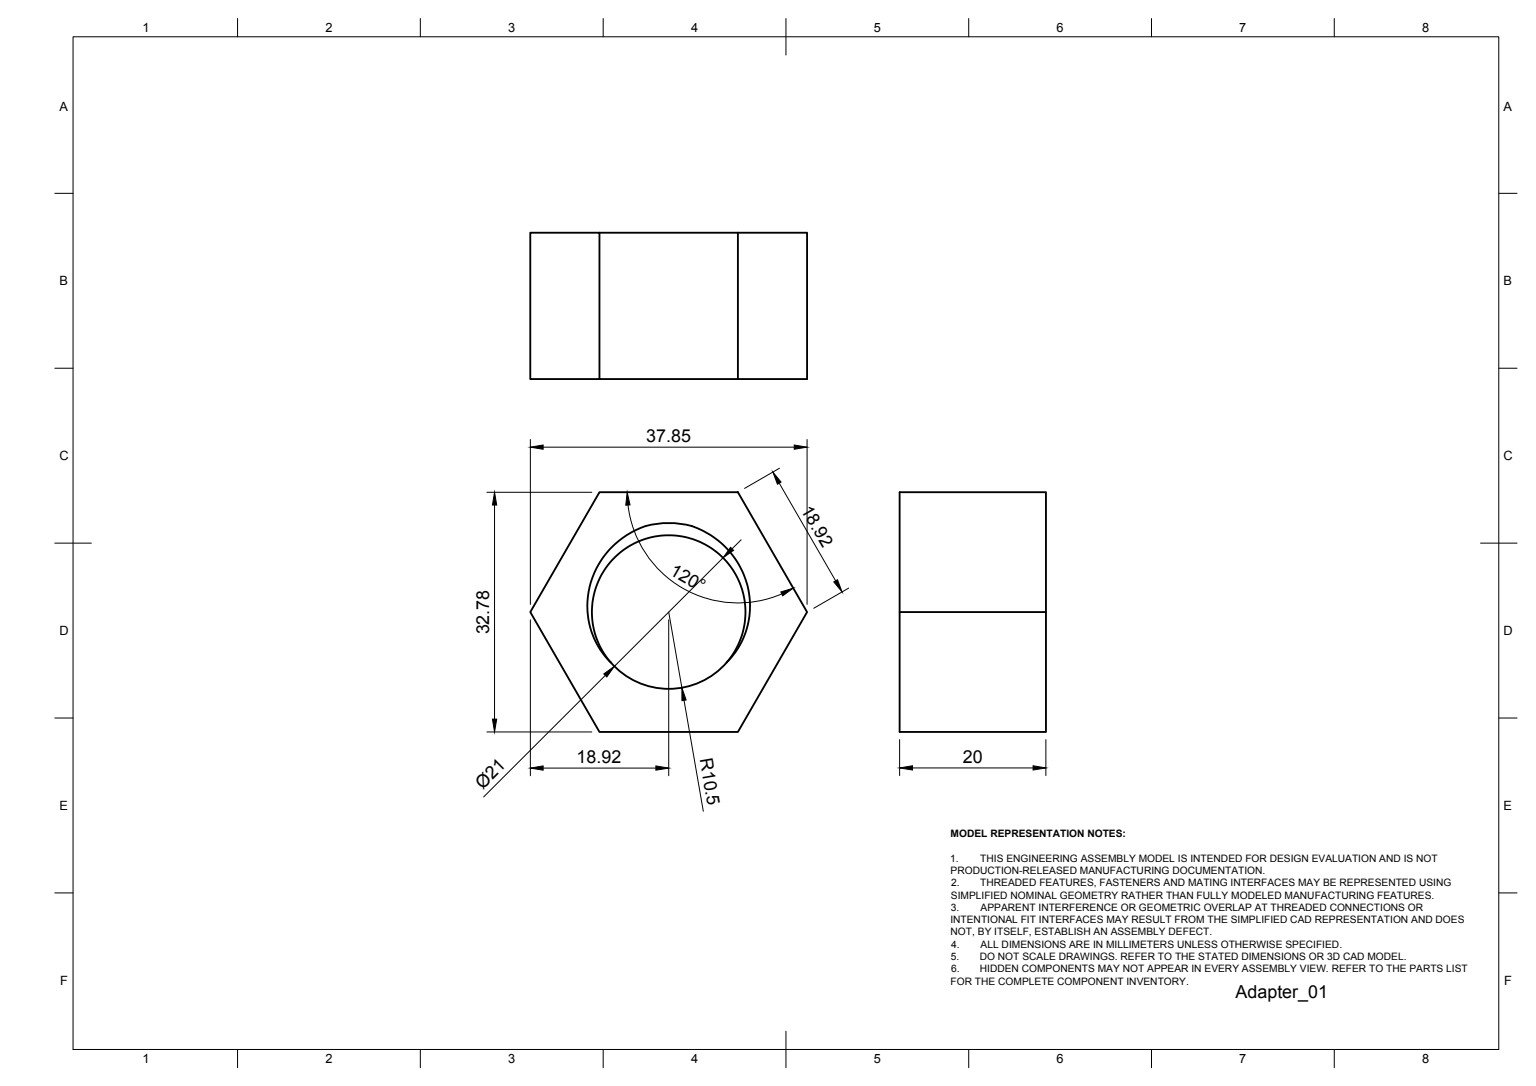
ISO-10303-21;
HEADER;
/* Generated by software containing ST-Developer
 * from STEP Tools, Inc. (www.steptools.com) 
 */

FILE_DESCRIPTION(
/* description */ (''),
/* implementation_level */ '2;1');

FILE_NAME(
/* name */ 'Adapter_01.step',
/* time_stamp */ '2026-10-06T12:47:13-07:00',
/* author */ (''),
/* organization */ (''),
/* preprocessor_version */ 'ST-DEVELOPER v20.2',
/* originating_system */ 'Autodesk Translation Framework v15.15.0.0',
/* authorisation */ '');

FILE_SCHEMA (('AUTOMOTIVE_DESIGN { 1 0 10303 214 3 1 1 }'));
ENDSEC;

DATA;
#10=MECHANICAL_DESIGN_GEOMETRIC_PRESENTATION_REPRESENTATION('',(#75),#42667);
#57=SHAPE_REPRESENTATION_RELATIONSHIP('SRR','None',#42710,#66);
#66=ADVANCED_BREP_SHAPE_REPRESENTATION('',(#84),#42666);
#75=STYLED_ITEM('',(#42756),#84);
#84=MANIFOLD_SOLID_BREP('Body1',#4040);
#92=B_SPLINE_SURFACE_WITH_KNOTS('',3,3,((#41391,#41392,#41393,#41394,#41395,
#41396,#41397,#41398,#41399,#41400,#41401,#41402,#41403,#41404,#41405,#41406,
#41407,#41408,#41409,#41410,#41411,#41412,#41413,#41414,#41415,#41416,#41417,
#41418,#41419,#41420,#41421,#41422,#41423,#41424,#41425,#41426,#41427,#41428,
#41429,#41430,#41431,#41432,#41433,#41434,#41435,#41436,#41437,#41438,#41439,
#41440,#41441,#41442,#41443,#41444,#41445,#41446,#41447,#41448,#41449,#41450,
#41451,#41452,#41453,#41454,#41455,#41456,#41457,#41458,#41459,#41460,#41461,
#41462,#41463,#41464,#41465,#41466,#41467,#41468,#41469,#41470,#41471,#41472,
#41473,#41474,#41475,#41476,#41477,#41478,#41479,#41480,#41481),(#41482,
#41483,#41484,#41485,#41486,#41487,#41488,#41489,#41490,#41491,#41492,#41493,
#41494,#41495,#41496,#41497,#41498,#41499,#41500,#41501,#41502,#41503,#41504,
#41505,#41506,#41507,#41508,#41509,#41510,#41511,#41512,#41513,#41514,#41515,
#41516,#41517,#41518,#41519,#41520,#41521,#41522,#41523,#41524,#41525,#41526,
#41527,#41528,#41529,#41530,#41531,#41532,#41533,#41534,#41535,#41536,#41537,
#41538,#41539,#41540,#41541,#41542,#41543,#41544,#41545,#41546,#41547,#41548,
#41549,#41550,#41551,#41552,#41553,#41554,#41555,#41556,#41557,#41558,#41559,
#41560,#41561,#41562,#41563,#41564,#41565,#41566,#41567,#41568,#41569,#41570,
#41571,#41572),(#41573,#41574,#41575,#41576,#41577,#41578,#41579,#41580,
#41581,#41582,#41583,#41584,#41585,#41586,#41587,#41588,#41589,#41590,#41591,
#41592,#41593,#41594,#41595,#41596,#41597,#41598,#41599,#41600,#41601,#41602,
#41603,#41604,#41605,#41606,#41607,#41608,#41609,#41610,#41611,#41612,#41613,
#41614,#41615,#41616,#41617,#41618,#41619,#41620,#41621,#41622,#41623,#41624,
#41625,#41626,#41627,#41628,#41629,#41630,#41631,#41632,#41633,#41634,#41635,
#41636,#41637,#41638,#41639,#41640,#41641,#41642,#41643,#41644,#41645,#41646,
#41647,#41648,#41649,#41650,#41651,#41652,#41653,#41654,#41655,#41656,#41657,
#41658,#41659,#41660,#41661,#41662,#41663),(#41664,#41665,#41666,#41667,
#41668,#41669,#41670,#41671,#41672,#41673,#41674,#41675,#41676,#41677,#41678,
#41679,#41680,#41681,#41682,#41683,#41684,#41685,#41686,#41687,#41688,#41689,
#41690,#41691,#41692,#41693,#41694,#41695,#41696,#41697,#41698,#41699,#41700,
#41701,#41702,#41703,#41704,#41705,#41706,#41707,#41708,#41709,#41710,#41711,
#41712,#41713,#41714,#41715,#41716,#41717,#41718,#41719,#41720,#41721,#41722,
#41723,#41724,#41725,#41726,#41727,#41728,#41729,#41730,#41731,#41732,#41733,
#41734,#41735,#41736,#41737,#41738,#41739,#41740,#41741,#41742,#41743,#41744,
#41745,#41746,#41747,#41748,#41749,#41750,#41751,#41752,#41753,#41754)),
 .UNSPECIFIED.,.F.,.F.,.F.,(4,4),(4,1,1,1,1,1,1,1,1,1,1,1,1,1,1,1,1,1,1,
1,1,1,1,1,1,1,1,1,1,1,1,1,1,1,1,1,1,1,1,1,1,1,1,1,1,1,1,1,1,1,1,1,1,1,1,
1,1,1,1,1,1,1,1,1,1,1,1,1,1,1,1,1,1,1,1,1,1,1,1,1,1,1,1,1,1,1,1,1,4),(-0.000129081019394558,
0.193330292353948),(11.8519068837255,12.3510302549558,12.8500245451668,
13.3490188353777,13.8480131255886,14.3470074157995,14.8460017060104,15.3449959962214,
15.8439902864323,16.3429845766432,16.8419788668541,17.3409731570651,17.839967447276,
18.3389617374869,18.8379560276978,19.3369503179088,19.8359446081197,20.3349388983306,
20.8339331885415,21.3329274787524,21.8319217689634,22.3309160591743,22.8299103493852,
23.3289046395961,23.8278989298071,24.326893220018,24.8258875102289,25.3248818004398,
25.8238760906508,26.3228703808617,26.8218646710726,27.3208589612835,27.8198532514944,
28.3188475417054,28.8178418319163,29.3168361221272,29.8158304123381,30.3148247025491,
30.81381899276,31.3128132829709,31.8118075731818,32.3108018633928,32.8097961536037,
33.3087904438146,33.8077847340255,34.3067790242364,34.8057733144474,35.3047676046583,
35.8037618948692,36.3027561850801,36.8017504752911,37.300744765502,37.7997390557129,
38.2987333459238,38.7977276361348,39.2967219263457,39.7957162165566,40.2947105067675,
40.7937047969784,41.2926990871894,41.7916933774003,42.2906876676112,42.7896819578221,
43.2886762480331,43.787670538244,44.2866648284549,44.7856591186658,45.2846534088767,
45.7836476990877,46.2826419892986,46.7816362795095,47.2806305697204,47.7796248599314,
48.2786191501423,48.7776134403532,49.2766077305641,49.7756020207751,50.274596310986,
50.7735906011969,51.2725848914078,51.7715791816187,52.2705734718297,52.7695677620406,
53.2685620522515,53.7675563424624,54.2665506326734,54.7655449228843,55.2645392130952,
55.7635335033061),.UNSPECIFIED.);
#93=B_SPLINE_SURFACE_WITH_KNOTS('',3,3,((#41996,#41997,#41998,#41999,#42000,
#42001,#42002,#42003,#42004,#42005,#42006,#42007,#42008,#42009,#42010,#42011,
#42012,#42013,#42014,#42015,#42016,#42017,#42018,#42019,#42020,#42021,#42022,
#42023,#42024,#42025,#42026,#42027,#42028,#42029,#42030,#42031,#42032,#42033,
#42034,#42035,#42036,#42037,#42038,#42039,#42040,#42041,#42042,#42043,#42044,
#42045,#42046,#42047,#42048,#42049,#42050,#42051,#42052,#42053,#42054,#42055,
#42056,#42057,#42058,#42059,#42060,#42061,#42062,#42063,#42064,#42065,#42066,
#42067,#42068,#42069,#42070,#42071,#42072,#42073,#42074,#42075,#42076,#42077,
#42078,#42079,#42080,#42081,#42082,#42083,#42084,#42085,#42086),(#42087,
#42088,#42089,#42090,#42091,#42092,#42093,#42094,#42095,#42096,#42097,#42098,
#42099,#42100,#42101,#42102,#42103,#42104,#42105,#42106,#42107,#42108,#42109,
#42110,#42111,#42112,#42113,#42114,#42115,#42116,#42117,#42118,#42119,#42120,
#42121,#42122,#42123,#42124,#42125,#42126,#42127,#42128,#42129,#42130,#42131,
#42132,#42133,#42134,#42135,#42136,#42137,#42138,#42139,#42140,#42141,#42142,
#42143,#42144,#42145,#42146,#42147,#42148,#42149,#42150,#42151,#42152,#42153,
#42154,#42155,#42156,#42157,#42158,#42159,#42160,#42161,#42162,#42163,#42164,
#42165,#42166,#42167,#42168,#42169,#42170,#42171,#42172,#42173,#42174,#42175,
#42176,#42177),(#42178,#42179,#42180,#42181,#42182,#42183,#42184,#42185,
#42186,#42187,#42188,#42189,#42190,#42191,#42192,#42193,#42194,#42195,#42196,
#42197,#42198,#42199,#42200,#42201,#42202,#42203,#42204,#42205,#42206,#42207,
#42208,#42209,#42210,#42211,#42212,#42213,#42214,#42215,#42216,#42217,#42218,
#42219,#42220,#42221,#42222,#42223,#42224,#42225,#42226,#42227,#42228,#42229,
#42230,#42231,#42232,#42233,#42234,#42235,#42236,#42237,#42238,#42239,#42240,
#42241,#42242,#42243,#42244,#42245,#42246,#42247,#42248,#42249,#42250,#42251,
#42252,#42253,#42254,#42255,#42256,#42257,#42258,#42259,#42260,#42261,#42262,
#42263,#42264,#42265,#42266,#42267,#42268),(#42269,#42270,#42271,#42272,
#42273,#42274,#42275,#42276,#42277,#42278,#42279,#42280,#42281,#42282,#42283,
#42284,#42285,#42286,#42287,#42288,#42289,#42290,#42291,#42292,#42293,#42294,
#42295,#42296,#42297,#42298,#42299,#42300,#42301,#42302,#42303,#42304,#42305,
#42306,#42307,#42308,#42309,#42310,#42311,#42312,#42313,#42314,#42315,#42316,
#42317,#42318,#42319,#42320,#42321,#42322,#42323,#42324,#42325,#42326,#42327,
#42328,#42329,#42330,#42331,#42332,#42333,#42334,#42335,#42336,#42337,#42338,
#42339,#42340,#42341,#42342,#42343,#42344,#42345,#42346,#42347,#42348,#42349,
#42350,#42351,#42352,#42353,#42354,#42355,#42356,#42357,#42358,#42359)),
 .UNSPECIFIED.,.F.,.F.,.F.,(4,4),(4,1,1,1,1,1,1,1,1,1,1,1,1,1,1,1,1,1,1,
1,1,1,1,1,1,1,1,1,1,1,1,1,1,1,1,1,1,1,1,1,1,1,1,1,1,1,1,1,1,1,1,1,1,1,1,
1,1,1,1,1,1,1,1,1,1,1,1,1,1,1,1,1,1,1,1,1,1,1,1,1,1,1,1,1,1,1,1,1,4),(-9.09719654654217E-5,
0.1933682374602),(14.3987024268659,14.8976967170768,15.3966910072877,15.8956852974986,
16.3946795877096,16.8936738779205,17.3926681681314,17.8916624583423,18.3906567485533,
18.8896510387642,19.3886453289751,19.887639619186,20.386633909397,20.8856281996079,
21.3846224898188,21.8836167800297,22.3826110702406,22.8816053604516,23.3805996506625,
23.8795939408734,24.3785882310843,24.8775825212953,25.3765768115062,25.8755711017171,
26.374565391928,26.8735596821389,27.3725539723499,27.8715482625608,28.3705425527717,
28.8695368429826,29.3685311331936,29.8675254234045,30.3665197136154,30.8655140038263,
31.3645082940373,31.8635025842482,32.3624968744591,32.86149116467,33.3604854548809,
33.8594797450919,34.3584740353028,34.8574683255137,35.3564626157246,35.8554569059356,
36.3544511961465,36.8534454863574,37.3524397765683,37.8514340667792,38.3504283569902,
38.8494226472011,39.348416937412,39.8474112276229,40.3464055178339,40.8453998080448,
41.3443940982557,41.8433883884666,42.3423826786776,42.8413769688885,43.3403712590994,
43.8393655493103,44.3383598395212,44.8373541297322,45.3363484199431,45.835342710154,
46.3343370003649,46.8333312905759,47.3323255807868,47.8313198709977,48.3303141612086,
48.8293084514195,49.3283027416305,49.8272970318414,50.3262913220523,50.8252856122632,
51.3242799024742,51.8232741926851,52.322268482896,52.8212627731069,53.3202570633179,
53.8192513535288,54.3182456437397,54.8172399339506,55.3162342241615,55.8152285143725,
56.3142228045834,56.8132170947943,57.3122113850052,57.8112056752162,58.3103290677895),
 .UNSPECIFIED.);
#324=B_SPLINE_CURVE_WITH_KNOTS('',3,(#36923,#36924,#36925,#36926),
 .UNSPECIFIED.,.F.,.F.,(4,4),(55.632514020542,55.7635335033061),
 .UNSPECIFIED.);
#325=B_SPLINE_CURVE_WITH_KNOTS('',3,(#36929,#36930,#36931,#36932,#36933),
 .UNSPECIFIED.,.F.,.F.,(4,1,4),(55.6324918109698,55.8152285143725,56.2866044747298),
 .UNSPECIFIED.);
#326=B_SPLINE_CURVE_WITH_KNOTS('',3,(#36939,#36940,#36941,#36942,#36943,
#36944,#36945,#36946,#36947,#36948,#36949,#36950,#36951,#36952,#36953,#36954,
#36955,#36956,#36957,#36958,#36959,#36960,#36961,#36962,#36963,#36964,#36965,
#36966,#36967,#36968,#36969,#36970,#36971,#36972,#36973,#36974,#36975,#36976,
#36977,#36978,#36979,#36980,#36981,#36982,#36983,#36984,#36985,#36986,#36987,
#36988,#36989,#36990,#36991,#36992,#36993,#36994,#36995,#36996,#36997,#36998,
#36999,#37000,#37001,#37002,#37003,#37004,#37005,#37006,#37007,#37008,#37009,
#37010,#37011,#37012,#37013,#37014,#37015,#37016,#37017,#37018,#37019,#37020,
#37021,#37022,#37023,#37024,#37025,#37026,#37027,#37028,#37029,#37030,#37031,
#37032,#37033,#37034,#37035,#37036,#37037,#37038,#37039,#37040,#37041,#37042,
#37043,#37044,#37045,#37046,#37047,#37048,#37049,#37050,#37051,#37052,#37053,
#37054,#37055,#37056,#37057,#37058,#37059,#37060,#37061,#37062,#37063,#37064,
#37065,#37066,#37067,#37068,#37069,#37070,#37071,#37072,#37073,#37074,#37075,
#37076,#37077,#37078,#37079,#37080,#37081,#37082,#37083,#37084,#37085,#37086,
#37087,#37088,#37089,#37090,#37091,#37092,#37093,#37094,#37095,#37096,#37097,
#37098,#37099,#37100,#37101,#37102,#37103,#37104,#37105,#37106,#37107,#37108,
#37109,#37110),.UNSPECIFIED.,.F.,.F.,(4,3,3,3,3,3,3,3,3,3,3,3,3,3,3,3,3,
3,3,3,3,3,3,3,3,3,3,3,3,3,3,3,3,3,3,3,3,3,3,3,3,3,3,3,3,3,3,3,3,3,3,3,3,
3,3,3,3,4),(49.3493405936366,49.4193689479141,49.4893896861999,49.5609427698437,
49.6309674799891,49.7032847503821,49.7756020207751,49.8456426343618,49.9156713518887,
49.9856922954051,50.0579182993003,50.1279429852639,50.201269648125,50.274596310986,
50.3446366811021,50.4146651537395,50.4846858515977,50.5569120389975,50.6269364804616,
50.7002635408293,50.7735906011969,50.8436318783237,50.9136612616073,50.9836828713458,
51.0559083763613,51.1259337214531,51.1992593064304,51.2725848914078,51.3426239524563,
51.4126511125654,51.4826704978761,51.5548976688117,51.6249208138906,51.6982499977546,
51.7715791816187,51.8416224003585,51.9116537285312,51.9816772813509,52.0539013289706,
52.1239285887193,52.1972510302745,52.2705734718297,52.3406109642765,52.4106365581925,
52.4806543837547,52.5528827283262,52.6229043486391,52.6962360553399,52.7695677620406,
52.8396086885631,52.9096377028379,52.9796589263131,53.0518847077977,53.1219096292928,
53.1952358407721,53.2685620522515,53.3417764954199,53.4070751084796),
 .UNSPECIFIED.);
#327=B_SPLINE_CURVE_WITH_KNOTS('',3,(#37111,#37112,#37113,#37114,#37115,
#37116,#37117,#37118),.UNSPECIFIED.,.F.,.F.,(4,1,1,1,1,4),(53.4070751110265,
53.7675563424624,54.2665506326734,54.7655449228843,55.2645392130952,55.632514020542),
 .UNSPECIFIED.);
#328=B_SPLINE_CURVE_WITH_KNOTS('',3,(#37120,#37121,#37122,#37123,#37124,
#37125,#37126,#37127),.UNSPECIFIED.,.F.,.F.,(4,1,1,1,1,4),(53.4070751344278,
53.8192513535288,54.3182456437397,54.8172399339506,55.3162342241615,55.6324918109698),
 .UNSPECIFIED.);
#329=B_SPLINE_CURVE_WITH_KNOTS('',3,(#37128,#37129,#37130,#37131,#37132,
#37133,#37134,#37135,#37136,#37137,#37138,#37139,#37140,#37141,#37142,#37143,
#37144,#37145,#37146,#37147,#37148,#37149,#37150,#37151,#37152,#37153,#37154,
#37155,#37156,#37157,#37158,#37159,#37160,#37161,#37162,#37163,#37164,#37165,
#37166,#37167,#37168,#37169,#37170,#37171,#37172,#37173,#37174,#37175,#37176,
#37177,#37178,#37179,#37180,#37181,#37182,#37183,#37184,#37185,#37186,#37187,
#37188,#37189,#37190,#37191,#37192,#37193,#37194,#37195,#37196,#37197,#37198,
#37199,#37200,#37201,#37202,#37203,#37204,#37205,#37206,#37207,#37208,#37209,
#37210,#37211,#37212,#37213,#37214,#37215,#37216,#37217,#37218,#37219,#37220,
#37221,#37222,#37223,#37224,#37225,#37226,#37227,#37228,#37229,#37230,#37231,
#37232,#37233,#37234,#37235,#37236,#37237,#37238,#37239,#37240,#37241,#37242,
#37243,#37244,#37245,#37246,#37247,#37248,#37249,#37250,#37251,#37252,#37253,
#37254,#37255,#37256,#37257,#37258,#37259,#37260,#37261,#37262,#37263,#37264,
#37265,#37266,#37267,#37268,#37269,#37270,#37271,#37272,#37273,#37274,#37275,
#37276,#37277,#37278,#37279,#37280,#37281,#37282,#37283,#37284,#37285,#37286,
#37287,#37288,#37289,#37290,#37291,#37292,#37293,#37294,#37295,#37296,#37297,
#37298,#37299,#37300,#37301,#37302),.UNSPECIFIED.,.F.,.F.,(4,3,3,3,3,3,
3,3,3,3,3,3,3,3,3,3,3,3,3,3,3,3,3,3,3,3,3,3,3,3,3,3,3,3,3,3,3,3,3,3,3,3,
3,3,3,3,3,3,3,3,3,3,3,3,3,3,3,3,4),(49.3493315211037,49.4193681064343,49.4893940333262,
49.5594134227735,49.6294388812757,49.6994638047524,49.7695045346538,49.8272970318414,
49.8973376266719,49.9673663251347,50.0373872493319,50.109613267512,50.1796379337725,
50.2529646279124,50.3262913220523,50.3963319018199,50.4663605851638,50.5363814942255,
50.6086075237349,50.678632175007,50.7519588936351,50.8252856122632,50.8953262259418,
50.9653549432983,51.0353758863851,51.1076018904074,51.1776265753145,51.2509532388943,
51.3242799024742,51.3943204573068,51.4643491156853,51.5343699998164,51.6065960480335,
51.6766206747678,51.7499474337265,51.8232741926851,51.8933148183004,51.963343547517,
52.0333645023575,52.1055904974922,52.1756151937477,52.2489418383219,52.322268482896,
52.3923090961645,52.4623378133711,52.5323587565658,52.6045847607011,52.674609446344,
52.7479361097254,52.8212627731069,52.8913031445529,52.961331618526,53.0313523177225,
53.1035785041213,53.1736029469128,53.2469300051154,53.3202570633179,53.3951479415614,
53.4070751110265),.UNSPECIFIED.);
#330=B_SPLINE_CURVE_WITH_KNOTS('',3,(#37308,#37309,#37310,#37311,#37312,
#37313,#37314,#37315,#37316,#37317,#37318,#37319,#37320,#37321,#37322,#37323,
#37324,#37325,#37326,#37327,#37328,#37329,#37330,#37331,#37332,#37333,#37334,
#37335,#37336,#37337,#37338,#37339,#37340,#37341,#37342,#37343,#37344,#37345,
#37346,#37347,#37348,#37349,#37350,#37351,#37352,#37353,#37354,#37355,#37356,
#37357,#37358,#37359,#37360,#37361,#37362,#37363,#37364,#37365,#37366,#37367,
#37368,#37369,#37370,#37371,#37372,#37373,#37374,#37375,#37376,#37377,#37378,
#37379,#37380,#37381,#37382,#37383,#37384,#37385,#37386,#37387,#37388,#37389,
#37390,#37391,#37392,#37393,#37394,#37395,#37396,#37397,#37398,#37399,#37400,
#37401,#37402,#37403,#37404,#37405,#37406,#37407,#37408,#37409,#37410,#37411,
#37412,#37413,#37414,#37415,#37416,#37417,#37418,#37419,#37420,#37421,#37422,
#37423,#37424,#37425,#37426,#37427,#37428,#37429,#37430,#37431,#37432,#37433,
#37434,#37435,#37436,#37437,#37438,#37439,#37440,#37441,#37442,#37443,#37444,
#37445,#37446,#37447,#37448,#37449,#37450,#37451,#37452,#37453,#37454,#37455,
#37456,#37457,#37458,#37459,#37460,#37461,#37462,#37463,#37464,#37465,#37466,
#37467,#37468,#37469,#37470,#37471,#37472,#37473,#37474,#37475,#37476,#37477,
#37478,#37479,#37480,#37481,#37482),.UNSPECIFIED.,.F.,.F.,(4,3,3,3,3,3,
3,3,3,3,3,3,3,3,3,3,3,3,3,3,3,3,3,3,3,3,3,3,3,3,3,3,3,3,3,3,3,3,3,3,3,3,
3,3,3,3,3,3,3,3,3,3,3,3,3,3,3,3,4),(43.0661349437165,43.1361595852945,43.2061863657319,
43.2762263384948,43.2886762480331,43.3587168388614,43.4287455333042,43.4987664534742,
43.5709924746666,43.6410171369318,43.7143438375879,43.787670538244,43.8577111290883,
43.9277398235473,43.9977607437335,44.0699867649139,44.1400114271953,44.2133381278251,
44.2866648284549,44.356705419211,44.426734113581,44.4967550336782,44.5689810549251,
44.6390057171185,44.7123324178922,44.7856591186658,44.8556997096685,44.9257284042863,
44.9957493246315,45.0679753456928,45.1380000081315,45.2113267085041,45.2846534088767,
45.3546939993659,45.4247226934689,45.4947436132985,45.5669696347458,45.6369942966754,
45.7103209978815,45.7836476990877,45.8536882903938,45.9237169853148,45.9937379059628,
46.0659639267968,46.1359885895326,46.2093152894156,46.2826419892986,46.3526825797948,
46.4227112739064,46.4927321937468,46.5649582151875,46.6349828771319,46.7083095783207,
46.7816362795095,46.8516132827516,46.9215804164053,46.9915381364908,47.0614983061719,
47.1238898038469),.UNSPECIFIED.);
#331=B_SPLINE_CURVE_WITH_KNOTS('',3,(#37483,#37484,#37485,#37486,#37487,
#37488,#37489,#37490,#37491,#37492,#37493,#37494,#37495,#37496,#37497,#37498,
#37499,#37500,#37501,#37502,#37503,#37504,#37505,#37506,#37507,#37508,#37509,
#37510,#37511,#37512,#37513,#37514,#37515,#37516,#37517,#37518,#37519,#37520,
#37521,#37522,#37523,#37524,#37525,#37526,#37527,#37528,#37529,#37530,#37531,
#37532,#37533,#37534,#37535,#37536,#37537,#37538,#37539,#37540,#37541,#37542,
#37543,#37544,#37545,#37546,#37547,#37548,#37549,#37550,#37551,#37552,#37553,
#37554,#37555,#37556,#37557,#37558,#37559,#37560,#37561,#37562,#37563,#37564,
#37565,#37566,#37567,#37568,#37569,#37570,#37571,#37572,#37573,#37574,#37575,
#37576,#37577,#37578,#37579),.UNSPECIFIED.,.F.,.F.,(4,3,3,3,3,3,3,3,3,3,
3,3,3,3,3,3,3,3,3,3,3,3,3,3,3,3,3,3,3,3,3,3,4),(47.1238898039153,47.1966069931218,
47.269346291875,47.2806305697204,47.3506711645816,47.4206998630754,47.4907207873035,
47.5629468054605,47.6329714717519,47.7062981658417,47.7796248599314,47.8496654396268,
47.919694122898,47.9897150318869,48.0619410614508,48.1319657126511,48.2052924313967,
48.2786191501423,48.3486597639494,48.4186884814349,48.4887094246505,48.5609354285762,
48.6309601136108,48.704286776982,48.7776134403532,48.8476539950211,48.9176826532346,
48.987703537201,49.0599295855418,49.1299542121136,49.2032809713389,49.2766077305641,
49.3493405936366),.UNSPECIFIED.);
#332=B_SPLINE_CURVE_WITH_KNOTS('',3,(#37581,#37582,#37583,#37584,#37585,
#37586,#37587,#37588,#37589,#37590,#37591,#37592,#37593,#37594,#37595,#37596,
#37597,#37598,#37599,#37600,#37601,#37602,#37603,#37604,#37605,#37606,#37607,
#37608,#37609,#37610,#37611,#37612,#37613,#37614,#37615,#37616,#37617,#37618,
#37619,#37620,#37621,#37622,#37623,#37624,#37625,#37626,#37627,#37628,#37629,
#37630,#37631,#37632,#37633,#37634,#37635,#37636,#37637,#37638,#37639,#37640,
#37641,#37642,#37643,#37644,#37645,#37646,#37647,#37648,#37649,#37650,#37651,
#37652,#37653,#37654,#37655,#37656,#37657,#37658,#37659,#37660,#37661,#37662,
#37663,#37664,#37665,#37666,#37667,#37668,#37669,#37670,#37671,#37672,#37673,
#37674,#37675,#37676,#37677),.UNSPECIFIED.,.F.,.F.,(4,3,3,3,3,3,3,3,3,3,
3,3,3,3,3,3,3,3,3,3,3,3,3,3,3,3,3,3,3,3,3,3,4),(47.1238898039108,47.1954657532806,
47.2670653523193,47.3323255807868,47.4023661717881,47.4723948664045,47.5424157867478,
47.6146418078103,47.6846664702475,47.7579931706226,47.8313198709977,47.9013604614893,
47.9713891555945,48.0414100754268,48.1136360968722,48.1836607588042,48.2569874600064,
48.3303141612086,48.4003547525115,48.4703834474297,48.5404043680745,48.6126303889108,
48.6826550516439,48.7559817515317,48.8293084514195,48.8993490419166,48.9693777360291,
49.0393986558705,49.1116246773105,49.1816493392556,49.2549760404431,49.3283027416305,
49.3493315211037),.UNSPECIFIED.);
#333=B_SPLINE_CURVE_WITH_KNOTS('',3,(#37678,#37679,#37680,#37681,#37682,
#37683,#37684,#37685,#37686,#37687,#37688,#37689,#37690,#37691,#37692,#37693,
#37694,#37695,#37696,#37697,#37698,#37699,#37700,#37701,#37702,#37703,#37704,
#37705,#37706,#37707,#37708,#37709,#37710,#37711,#37712,#37713,#37714,#37715,
#37716,#37717,#37718,#37719,#37720,#37721,#37722,#37723,#37724,#37725,#37726,
#37727,#37728,#37729,#37730,#37731,#37732,#37733,#37734,#37735,#37736,#37737,
#37738,#37739,#37740,#37741,#37742,#37743,#37744,#37745,#37746,#37747,#37748,
#37749,#37750,#37751,#37752,#37753,#37754,#37755,#37756,#37757,#37758,#37759,
#37760,#37761,#37762,#37763,#37764,#37765,#37766,#37767,#37768,#37769,#37770,
#37771,#37772,#37773,#37774,#37775,#37776,#37777,#37778,#37779,#37780,#37781,
#37782,#37783,#37784,#37785,#37786,#37787,#37788,#37789,#37790,#37791,#37792,
#37793,#37794,#37795,#37796,#37797,#37798,#37799,#37800,#37801,#37802,#37803,
#37804,#37805,#37806,#37807,#37808,#37809,#37810,#37811,#37812,#37813,#37814,
#37815,#37816,#37817,#37818,#37819,#37820,#37821,#37822,#37823,#37824,#37825,
#37826,#37827,#37828,#37829,#37830,#37831,#37832,#37833,#37834,#37835,#37836,
#37837,#37838,#37839,#37840,#37841,#37842,#37843,#37844,#37845,#37846,#37847,
#37848,#37849),.UNSPECIFIED.,.F.,.F.,(4,3,3,3,3,3,3,3,3,3,3,3,3,3,3,3,3,
3,3,3,3,3,3,3,3,3,3,3,3,3,3,3,3,3,3,3,3,3,3,3,3,3,3,3,3,3,3,3,3,3,3,3,3,
3,3,3,3,4),(43.0661440137509,43.1361697254765,43.2061945280937,43.2762355868376,
43.3403712590994,43.4104118499255,43.4804405443662,43.550461464534,43.6226874857281,
43.6927121479913,43.7660388486508,43.8393655493103,43.909406140138,43.9794348345803,
44.0494557547496,44.1216817759425,44.1917064382073,44.2650331388643,44.3383598395212,
44.408400430345,44.4784291247834,44.5484500449487,44.6206760661446,44.6907007284056,
44.7640274290689,44.8373541297322,44.9073947205635,44.9774234150094,45.0474443351824,
45.1196703563726,45.1896950186409,45.263021719292,45.3363484199431,45.4063890107635,
45.4764177051986,45.5464386253606,45.618664646559,45.6886893088167,45.7620160094854,
45.835342710154,45.9053833009824,45.9754119954253,46.0454329155953,46.1176589367877,
46.187683599053,46.2610102997089,46.3343370003649,46.4043775912091,46.4744062856679,
46.544427205854,46.6166532270345,46.6866778893158,46.7600045899459,46.8333312905759,
46.9059709188937,46.9763616597276,47.0501257317873,47.1238898038469),
 .UNSPECIFIED.);
#334=B_SPLINE_CURVE_WITH_KNOTS('',3,(#37855,#37856,#37857,#37858,#37859,
#37860,#37861,#37862,#37863,#37864,#37865,#37866,#37867),.UNSPECIFIED.,
 .F.,.F.,(4,1,1,1,1,1,1,1,1,1,4),(36.7829477512195,36.8017504752911,37.300744765502,
37.7997390557129,38.2987333459238,38.7977276361348,39.2967219263457,39.7957162165566,
40.2947105067675,40.7937047969784,40.8407044966673),.UNSPECIFIED.);
#335=B_SPLINE_CURVE_WITH_KNOTS('',3,(#37868,#37869,#37870,#37871,#37872,
#37873,#37874,#37875,#37876,#37877,#37878,#37879,#37880,#37881,#37882,#37883,
#37884,#37885,#37886,#37887,#37888,#37889,#37890,#37891,#37892,#37893,#37894,
#37895,#37896,#37897,#37898,#37899,#37900,#37901,#37902,#37903,#37904,#37905,
#37906,#37907,#37908,#37909,#37910,#37911,#37912,#37913,#37914,#37915,#37916,
#37917,#37918,#37919,#37920,#37921,#37922,#37923,#37924,#37925,#37926,#37927,
#37928,#37929,#37930,#37931,#37932,#37933,#37934,#37935,#37936,#37937,#37938,
#37939,#37940,#37941,#37942,#37943,#37944,#37945,#37946,#37947,#37948,#37949,
#37950,#37951,#37952,#37953,#37954,#37955,#37956,#37957,#37958,#37959,#37960,
#37961,#37962,#37963,#37964),.UNSPECIFIED.,.F.,.F.,(4,3,3,3,3,3,3,3,3,3,
3,3,3,3,3,3,3,3,3,3,3,3,3,3,3,3,3,3,3,3,3,3,4),(40.8407044966673,40.910513107026,
40.9803103162599,41.050100831576,41.1198969722149,41.1896937756429,41.2595054868552,
41.2926990871894,41.3627396780171,41.4327683724595,41.5027892926283,41.5750153138213,
41.645039976086,41.7183666767432,41.7916933774003,41.861733968224,41.9317626626622,
42.0017835828273,42.0740096040233,42.1440342662842,42.2173609669477,42.2906876676112,
42.3607282584425,42.4307569528884,42.500777873061,42.5730038942513,42.6430285565196,
42.7163552571708,42.7896819578221,42.859723254519,42.9297517388031,42.9997772294764,
43.0661349437165),.UNSPECIFIED.);
#336=B_SPLINE_CURVE_WITH_KNOTS('',3,(#37966,#37967,#37968,#37969,#37970,
#37971,#37972,#37973,#37974,#37975,#37976,#37977,#37978,#37979,#37980,#37981,
#37982,#37983,#37984,#37985,#37986,#37987,#37988,#37989,#37990,#37991,#37992,
#37993,#37994,#37995,#37996,#37997,#37998,#37999,#38000,#38001,#38002,#38003,
#38004,#38005,#38006,#38007,#38008,#38009,#38010,#38011,#38012,#38013,#38014,
#38015,#38016,#38017,#38018,#38019,#38020,#38021,#38022,#38023,#38024,#38025,
#38026,#38027,#38028,#38029,#38030,#38031,#38032,#38033,#38034,#38035,#38036,
#38037,#38038,#38039,#38040,#38041,#38042,#38043,#38044,#38045,#38046,#38047,
#38048,#38049,#38050,#38051,#38052,#38053,#38054,#38055,#38056,#38057,#38058,
#38059,#38060,#38061,#38062,#38063,#38064,#38065),.UNSPECIFIED.,.F.,.F.,
(4,3,3,3,3,3,3,3,3,3,3,3,3,3,3,3,3,3,3,3,3,3,3,3,3,3,3,3,3,3,3,3,3,4),(40.8407044966673,
40.8453998080448,40.9154403988712,40.9854690933122,41.0554900134805,41.1277160346743,
41.1977406969378,41.2710673975968,41.3443940982557,41.4144346890823,41.4844633835235,
41.5544843036917,41.6267103248854,41.6967349871492,41.7700616878079,41.8433883884666,
41.913428979293,41.9834576737341,42.0534785939022,42.1257046150961,42.1957292773597,
42.2690559780186,42.3423826786776,42.4124232695042,42.4824519639455,42.5524728841137,
42.6246989053074,42.6947235675711,42.7680502682298,42.8413769688885,42.9114171285507,
42.981444789593,43.051465392962,43.0661440137509),.UNSPECIFIED.);
#337=B_SPLINE_CURVE_WITH_KNOTS('',3,(#38066,#38067,#38068,#38069,#38070,
#38071,#38072,#38073,#38074,#38075,#38076,#38077,#38078,#38079,#38080,#38081,
#38082,#38083,#38084,#38085,#38086,#38087,#38088,#38089,#38090,#38091,#38092,
#38093,#38094,#38095,#38096,#38097,#38098,#38099,#38100,#38101,#38102,#38103,
#38104,#38105,#38106,#38107,#38108,#38109,#38110,#38111,#38112,#38113,#38114,
#38115,#38116,#38117,#38118,#38119,#38120,#38121,#38122,#38123,#38124,#38125,
#38126,#38127,#38128,#38129,#38130,#38131,#38132,#38133,#38134,#38135,#38136,
#38137,#38138,#38139,#38140,#38141,#38142,#38143,#38144,#38145,#38146,#38147,
#38148,#38149,#38150,#38151,#38152,#38153,#38154,#38155,#38156,#38157,#38158,
#38159,#38160,#38161,#38162,#38163,#38164,#38165,#38166,#38167,#38168,#38169,
#38170,#38171,#38172,#38173,#38174,#38175,#38176,#38177,#38178,#38179,#38180,
#38181,#38182,#38183,#38184,#38185,#38186,#38187,#38188,#38189,#38190,#38191,
#38192,#38193,#38194,#38195,#38196,#38197,#38198,#38199,#38200,#38201,#38202,
#38203,#38204,#38205,#38206,#38207,#38208,#38209,#38210,#38211,#38212,#38213,
#38214,#38215,#38216,#38217,#38218,#38219,#38220,#38221,#38222,#38223,#38224,
#38225,#38226,#38227,#38228,#38229,#38230,#38231,#38232,#38233,#38234,#38235,
#38236,#38237),.UNSPECIFIED.,.F.,.F.,(4,3,3,3,3,3,3,3,3,3,3,3,3,3,3,3,3,
3,3,3,3,3,3,3,3,3,3,3,3,3,3,3,3,3,3,3,3,3,3,3,3,3,3,3,3,3,3,3,3,3,3,3,3,
3,3,3,3,4),(36.7829389522053,36.8534454863574,36.9234860771838,36.993514771625,
37.0635356917935,37.1357617129872,37.2057863752507,37.2791130759095,37.3524397765683,
37.4224803673948,37.4925090618357,37.5625299820039,37.6347560031977,37.7047806654614,
37.7781073661203,37.8514340667792,37.9214746576057,37.9915033520468,38.0615242722151,
38.1337502934089,38.2037749556726,38.2771016563314,38.3504283569902,38.4204689478168,
38.4904976422578,38.5605185624258,38.6327445836196,38.7027692458831,38.7760959465421,
38.8494226472011,38.9194632380276,38.9894919324685,39.0595128526359,39.1317388738299,
39.2017635360937,39.2750902367529,39.348416937412,39.4184575282385,39.4884862226793,
39.5585071428479,39.6307331640416,39.7007578263054,39.7740845269641,39.8474112276229,
39.9174518184494,39.9874805128906,40.0575014330589,40.1297274542526,40.1997521165164,
40.2730788171751,40.3464055178339,40.4164150422325,40.4864125754172,40.5564023218123,
40.6274778655123,40.6974714282655,40.7690879624389,40.8407044966123),
 .UNSPECIFIED.);
#338=B_SPLINE_CURVE_WITH_KNOTS('',3,(#38243,#38244,#38245,#38246,#38247,
#38248,#38249,#38250,#38251,#38252,#38253,#38254,#38255,#38256,#38257,#38258,
#38259,#38260,#38261,#38262,#38263,#38264,#38265,#38266,#38267,#38268,#38269,
#38270,#38271,#38272,#38273,#38274,#38275,#38276,#38277,#38278,#38279,#38280,
#38281,#38282,#38283,#38284,#38285,#38286,#38287,#38288,#38289,#38290,#38291,
#38292,#38293,#38294,#38295,#38296,#38297,#38298,#38299,#38300,#38301,#38302,
#38303,#38304,#38305,#38306,#38307,#38308,#38309,#38310,#38311,#38312,#38313,
#38314,#38315,#38316,#38317,#38318,#38319,#38320,#38321,#38322,#38323,#38324,
#38325,#38326,#38327,#38328,#38329,#38330,#38331,#38332,#38333,#38334,#38335,
#38336,#38337,#38338,#38339,#38340,#38341,#38342,#38343,#38344,#38345,#38346,
#38347,#38348,#38349,#38350,#38351,#38352,#38353,#38354,#38355,#38356,#38357,
#38358,#38359,#38360,#38361,#38362,#38363,#38364,#38365,#38366,#38367,#38368,
#38369,#38370,#38371,#38372,#38373,#38374,#38375,#38376,#38377,#38378,#38379,
#38380,#38381,#38382,#38383,#38384,#38385,#38386,#38387,#38388,#38389,#38390,
#38391,#38392,#38393,#38394,#38395,#38396,#38397,#38398,#38399,#38400,#38401,
#38402,#38403,#38404,#38405,#38406,#38407,#38408,#38409,#38410,#38411,#38412,
#38413,#38414,#38415,#38416,#38417),.UNSPECIFIED.,.F.,.F.,(4,3,3,3,3,3,
3,3,3,3,3,3,3,3,3,3,3,3,3,3,3,3,3,3,3,3,3,3,3,3,3,3,3,3,3,3,3,3,3,3,3,3,
3,3,3,3,3,3,3,3,3,3,3,3,3,3,3,3,4),(30.4997797388357,30.5697978420759,30.6398226552016,
30.7098483404733,30.7798883251637,30.81381899276,30.8838595835864,30.9538882780275,
31.0239091981955,31.0961352193893,31.166159881653,31.2394865823119,31.3128132829709,
31.3828538737974,31.4528825682385,31.5229034884066,31.5951295096004,31.6651541718641,
31.7384808725229,31.8118075731818,31.8818481640083,31.9518768584493,32.0218977786175,
32.0941237998113,32.164148462075,32.2374751627339,32.3108018633928,32.3808424542193,
32.4508711486604,32.5208920688285,32.5931180900223,32.6631427522861,32.7364694529449,
32.8097961536037,32.8798367444301,32.9498654388712,33.0198863590392,33.0921123802331,
33.1621370424967,33.2354637431556,33.3087904438146,33.378831034641,33.4488597290821,
33.5188806492501,33.5911066704439,33.6611313327075,33.7344580333665,33.8077847340255,
33.877825324852,33.9478540192931,34.0178749394612,34.090100960655,34.1601256229187,
34.2334523235775,34.3067790242364,34.3776775785114,34.4485623759747,34.5194352520091,
34.5575191894138),.UNSPECIFIED.);
#339=B_SPLINE_CURVE_WITH_KNOTS('',3,(#38418,#38419,#38420,#38421,#38422,
#38423,#38424,#38425),.UNSPECIFIED.,.F.,.F.,(4,1,1,1,1,4),(34.5575191894877,
34.8057733144474,35.3047676046583,35.8037618948692,36.3027561850801,36.7829477512195),
 .UNSPECIFIED.);
#340=B_SPLINE_CURVE_WITH_KNOTS('',3,(#38427,#38428,#38429,#38430,#38431,
#38432,#38433,#38434,#38435,#38436,#38437,#38438,#38439,#38440,#38441,#38442,
#38443,#38444,#38445,#38446,#38447,#38448,#38449,#38450,#38451,#38452,#38453,
#38454,#38455,#38456,#38457,#38458,#38459,#38460,#38461,#38462,#38463,#38464,
#38465,#38466,#38467,#38468,#38469,#38470,#38471,#38472,#38473,#38474,#38475,
#38476,#38477,#38478,#38479,#38480,#38481,#38482,#38483,#38484,#38485,#38486,
#38487,#38488,#38489,#38490,#38491,#38492,#38493,#38494,#38495,#38496,#38497,
#38498,#38499,#38500,#38501,#38502,#38503,#38504,#38505,#38506,#38507,#38508,
#38509,#38510,#38511,#38512,#38513,#38514,#38515,#38516,#38517,#38518,#38519,
#38520,#38521,#38522,#38523),.UNSPECIFIED.,.F.,.F.,(4,3,3,3,3,3,3,3,3,3,
3,3,3,3,3,3,3,3,3,3,3,3,3,3,3,3,3,3,3,3,3,3,4),(34.5575191894877,34.6277996055737,
34.6980904637057,34.7683845128919,34.8386929125139,34.8574683255137,34.9275089163402,
34.9975376107813,35.0675585309494,35.1397845521432,35.2098092144068,35.2831359150657,
35.3564626157246,35.4265032065511,35.4965319009923,35.5665528211606,35.6387788423543,
35.7088035046181,35.7821302052769,35.8554569059356,35.9254974967621,35.9955261912031,
36.0655471113711,36.1377731325649,36.2077977948286,36.2811244954875,36.3544511961465,
36.4244912351492,36.4945191737348,36.5666241183524,36.6366450905632,36.7097920213842,
36.7829389522053),.UNSPECIFIED.);
#341=B_SPLINE_CURVE_WITH_KNOTS('',3,(#38524,#38525,#38526,#38527,#38528,
#38529,#38530,#38531,#38532,#38533,#38534,#38535,#38536,#38537,#38538,#38539,
#38540,#38541,#38542,#38543,#38544,#38545,#38546,#38547,#38548,#38549,#38550,
#38551,#38552,#38553,#38554,#38555,#38556,#38557,#38558,#38559,#38560,#38561,
#38562,#38563,#38564,#38565,#38566,#38567,#38568,#38569,#38570,#38571,#38572,
#38573,#38574,#38575,#38576,#38577,#38578,#38579,#38580,#38581,#38582,#38583,
#38584,#38585,#38586,#38587,#38588,#38589,#38590,#38591,#38592,#38593,#38594,
#38595,#38596,#38597,#38598,#38599,#38600,#38601,#38602,#38603,#38604,#38605,
#38606,#38607,#38608,#38609,#38610,#38611,#38612,#38613,#38614,#38615,#38616,
#38617,#38618,#38619,#38620,#38621,#38622,#38623,#38624,#38625,#38626,#38627,
#38628,#38629,#38630,#38631,#38632,#38633,#38634,#38635,#38636,#38637,#38638,
#38639,#38640,#38641,#38642,#38643,#38644,#38645,#38646,#38647,#38648,#38649,
#38650,#38651,#38652,#38653,#38654,#38655,#38656,#38657,#38658,#38659,#38660,
#38661,#38662,#38663,#38664,#38665,#38666,#38667,#38668,#38669,#38670,#38671,
#38672,#38673,#38674,#38675,#38676,#38677,#38678,#38679,#38680,#38681,#38682,
#38683,#38684,#38685,#38686,#38687,#38688,#38689,#38690,#38691,#38692,#38693,
#38694,#38695,#38696,#38697,#38698),.UNSPECIFIED.,.F.,.F.,(4,3,3,3,3,3,
3,3,3,3,3,3,3,3,3,3,3,3,3,3,3,3,3,3,3,3,3,3,3,3,3,3,3,3,3,3,3,3,3,3,3,3,
3,3,3,3,3,3,3,3,3,3,3,3,3,3,3,3,4),(30.4997851996723,30.5698066945125,30.6398241339171,
30.7098487763432,30.7798753719464,30.8499153073756,30.8655140038263,30.9355545946528,
31.0055832890939,31.0756042092621,31.1478302304559,31.2178548927196,31.2911815933785,
31.3645082940373,31.4345488848638,31.5045775793049,31.574598499473,31.6468245206668,
31.7168491829305,31.7901758835893,31.8635025842482,31.9335431750747,32.0035718695158,
32.0735927896839,32.1458188108777,32.2158434731413,32.2891701738002,32.3624968744591,
32.4325374652855,32.5025661597266,32.5725870798947,32.6448131010885,32.7148377633521,
32.788164464011,32.86149116467,32.9315317554965,33.0015604499375,33.0715813701056,
33.1438073912994,33.2138320535631,33.287158754222,33.3604854548809,33.4305260457074,
33.5005547401485,33.5705756603166,33.6428016815104,33.712826343774,33.786153044433,
33.8594797450919,33.9295203359184,33.9995490303595,34.0695699505274,34.1417959717213,
34.211820633985,34.2851473346439,34.3584740353028,34.4302564390369,34.5020210945599,
34.557519189415),.UNSPECIFIED.);
#342=B_SPLINE_CURVE_WITH_KNOTS('',3,(#38704,#38705,#38706,#38707,#38708,
#38709,#38710,#38711,#38712,#38713,#38714,#38715,#38716,#38717,#38718,#38719,
#38720,#38721,#38722,#38723,#38724,#38725,#38726,#38727,#38728,#38729,#38730,
#38731,#38732,#38733,#38734,#38735,#38736,#38737,#38738,#38739,#38740,#38741,
#38742,#38743,#38744,#38745,#38746,#38747,#38748,#38749,#38750,#38751,#38752,
#38753,#38754,#38755,#38756,#38757,#38758,#38759,#38760,#38761,#38762,#38763,
#38764,#38765,#38766,#38767,#38768,#38769,#38770,#38771,#38772,#38773,#38774,
#38775,#38776,#38777,#38778,#38779,#38780,#38781,#38782,#38783,#38784,#38785,
#38786,#38787,#38788,#38789,#38790,#38791,#38792,#38793,#38794,#38795,#38796,
#38797,#38798,#38799,#38800,#38801,#38802,#38803,#38804,#38805,#38806,#38807,
#38808,#38809,#38810,#38811,#38812,#38813,#38814,#38815,#38816,#38817,#38818,
#38819,#38820,#38821,#38822,#38823,#38824,#38825,#38826,#38827,#38828,#38829,
#38830,#38831,#38832,#38833,#38834,#38835,#38836,#38837,#38838,#38839,#38840,
#38841,#38842,#38843,#38844,#38845,#38846,#38847,#38848,#38849,#38850,#38851,
#38852,#38853,#38854,#38855,#38856,#38857,#38858,#38859,#38860,#38861,#38862,
#38863,#38864,#38865,#38866,#38867,#38868,#38869,#38870,#38871,#38872,#38873,
#38874,#38875,#38876,#38877,#38878),.UNSPECIFIED.,.F.,.F.,(4,3,3,3,3,3,
3,3,3,3,3,3,3,3,3,3,3,3,3,3,3,3,3,3,3,3,3,3,3,3,3,3,3,3,3,3,3,3,3,3,3,3,
3,3,3,3,3,3,3,3,3,3,3,3,3,3,3,3,4),(24.216566741472,24.2866068494992,24.326893220018,
24.3969338108387,24.4669625052738,24.5369834254368,24.6092094466348,24.6792341088923,
24.7525608095606,24.8258875102289,24.8959281010602,24.9659567955063,25.0359777156793,
25.1082037368695,25.1782283991379,25.2515550997889,25.3248818004398,25.3949223912636,
25.4649510857019,25.5349720058675,25.6071980270633,25.6772226893242,25.7505493899875,
25.8238760906508,25.8939166814786,25.963945375921,26.0339662960902,26.106192317283,
26.1762169795479,26.2495436802048,26.3228703808617,26.3929109716879,26.4629396661284,
26.5329605862962,26.6051866074903,26.6752112697534,26.748537970413,26.8218646710726,
26.8919052618991,26.9619339563401,27.031954876509,27.1041808977026,27.1742055599662,
27.2475322606249,27.3208589612835,27.3908995521103,27.4609282465518,27.5309491667197,
27.6031751879134,27.6731998501771,27.7465265508357,27.8198532514944,27.8896727070108,
27.9594796023928,28.0292786272708,28.0990816217299,28.1688842155913,28.238700456284,
28.2743338822293),.UNSPECIFIED.);
#343=B_SPLINE_CURVE_WITH_KNOTS('',3,(#38879,#38880,#38881,#38882,#38883,
#38884,#38885,#38886,#38887,#38888,#38889,#38890,#38891,#38892,#38893,#38894,
#38895,#38896,#38897,#38898,#38899,#38900,#38901,#38902,#38903,#38904,#38905,
#38906,#38907,#38908,#38909,#38910,#38911,#38912,#38913,#38914,#38915,#38916,
#38917,#38918,#38919,#38920,#38921,#38922,#38923,#38924,#38925,#38926,#38927,
#38928,#38929,#38930,#38931,#38932,#38933,#38934,#38935,#38936,#38937,#38938,
#38939,#38940,#38941,#38942,#38943,#38944,#38945,#38946,#38947,#38948,#38949,
#38950,#38951,#38952,#38953,#38954,#38955,#38956,#38957,#38958,#38959,#38960,
#38961,#38962,#38963,#38964,#38965,#38966,#38967,#38968,#38969,#38970,#38971,
#38972,#38973,#38974,#38975),.UNSPECIFIED.,.F.,.F.,(4,3,3,3,3,3,3,3,3,3,
3,3,3,3,3,3,3,3,3,3,3,3,3,3,3,3,3,3,3,3,3,3,4),(28.2743338823081,28.3188475417054,
28.3888881325318,28.4589168269729,28.5289377471412,28.601163768335,28.6711884305987,
28.7445151312575,28.8178418319163,28.8878824227428,28.9579111171838,29.0279320373515,
29.1001580585454,29.170182720809,29.2435094214681,29.3168361221272,29.3868767129537,
29.4569054073949,29.526926327563,29.5991523487568,29.6691770110205,29.7425037116793,
29.8158304123381,29.8858710031646,29.9558996976058,30.025920617774,30.0981466389678,
30.1681713012315,30.2414980018903,30.3148247025491,30.3848646031318,30.4548937584111,
30.4997797388357),.UNSPECIFIED.);
#344=B_SPLINE_CURVE_WITH_KNOTS('',3,(#38977,#38978,#38979,#38980,#38981,
#38982,#38983,#38984,#38985,#38986,#38987,#38988,#38989,#38990,#38991,#38992,
#38993,#38994,#38995,#38996,#38997,#38998,#38999,#39000,#39001,#39002,#39003,
#39004,#39005,#39006,#39007,#39008,#39009,#39010,#39011,#39012,#39013,#39014,
#39015,#39016,#39017,#39018,#39019,#39020,#39021,#39022,#39023,#39024,#39025,
#39026,#39027,#39028,#39029,#39030,#39031,#39032,#39033,#39034,#39035,#39036,
#39037,#39038,#39039,#39040,#39041,#39042,#39043,#39044,#39045,#39046,#39047,
#39048,#39049,#39050,#39051,#39052,#39053,#39054,#39055,#39056,#39057,#39058,
#39059,#39060,#39061,#39062,#39063,#39064,#39065,#39066,#39067,#39068,#39069,
#39070,#39071,#39072,#39073),.UNSPECIFIED.,.F.,.F.,(4,3,3,3,3,3,3,3,3,3,
3,3,3,3,3,3,3,3,3,3,3,3,3,3,3,3,3,3,3,3,3,3,4),(28.2743338823081,28.3488858316158,
28.3705425527717,28.4405831435994,28.5106118380417,28.5806327582111,28.652858779404,
28.7228834416689,28.7962101423258,28.8695368429826,28.9395774338088,29.0096061282494,
29.0796270484171,29.1518530696112,29.2218777318745,29.295204432534,29.3685311331936,
29.4385717240202,29.5086004184613,29.5786213386295,29.6508473598232,29.7208720220869,
29.7941987227457,29.8675254234045,29.937566014231,30.0075947086721,30.0776156288402,
30.149841650034,30.2198663122976,30.2931930129565,30.3665197136154,30.4365607218776,
30.4997851996723),.UNSPECIFIED.);
#345=B_SPLINE_CURVE_WITH_KNOTS('',3,(#39074,#39075,#39076,#39077,#39078,
#39079,#39080,#39081,#39082,#39083,#39084,#39085,#39086,#39087,#39088,#39089,
#39090,#39091,#39092,#39093,#39094,#39095,#39096,#39097,#39098,#39099,#39100,
#39101,#39102,#39103,#39104,#39105,#39106,#39107,#39108,#39109,#39110,#39111,
#39112,#39113,#39114,#39115,#39116,#39117,#39118,#39119,#39120,#39121,#39122,
#39123,#39124,#39125,#39126,#39127,#39128,#39129,#39130,#39131,#39132,#39133,
#39134,#39135,#39136,#39137,#39138,#39139,#39140,#39141,#39142,#39143,#39144,
#39145,#39146,#39147,#39148,#39149,#39150,#39151,#39152,#39153,#39154,#39155,
#39156,#39157,#39158,#39159,#39160,#39161,#39162,#39163,#39164,#39165,#39166,
#39167,#39168,#39169,#39170,#39171,#39172,#39173,#39174,#39175,#39176,#39177,
#39178,#39179,#39180,#39181,#39182,#39183,#39184,#39185,#39186,#39187,#39188,
#39189,#39190,#39191,#39192,#39193,#39194,#39195,#39196,#39197,#39198,#39199,
#39200,#39201,#39202,#39203,#39204,#39205,#39206,#39207,#39208,#39209,#39210,
#39211,#39212,#39213,#39214,#39215,#39216,#39217,#39218,#39219,#39220,#39221,
#39222,#39223,#39224,#39225,#39226,#39227,#39228,#39229,#39230,#39231,#39232,
#39233,#39234,#39235,#39236,#39237,#39238,#39239,#39240,#39241,#39242,#39243,
#39244,#39245,#39246,#39247,#39248),.UNSPECIFIED.,.F.,.F.,(4,3,3,3,3,3,
3,3,3,3,3,3,3,3,3,3,3,3,3,3,3,3,3,3,3,3,3,3,3,3,3,3,3,3,3,3,3,3,3,3,3,3,
3,3,3,3,3,3,3,3,3,3,3,3,3,3,3,3,4),(24.2165701374682,24.2865963860171,24.356636287462,
24.3785882310843,24.4486288215852,24.5186575156965,24.5886784355325,24.6609044569732,
24.7309291189008,24.804255820098,24.8775825212953,24.9476231122925,25.0176518069063,
25.0876727272481,25.1598987483126,25.2299234107518,25.303250111129,25.3765768115062,
25.4466174022641,25.5166460966359,25.5866670167347,25.6588930379803,25.7289177001737,
25.8022444009454,25.8755711017171,25.9456116925611,26.0156403870197,26.0856613072058,
26.1578873283863,26.2279119906679,26.3012386912979,26.374565391928,26.4446059827562,
26.5146346771987,26.5846555973683,26.6568816185609,26.7269062808266,26.8002329814827,
26.8735596821389,26.9436002729597,27.0136289673946,27.0836498875575,27.1558759087556,
27.2259005710137,27.2992272716818,27.3725539723499,27.4425945631809,27.5126232576271,
27.5826441778001,27.6548701989903,27.7248948612584,27.7982215619096,27.8715482625608,
27.9413131725913,28.0110652143382,28.0808150034561,28.1505602216933,28.2203156472821,
28.2743338822406),.UNSPECIFIED.);
#346=B_SPLINE_CURVE_WITH_KNOTS('',3,(#39254,#39255,#39256,#39257,#39258,
#39259,#39260,#39261,#39262),.UNSPECIFIED.,.F.,.F.,(4,1,1,1,1,1,4),(15.7079632679489,
15.8956852974986,16.3946795877096,16.8936738779205,17.3926681681314,17.8916624583423,
17.9334121841373),.UNSPECIFIED.);
#347=B_SPLINE_CURVE_WITH_KNOTS('',3,(#39264,#39265,#39266,#39267,#39268,
#39269),.UNSPECIFIED.,.F.,.F.,(4,1,1,4),(14.3987024268659,14.8976967170768,
15.3966910072877,15.7079632679489),.UNSPECIFIED.);
#348=B_SPLINE_CURVE_WITH_KNOTS('',3,(#39273,#39274,#39275,#39276,#39277,
#39278,#39279,#39280,#39281,#39282,#39283,#39284,#39285,#39286,#39287,#39288,
#39289,#39290,#39291,#39292,#39293,#39294,#39295,#39296,#39297,#39298,#39299,
#39300,#39301,#39302,#39303,#39304,#39305,#39306,#39307,#39308,#39309,#39310,
#39311,#39312,#39313,#39314,#39315,#39316,#39317,#39318,#39319,#39320,#39321,
#39322,#39323,#39324,#39325,#39326,#39327,#39328,#39329,#39330,#39331,#39332,
#39333,#39334,#39335,#39336,#39337,#39338,#39339,#39340,#39341,#39342,#39343,
#39344,#39345,#39346,#39347,#39348,#39349,#39350,#39351,#39352,#39353,#39354),
 .UNSPECIFIED.,.F.,.F.,(4,3,3,3,3,3,3,3,3,3,3,3,3,3,3,3,3,3,3,3,3,3,3,3,
3,3,3,4),(13.8756314554422,13.9455244015096,14.0154054819089,14.085279198689,
14.1551582454853,14.2250368331584,14.2949311931912,14.3470074157995,14.4170482343004,
14.487077175958,14.5570983621865,14.6293241981425,14.6993491698426,14.7726754379265,
14.8460017060104,14.9160393182244,14.9860649926552,15.0560828595175,15.1283111436935,
15.198332708346,15.2716643522837,15.3449959962214,15.4148686130277,15.488142276758,
15.5579967616873,15.6278466788921,15.697700868083,15.7079632679489),
 .UNSPECIFIED.);
#349=B_SPLINE_CURVE_WITH_KNOTS('',3,(#39355,#39356,#39357,#39358,#39359,
#39360,#39361,#39362,#39363,#39364,#39365,#39366,#39367,#39368,#39369,#39370,
#39371,#39372,#39373,#39374,#39375,#39376,#39377,#39378,#39379,#39380,#39381,
#39382,#39383,#39384,#39385,#39386,#39387,#39388,#39389,#39390,#39391,#39392,
#39393,#39394,#39395,#39396,#39397,#39398,#39399,#39400,#39401,#39402,#39403,
#39404,#39405,#39406,#39407,#39408,#39409,#39410,#39411,#39412,#39413,#39414,
#39415,#39416,#39417,#39418,#39419,#39420,#39421,#39422,#39423,#39424,#39425,
#39426,#39427,#39428,#39429,#39430,#39431,#39432,#39433,#39434,#39435,#39436,
#39437,#39438,#39439,#39440,#39441,#39442,#39443,#39444,#39445,#39446,#39447,
#39448,#39449,#39450,#39451),.UNSPECIFIED.,.F.,.F.,(4,3,3,3,3,3,3,3,3,3,
3,3,3,3,3,3,3,3,3,3,3,3,3,3,3,3,3,3,3,3,3,3,4),(15.7079632680278,15.781258546969,
15.8439902864323,15.9140293859905,15.9840565719878,16.0540759705774,16.1263031220939,
16.1963262492752,16.2696554129592,16.3429845766432,16.4130258394328,16.4830552130784,
16.5530768178735,16.6253023301186,16.6953276818739,16.768653274364,16.8419788668541,
16.9120192399517,16.9820477145933,17.0520684134795,17.1242945993759,17.1943190394544,
17.2676460982597,17.3409731570651,17.4110137716016,17.4810424897669,17.5510634336108,
17.6232894370271,17.6933141225493,17.7666407849127,17.839967447276,17.9100073812242,
17.933415291275),.UNSPECIFIED.);
#350=B_SPLINE_CURVE_WITH_KNOTS('',3,(#39457,#39458,#39459,#39460,#39461,
#39462,#39463,#39464,#39465,#39466,#39467,#39468,#39469,#39470,#39471,#39472,
#39473,#39474,#39475,#39476,#39477,#39478,#39479,#39480,#39481,#39482,#39483,
#39484,#39485,#39486,#39487,#39488,#39489,#39490,#39491,#39492,#39493,#39494,
#39495,#39496,#39497,#39498,#39499,#39500,#39501,#39502,#39503,#39504,#39505,
#39506,#39507,#39508,#39509,#39510,#39511,#39512,#39513,#39514,#39515,#39516,
#39517,#39518,#39519,#39520,#39521,#39522,#39523,#39524,#39525,#39526),
 .UNSPECIFIED.,.F.,.F.,(4,3,3,3,3,3,3,3,3,3,3,3,3,3,3,3,3,3,3,3,3,3,3,4),
(42.3163681282077,42.389003921528,42.4145146679284,42.48729869792,42.5600703328061,
42.632833872698,42.7056024032701,42.7783690429379,42.8511510266575,42.9135089581394,
42.9859787125309,43.0584354826672,43.1308844455598,43.2033410888313,43.275797773863,
43.3482751674385,43.4125032483503,43.4856192267066,43.5587218933442,43.6318145250677,
43.7049066040599,43.7779931512484,43.8510867420094,43.9114975385612),
 .UNSPECIFIED.);
#351=B_SPLINE_CURVE_WITH_KNOTS('',3,(#39529,#39530,#39531,#39532,#39533,
#39534,#39535,#39536,#39537,#39538,#39539,#39540,#39541,#39542,#39543,#39544,
#39545,#39546,#39547,#39548,#39549,#39550,#39551,#39552,#39553,#39554,#39555,
#39556,#39557,#39558,#39559,#39560,#39561,#39562,#39563,#39564,#39565,#39566,
#39567,#39568,#39569,#39570,#39571,#39572,#39573,#39574,#39575,#39576,#39577,
#39578,#39579,#39580),.UNSPECIFIED.,.F.,.F.,(4,2,2,2,2,2,2,2,2,2,2,2,2,
2,2,2,2,2,2,2,2,2,2,2,2,4),(-44.0788261103538,-43.9100592942155,-43.7715029329665,
-43.7074184572621,-43.6112929604573,-43.4302409268727,-43.2699713391976,
-43.0774948020758,-42.9661053858083,-42.8280933119776,-42.6572261911526,
-42.5615004460577,-42.3810883050336,-42.2202473083055,-42.0277910513795,
-41.9140420430288,-41.7767841864719,-41.610215244241,-41.5129059215617,
-41.4051211968993,-41.2624970586652,-41.0648615614014,-40.9791137834735,
-40.8748767190918,-40.7342210145313,-40.6004689346889),.UNSPECIFIED.);
#352=B_SPLINE_CURVE_WITH_KNOTS('',3,(#39586,#39587,#39588,#39589,#39590,
#39591,#39592,#39593,#39594,#39595),.UNSPECIFIED.,.F.,.F.,(4,1,1,1,1,1,
1,4),(36.0332287400247,36.4265831853974,36.9255774756083,37.4245717658192,
37.9235660560301,38.4225603462411,38.921554636452,39.0083726841606),
 .UNSPECIFIED.);
#353=B_SPLINE_CURVE_WITH_KNOTS('',3,(#39596,#39597,#39598,#39599,#39600,
#39601,#39602,#39603,#39604,#39605,#39606,#39607,#39608,#39609,#39610,#39611,
#39612,#39613,#39614,#39615,#39616,#39617,#39618,#39619,#39620,#39621,#39622,
#39623,#39624,#39625,#39626,#39627,#39628,#39629,#39630,#39631,#39632,#39633,
#39634,#39635,#39636,#39637,#39638,#39639,#39640,#39641,#39642,#39643,#39644,
#39645,#39646,#39647,#39648,#39649,#39650,#39651,#39652,#39653,#39654,#39655,
#39656,#39657,#39658,#39659,#39660,#39661,#39662,#39663,#39664,#39665,#39666,
#39667,#39668,#39669,#39670,#39671,#39672,#39673,#39674,#39675,#39676,#39677,
#39678,#39679,#39680,#39681,#39682,#39683,#39684,#39685,#39686,#39687,#39688,
#39689,#39690,#39691,#39692,#39693,#39694,#39695,#39696,#39697,#39698,#39699,
#39700,#39701,#39702,#39703,#39704,#39705,#39706,#39707,#39708,#39709,#39710,
#39711,#39712,#39713,#39714,#39715,#39716,#39717,#39718,#39719,#39720,#39721,
#39722,#39723,#39724,#39725,#39726,#39727,#39728,#39729,#39730,#39731,#39732,
#39733,#39734,#39735,#39736,#39737),.UNSPECIFIED.,.F.,.F.,(4,3,3,3,3,3,
3,3,3,3,3,3,3,3,3,3,3,3,3,3,3,3,3,3,3,3,3,3,3,3,3,3,3,3,3,3,3,3,3,3,3,3,
3,3,3,3,3,4),(39.0083726877398,39.0807497775609,39.1531170797185,39.225488567641,
39.2978589558457,39.3702461345474,39.4205489266629,39.4932256719064,39.5658896866155,
39.6385455807479,39.711207210472,39.7838675238172,39.8565448817808,39.9195432168738,
39.9922242628658,40.0648925892348,40.1375527937686,40.2102187009694,40.2828832672999,
40.3555648079552,40.4185375070847,40.4912126225807,40.5638750101892,40.6365292843827,
40.7091893168006,40.7818480476756,40.8545238586228,40.9175317972957,40.9902104856699,
41.062876431308,41.1355342389029,41.2081977415302,41.2808599026547,41.353539054321,
41.4165260875066,41.4892161017965,41.561893459126,41.6345627313086,41.7072376971513,
41.7799113036542,41.8526017895961,41.9155203777175,41.9881552979112,42.0607769946022,
42.1333953792814,42.2060085346025,42.2786289307035,42.3163681282077),
 .UNSPECIFIED.);
#354=B_SPLINE_CURVE_WITH_KNOTS('',3,(#39738,#39739,#39740,#39741,#39742,
#39743,#39744,#39745,#39746,#39747,#39748,#39749,#39750,#39751,#39752,#39753,
#39754,#39755,#39756,#39757,#39758,#39759,#39760,#39761,#39762,#39763,#39764,
#39765,#39766,#39767,#39768,#39769,#39770,#39771,#39772,#39773,#39774,#39775,
#39776,#39777,#39778,#39779,#39780,#39781,#39782,#39783,#39784,#39785,#39786,
#39787,#39788,#39789,#39790,#39791,#39792,#39793,#39794,#39795,#39796,#39797,
#39798,#39799,#39800,#39801,#39802,#39803,#39804,#39805,#39806,#39807,#39808,
#39809,#39810,#39811,#39812,#39813,#39814,#39815,#39816,#39817,#39818,#39819,
#39820,#39821,#39822,#39823,#39824,#39825,#39826,#39827,#39828,#39829,#39830,
#39831,#39832,#39833,#39834,#39835,#39836,#39837,#39838,#39839),
 .UNSPECIFIED.,.F.,.F.,(4,2,2,2,2,2,2,2,2,2,2,2,2,2,2,2,2,2,2,2,2,2,2,2,
2,2,2,2,2,2,2,2,2,2,2,2,2,2,2,2,2,2,2,2,2,2,2,2,2,2,4),(-40.6004689346889,
-40.5382784573951,-40.4534405320164,-40.3416795319586,-40.2037368545846,
-40.0326379413695,-39.9370698191387,-39.8251955624539,-39.6845032915067,
-39.4885263073456,-39.403674714177,-39.2918929257224,-39.1539481787511,
-38.9828339395382,-38.8872668655935,-38.7067744022686,-38.5459606666476,
-38.3535424066591,-38.2397373413956,-38.1024465050108,-37.9357284554644,
-37.8384839479232,-37.7304538855592,-37.5879176504572,-37.3903593908053,
-37.304622440894,-37.2004669159065,-37.0597470509154,-36.8637359886231,
-36.7788689324912,-36.667072666136,-36.5291062499929,-36.3579734505362,
-36.2623864991692,-36.0819166913421,-35.9210530384614,-35.7285782081487,
-35.6147565473853,-35.4774450105914,-35.310701862699,-35.2134429347374,
-35.1053958777011,-34.962838858293,-34.7652516189409,-34.6795019382082,
-34.5753295110467,-34.4345891017111,-34.2385490090928,-34.1536696820834,
-34.0418530693211,-33.9901053404391),.UNSPECIFIED.);
#355=B_SPLINE_CURVE_WITH_KNOTS('',3,(#39845,#39846,#39847,#39848,#39849,
#39850,#39851,#39852,#39853,#39854,#39855,#39856,#39857,#39858,#39859,#39860,
#39861,#39862,#39863,#39864,#39865,#39866,#39867,#39868,#39869,#39870,#39871,
#39872,#39873,#39874,#39875,#39876,#39877,#39878,#39879,#39880,#39881,#39882,
#39883,#39884,#39885,#39886,#39887,#39888),.UNSPECIFIED.,.F.,.F.,(4,2,2,
2,2,2,2,2,2,2,2,2,2,2,2,2,2,2,2,2,2,4),(-3.12972961237737,-3.02357540757013,
-2.9118472766391,-2.82699219400489,-2.63100103262062,-2.49030154085052,
-2.38757442686493,-2.30338638173099,-2.10758954946452,-1.96765695708937,
-1.86128621636086,-1.66893810480045,-1.5071366225871,-1.33126439654607,
-1.23915881419717,-1.05929928033435,-0.920096409516259,-0.811915618831055,
-0.619563874526152,-0.458108313007325,-0.280274621053177,-9.05352858358878E-5),
 .UNSPECIFIED.);
#356=B_SPLINE_CURVE_WITH_KNOTS('',3,(#39889,#39890,#39891,#39892,#39893,
#39894,#39895,#39896,#39897,#39898,#39899),.UNSPECIFIED.,.F.,.F.,(4,1,1,
1,1,1,1,1,4),(32.725187376981,32.9336231539209,33.4326174441318,33.9316117343428,
34.4306060245537,34.9296003147646,35.4285946049755,35.9275888951864,36.0332287400247),
 .UNSPECIFIED.);
#357=B_SPLINE_CURVE_WITH_KNOTS('',3,(#39900,#39901,#39902,#39903,#39904,
#39905,#39906,#39907,#39908,#39909,#39910,#39911,#39912,#39913,#39914,#39915,
#39916,#39917,#39918,#39919,#39920,#39921,#39922,#39923,#39924,#39925,#39926,
#39927,#39928,#39929,#39930,#39931,#39932,#39933,#39934,#39935,#39936,#39937,
#39938,#39939,#39940,#39941,#39942,#39943,#39944,#39945,#39946,#39947,#39948,
#39949,#39950,#39951,#39952,#39953,#39954,#39955,#39956,#39957,#39958,#39959,
#39960,#39961,#39962,#39963,#39964,#39965,#39966,#39967,#39968,#39969,#39970,
#39971,#39972,#39973,#39974,#39975,#39976,#39977,#39978,#39979,#39980,#39981,
#39982,#39983,#39984,#39985,#39986,#39987,#39988,#39989,#39990,#39991,#39992,
#39993,#39994,#39995),.UNSPECIFIED.,.F.,.F.,(4,2,2,2,2,2,2,2,2,2,2,2,2,
2,2,2,2,2,2,2,2,2,2,2,2,2,2,2,2,2,2,2,2,2,2,2,2,2,2,2,2,2,2,2,2,2,2,4),
(-33.9901053404391,-33.9038673318948,-33.7327011419815,-33.637106182711,
-33.4565608324522,-33.2956990203788,-33.1032226333052,-32.9893828405317,
-32.8520512012745,-32.6852812141468,-32.5880094929732,-32.479942641251,
-32.3373661984005,-32.1397513242891,-32.0539895105622,-31.9498084148103,
-31.8090448132149,-31.6129742235052,-31.5280807487632,-31.4162587573692,
-31.2782486103253,-31.1070816380028,-31.0114528472798,-30.8310388829762,
-30.670069132821,-30.4774319561785,-30.3631025817692,-30.2258998761992,
-30.0582964428501,-29.9617041394288,-29.8519653702877,-29.7101594091751,
-29.5132722958157,-29.427812221667,-29.3194457043472,-29.1801681390832,
-29.0002019561717,-28.9080559415564,-28.7321128205142,-28.5701604041746,
-28.3774966919828,-28.2702927158626,-28.1305494704203,-27.9507188228387,
-27.8579567925644,-27.6805464113609,-27.5190867418308,-27.3770201043626),
 .UNSPECIFIED.);
#358=B_SPLINE_CURVE_WITH_KNOTS('',3,(#40000,#40001,#40002,#40003,#40004,
#40005,#40006,#40007,#40008,#40009,#40010,#40011,#40012,#40013,#40014,#40015,
#40016,#40017,#40018,#40019,#40020,#40021,#40022,#40023,#40024,#40025,#40026,
#40027,#40028,#40029,#40030,#40031,#40032,#40033,#40034,#40035,#40036,#40037,
#40038,#40039,#40040,#40041,#40042,#40043,#40044,#40045,#40046,#40047,#40048,
#40049,#40050,#40051,#40052,#40053,#40054,#40055,#40056,#40057,#40058,#40059,
#40060,#40061,#40062,#40063,#40064,#40065,#40066,#40067,#40068,#40069,#40070,
#40071,#40072,#40073,#40074,#40075,#40076,#40077,#40078,#40079,#40080,#40081,
#40082,#40083,#40084,#40085,#40086,#40087,#40088,#40089,#40090,#40091,#40092,
#40093,#40094,#40095,#40096,#40097,#40098,#40099),.UNSPECIFIED.,.F.,.F.,
(4,2,2,2,2,2,2,2,2,2,2,2,2,2,2,2,2,2,2,2,2,2,2,2,2,2,2,2,2,2,2,2,2,2,2,
2,2,2,2,2,2,2,2,2,2,2,2,2,2,4),(-9.73964911326357,-9.65894423564208,-9.52165405446729,
-9.3550271395587,-9.25772955066524,-9.14984664875812,-9.0072582203635,-8.8096536995634,
-8.72390183789383,-8.61720571772894,-8.47737195858178,-8.28150856230035,
-8.19745982266304,-8.09412525168699,-7.95365224694775,-7.75777396042404,
-7.67308436584228,-7.55990517587196,-7.42241227653874,-7.24394313945267,
-7.15319218095859,-6.98064229341811,-6.81757845654217,-6.68181777293533,
-6.60983127964453,-6.48324291880089,-6.31089336699378,-6.17277800050596,
-6.06145328491304,-5.97652415069389,-5.78044190248597,-5.63962740124722,
-5.5370822032355,-5.34422406511019,-5.18331135139813,-5.003004613449,-4.90741064099126,
-4.73631665844469,-4.59836968489508,-4.48660310628703,-4.40174350696052,
-4.2057366129771,-4.06502900376254,-3.96227941747858,-3.76913349288581,
-3.60798908702072,-3.42816805541769,-3.33253521362127,-3.16151849539383,
-3.12972961237737),.UNSPECIFIED.);
#359=B_SPLINE_CURVE_WITH_KNOTS('',3,(#40100,#40101,#40102,#40103,#40104,
#40105,#40106,#40107,#40108,#40109,#40110,#40111,#40112,#40113,#40114,#40115,
#40116,#40117,#40118,#40119,#40120,#40121,#40122,#40123,#40124,#40125,#40126,
#40127,#40128,#40129,#40130,#40131,#40132,#40133,#40134,#40135,#40136,#40137,
#40138,#40139,#40140,#40141,#40142,#40143,#40144,#40145,#40146,#40147,#40148,
#40149,#40150,#40151,#40152,#40153,#40154,#40155,#40156,#40157,#40158,#40159,
#40160,#40161,#40162,#40163,#40164,#40165,#40166,#40167,#40168,#40169,#40170,
#40171,#40172,#40173,#40174,#40175,#40176,#40177,#40178,#40179,#40180,#40181,
#40182,#40183,#40184,#40185,#40186,#40187,#40188,#40189,#40190,#40191,#40192,
#40193,#40194,#40195,#40196,#40197,#40198,#40199),.UNSPECIFIED.,.F.,.F.,
(4,2,2,2,2,2,2,2,2,2,2,2,2,2,2,2,2,2,2,2,2,2,2,2,2,2,2,2,2,2,2,2,2,2,2,
2,2,2,2,2,2,2,2,2,2,2,2,2,2,4),(-27.3770201043626,-27.3259869988704,-27.2121100458388,
-27.0747318318027,-26.907907677031,-26.8106015462648,-26.7025019622452,
-26.5598757460337,-26.3621925865554,-26.276401273343,-26.1721783179693,
-26.031369543728,-25.835234238612,-25.7503136825854,-25.6384428300776,-25.5003900650916,
-25.3291408924148,-25.2334994027494,-25.1215330292327,-24.980722116227,
-24.7845791659393,-24.6996577482217,-24.587751418088,-24.4497009256982,
-24.2783782653954,-24.1827821137484,-24.0018061486208,-23.8410358604269,
-23.648313506953,-23.5456683319773,-23.4047387851586,-23.208514119051,-23.1235150604426,
-23.0121125410751,-22.8738727807086,-22.7013677308331,-22.6062089414503,
-22.4931655671665,-22.3528244948875,-22.1626309692493,-22.0396620413223,
-21.8456830127117,-21.6867004145244,-21.5047151786164,-21.4130670928768,
-21.2333822520101,-21.0946713588781,-20.984635287894,-20.89943271034,-20.7616952607919),
 .UNSPECIFIED.);
#360=B_SPLINE_CURVE_WITH_KNOTS('',3,(#40205,#40206,#40207,#40208,#40209,
#40210,#40211,#40212,#40213,#40214,#40215,#40216,#40217,#40218,#40219,#40220,
#40221,#40222,#40223,#40224,#40225,#40226,#40227,#40228,#40229,#40230,#40231,
#40232,#40233,#40234,#40235,#40236,#40237,#40238,#40239,#40240,#40241,#40242,
#40243,#40244,#40245,#40246,#40247,#40248,#40249,#40250,#40251,#40252),
 .UNSPECIFIED.,.F.,.F.,(4,2,2,2,2,2,2,2,2,2,2,2,2,2,2,2,2,2,2,2,2,2,2,4),
(-3.1291763693966,-3.06051423746629,-2.92058449029293,-2.81420514005639,
-2.62190166055115,-2.46014874464375,-2.28413518085184,-2.19197068595235,
-2.01208501479044,-1.87281886403111,-1.7648008422835,-1.67935277495058,
-1.48248212458146,-1.3406588528544,-1.23128928405176,-1.13465866826387,
-0.967307336117015,-0.830191190375465,-0.716028156243458,-0.52358859575441,
-0.362789859682845,-0.261165452376227,-0.169848216096543,-9.06239312916104E-5),
 .UNSPECIFIED.);
#361=B_SPLINE_CURVE_WITH_KNOTS('',3,(#40253,#40254,#40255,#40256,#40257,
#40258,#40259,#40260,#40261,#40262,#40263,#40264,#40265,#40266,#40267,#40268,
#40269,#40270,#40271,#40272,#40273,#40274,#40275,#40276,#40277,#40278,#40279,
#40280,#40281,#40282,#40283,#40284,#40285,#40286,#40287,#40288,#40289,#40290,
#40291,#40292,#40293,#40294,#40295,#40296,#40297,#40298,#40299,#40300,#40301,
#40302),.UNSPECIFIED.,.F.,.F.,(4,2,2,2,2,2,2,2,2,2,2,2,2,2,2,2,2,2,2,2,
2,2,2,2,4),(-13.2194666776149,-12.9315530398099,-12.75122112135,-12.589908851332,
-12.3969841603575,-12.2832071728717,-12.1459516433032,-11.9792739482411,
-11.8820560811831,-11.7740494421549,-11.6315517500151,-11.4340460508408,
-11.3483315663086,-11.2442051653794,-11.1035204605134,-10.9075589984911,
-10.8227130527622,-10.7109499613579,-10.5730172528488,-10.4019388774833,
-10.3063678811762,-10.126014625418,-9.96515477963546,-9.77269368223828,
-9.73964911326357),.UNSPECIFIED.);
#362=B_SPLINE_CURVE_WITH_KNOTS('',3,(#40303,#40304,#40305,#40306,#40307,
#40308,#40309,#40310,#40311,#40312,#40313,#40314,#40315,#40316,#40317,#40318,
#40319,#40320,#40321,#40322,#40323,#40324,#40325,#40326,#40327,#40328,#40329,
#40330,#40331,#40332,#40333,#40334,#40335,#40336,#40337,#40338,#40339,#40340,
#40341,#40342,#40343,#40344,#40345,#40346,#40347,#40348,#40349,#40350,#40351,
#40352,#40353,#40354,#40355,#40356,#40357,#40358,#40359,#40360,#40361,#40362,
#40363,#40364,#40365,#40366,#40367,#40368,#40369,#40370,#40371,#40372,#40373,
#40374,#40375,#40376,#40377,#40378,#40379,#40380,#40381,#40382,#40383,#40384,
#40385,#40386,#40387,#40388,#40389,#40390,#40391,#40392,#40393,#40394,#40395,
#40396,#40397,#40398),.UNSPECIFIED.,.F.,.F.,(4,2,2,2,2,2,2,2,2,2,2,2,2,
2,2,2,2,2,2,2,2,2,2,2,2,2,2,2,2,2,2,2,2,2,2,2,2,2,2,2,2,2,2,2,2,2,2,4),
(-20.7616952607919,-20.7029496957438,-20.5616751617043,-20.4598332609485,
-20.3752879168612,-20.1793086272156,-20.0389735427187,-19.9259781567096,
-19.830811580402,-19.6583753171218,-19.5201676949303,-19.4087472888494,
-19.323760071219,-19.1275406855933,-18.9866294727618,-18.8840041560849,
-18.6906355469538,-18.5292460976927,-18.3515792968921,-18.2587033595283,
-18.0792230303878,-17.9395673429201,-17.8321166758214,-17.6396150280574,
-17.4778874941757,-17.3012505448391,-17.2088095322091,-17.0287011678067,
-16.8891105195559,-16.7815262771041,-16.5890128193696,-16.427297435627,
-16.2506692805385,-16.1582332097997,-15.9781367449341,-15.8385542371383,
-15.7309808305531,-15.5384940691259,-15.3768029696543,-15.2001485340552,
-15.1077027118569,-14.9276141391687,-14.7880249429551,-14.6805000622446,
-14.4879272859893,-14.326137266756,-14.1498118449496,-14.1472447933216),
 .UNSPECIFIED.);
#363=B_SPLINE_CURVE_WITH_KNOTS('',3,(#40403,#40404,#40405,#40406,#40407,
#40408,#40409,#40410,#40411,#40412,#40413,#40414,#40415,#40416,#40417,#40418,
#40419,#40420,#40421,#40422,#40423,#40424,#40425,#40426,#40427,#40428,#40429,
#40430,#40431,#40432,#40433,#40434,#40435,#40436,#40437,#40438,#40439,#40440,
#40441,#40442,#40443,#40444,#40445,#40446,#40447,#40448,#40449,#40450,#40451,
#40452,#40453,#40454,#40455,#40456,#40457,#40458,#40459,#40460,#40461,#40462,
#40463,#40464,#40465,#40466,#40467,#40468,#40469,#40470,#40471,#40472,#40473,
#40474,#40475,#40476,#40477,#40478,#40479,#40480,#40481,#40482,#40483,#40484,
#40485,#40486,#40487,#40488,#40489,#40490,#40491,#40492,#40493,#40494,#40495,
#40496),.UNSPECIFIED.,.F.,.F.,(4,2,2,2,2,2,2,2,2,2,2,2,2,2,2,2,2,2,2,2,
2,2,2,2,2,2,2,2,2,2,2,2,2,2,2,2,2,2,2,2,2,2,2,2,2,2,4),(-9.73907321948152,
-9.68207929033005,-9.50606682630167,-9.34429241933644,-9.15174505724938,
-9.04418921938962,-8.90471039453844,-8.72475108610191,-8.63238861275138,
-8.4558984142504,-8.29427536776061,-8.10176496422375,-7.99359727989772,
-7.85434396130632,-7.67445500876044,-7.58231096741114,-7.40634697865959,
-7.24452603681246,-7.05199716640114,-6.94479278155016,-6.80515102333529,
-6.60907326560968,-6.49007026026039,-6.29718462836577,-6.13630043188297,
-5.95593809362674,-5.86035028525291,-5.6892474537243,-5.55130125481543,
-5.4395305186487,-5.35467110717155,-5.15866392769172,-5.01795654371566,
-4.91520488564753,-4.72235805791818,-4.56150317778389,-4.38113214900285,
-4.28555670779011,-4.11446637221707,-3.97653408287644,-3.86477229610324,
-3.77992130119884,-3.58393321331188,-3.44323974315957,-3.3404971617921,
-3.25631275523785,-3.1291763693966),.UNSPECIFIED.);
#364=B_SPLINE_CURVE_WITH_KNOTS('',3,(#40497,#40498,#40499,#40500,#40501,
#40502,#40503,#40504,#40505,#40506,#40507,#40508,#40509,#40510,#40511,#40512,
#40513,#40514,#40515,#40516,#40517,#40518,#40519,#40520,#40521,#40522,#40523,
#40524,#40525,#40526,#40527,#40528,#40529,#40530,#40531,#40532,#40533,#40534,
#40535,#40536,#40537,#40538,#40539,#40540,#40541,#40542,#40543,#40544,#40545,
#40546,#40547,#40548,#40549,#40550,#40551,#40552,#40553,#40554,#40555,#40556,
#40557,#40558,#40559,#40560,#40561,#40562,#40563,#40564,#40565,#40566,#40567,
#40568,#40569,#40570,#40571,#40572,#40573,#40574,#40575,#40576,#40577,#40578,
#40579,#40580,#40581,#40582,#40583,#40584,#40585,#40586,#40587,#40588,#40589,
#40590,#40591,#40592,#40593,#40594),.UNSPECIFIED.,.F.,.F.,(4,2,2,2,2,2,
2,2,2,2,2,2,2,2,2,2,2,2,2,2,2,2,2,2,2,2,2,2,2,2,2,2,2,2,2,2,2,2,2,2,2,2,
2,2,2,2,2,2,4),(-14.1472447933216,-14.0575049034936,-13.8774699909368,-13.7380261550839,
-13.6301613925409,-13.5446124284645,-13.3475129133717,-13.2054895048621,
-13.0962773970659,-12.9994925420233,-12.8321382968731,-12.6949129619141,
-12.5807375184919,-12.3881730793577,-12.2272643235089,-12.0467975217235,
-11.9511856625091,-11.7800223315118,-11.642034203121,-11.530225553396,-11.4453399801411,
-11.2492718413425,-11.1085208405746,-11.0057366599301,-10.9215177099878,
-10.7256392876854,-10.5856521355424,-10.4792301701748,-10.2867797134512,
-10.1248885606261,-9.94900977779425,-9.85689350345923,-9.67697256748017,
-9.53774173278488,-9.42943981513686,-9.23675780060404,-9.07499128425171,
-8.89879946346959,-8.80655398530214,-8.62658737009246,-8.48722110161676,
-8.37930287719263,-8.29379866125501,-8.0968018075072,-7.95486647715765,
-7.84559633168378,-7.74887863963778,-7.58153365577835,-7.53564154876179),
 .UNSPECIFIED.);
#365=B_SPLINE_CURVE_WITH_KNOTS('',3,(#40600,#40601,#40602,#40603,#40604,
#40605,#40606,#40607,#40608,#40609,#40610,#40611,#40612,#40613),
 .UNSPECIFIED.,.F.,.F.,(4,2,2,2,2,2,4),(-0.926590328528814,-0.753955484513565,
-0.6139958295923,-0.515954230626158,-0.443702087204974,-0.243068847343075,
-0.000135688299652575),.UNSPECIFIED.);
#366=B_SPLINE_CURVE_WITH_KNOTS('',3,(#40616,#40617,#40618,#40619,#40620,
#40621,#40622,#40623,#40624,#40625,#40626,#40627,#40628,#40629,#40630,#40631,
#40632,#40633,#40634,#40635,#40636,#40637,#40638,#40639,#40640,#40641,#40642,
#40643,#40644,#40645,#40646,#40647,#40648,#40649,#40650,#40651,#40652,#40653,
#40654,#40655,#40656,#40657,#40658,#40659,#40660,#40661,#40662,#40663,#40664,
#40665,#40666,#40667,#40668,#40669,#40670,#40671,#40672,#40673,#40674,#40675,
#40676,#40677,#40678,#40679,#40680,#40681,#40682,#40683,#40684,#40685,#40686,
#40687,#40688,#40689,#40690,#40691,#40692,#40693,#40694,#40695,#40696,#40697,
#40698,#40699,#40700,#40701,#40702,#40703,#40704,#40705,#40706,#40707,#40708,
#40709,#40710,#40711,#40712,#40713,#40714,#40715,#40716,#40717,#40718,#40719,
#40720,#40721,#40722,#40723,#40724,#40725,#40726,#40727),.UNSPECIFIED.,
 .F.,.F.,(4,3,3,3,3,3,3,3,3,3,3,3,3,3,3,3,3,3,3,3,3,3,3,3,3,3,3,3,3,3,3,
3,3,3,3,3,3,4),(2.02359556728784,2.09612063785746,2.16863302303831,2.24113775293914,
2.31364811582229,2.38615861296181,2.45868474905377,2.49497145105461,2.56765002727523,
2.64031589890252,2.71297367059207,2.78563719645063,2.85829941345175,2.93097867400525,
2.99396574126554,3.06664098081929,3.13930345029594,3.21195776421116,3.28461777093719,
3.35727644001194,3.42995213051997,3.49296003147646,3.56564099670242,3.63830926977429,
3.71096944845288,3.78363537238572,3.85629997895852,3.92898159803042,3.99195432168738,
4.06463110674485,4.13729514772772,4.20995105460738,4.28261267608537,4.35527296959603,
4.42795028890617,4.49094861189831,4.56362770609116,4.61729307130943),
 .UNSPECIFIED.);
#367=B_SPLINE_CURVE_WITH_KNOTS('',3,(#40730,#40731,#40732,#40733,#40734,
#40735,#40736,#40737,#40738,#40739,#40740,#40741,#40742,#40743,#40744,#40745,
#40746,#40747,#40748,#40749,#40750,#40751,#40752,#40753,#40754,#40755,#40756,
#40757,#40758,#40759,#40760,#40761,#40762,#40763,#40764,#40765,#40766,#40767,
#40768,#40769,#40770,#40771,#40772,#40773,#40774,#40775,#40776,#40777,#40778,
#40779,#40780,#40781,#40782,#40783,#40784,#40785,#40786,#40787,#40788,#40789,
#40790,#40791,#40792,#40793,#40794,#40795,#40796,#40797,#40798,#40799,#40800,
#40801,#40802,#40803,#40804,#40805,#40806,#40807,#40808,#40809,#40810,#40811,
#40812,#40813,#40814,#40815,#40816,#40817,#40818,#40819,#40820,#40821,#40822,
#40823,#40824,#40825,#40826,#40827,#40828,#40829,#40830,#40831,#40832,#40833,
#40834,#40835,#40836,#40837,#40838,#40839,#40840,#40841,#40842,#40843,#40844,
#40845,#40846,#40847,#40848,#40849,#40850,#40851,#40852,#40853,#40854,#40855,
#40856),.UNSPECIFIED.,.F.,.F.,(4,3,3,3,3,3,3,3,3,3,3,3,3,3,3,3,3,3,3,3,
3,3,3,3,3,3,3,3,3,3,3,3,3,3,3,3,3,3,3,3,3,3,4),(4.61729307130943,4.68995293710172,
4.7649504283536,4.83761291716063,4.91377790963493,4.98994290210923,5.06262100423254,
5.13528637842111,5.20794363080203,5.280606607111,5.35326825861506,5.42594693144097,
5.48893719232016,5.56161554328838,5.63428116853687,5.70693867347046,5.77960190281452,
5.85226380724567,5.92494273101668,5.98793148253108,6.06060984370026,6.13327547967456,
6.20593299582697,6.27859623707525,6.35125815377287,6.42393709031945,6.486925772742,
6.55960406326347,6.63226962758147,6.70492707127597,6.77759023934746,6.85025208257815,
6.92293094570417,6.98592006295293,7.05859841273454,7.13126403706467,7.20392154135016,
7.27658477047137,7.3492466749157,7.42192559908852,7.48491435316385,7.56187309461106,
7.59244614826265),.UNSPECIFIED.);
#368=B_SPLINE_CURVE_WITH_KNOTS('',3,(#40857,#40858,#40859,#40860,#40861,
#40862,#40863,#40864,#40865,#40866,#40867,#40868,#40869,#40870,#40871,#40872,
#40873,#40874,#40875,#40876,#40877,#40878,#40879,#40880,#40881,#40882,#40883,
#40884,#40885,#40886,#40887,#40888,#40889,#40890,#40891,#40892,#40893,#40894,
#40895,#40896,#40897,#40898,#40899,#40900,#40901,#40902,#40903,#40904,#40905,
#40906),.UNSPECIFIED.,.F.,.F.,(4,2,2,2,2,2,2,2,2,2,2,2,2,2,2,2,2,2,2,2,
2,2,2,2,4),(-13.2184356728779,-13.0690661818794,-12.9182477272931,-12.8289515586441,
-12.6545072282153,-12.4931147641064,-12.3007284920065,-12.1919123903746,
-12.0529529736406,-11.8732347157786,-11.7813473250141,-11.6059894283038,
-11.4440147867751,-11.2513298643328,-11.1440427766819,-11.0044821083306,
-10.8245209291215,-10.7320706544749,-10.5553651898818,-10.3938460406952,
-10.2014560813668,-10.0933860004824,-9.95411910849321,-9.7742410176212,
-9.73907321948152),.UNSPECIFIED.);
#369=B_SPLINE_CURVE_WITH_KNOTS('',3,(#40907,#40908,#40909,#40910,#40911,
#40912,#40913,#40914,#40915,#40916,#40917,#40918,#40919,#40920,#40921,#40922,
#40923,#40924,#40925,#40926,#40927,#40928,#40929,#40930,#40931,#40932,#40933,
#40934,#40935,#40936,#40937,#40938,#40939,#40940,#40941,#40942,#40943,#40944,
#40945,#40946,#40947,#40948,#40949,#40950,#40951,#40952,#40953,#40954,#40955,
#40956,#40957,#40958,#40959,#40960,#40961,#40962,#40963,#40964,#40965,#40966,
#40967,#40968,#40969,#40970,#40971,#40972,#40973,#40974,#40975,#40976,#40977,
#40978,#40979,#40980,#40981,#40982,#40983,#40984,#40985,#40986,#40987,#40988,
#40989,#40990,#40991,#40992,#40993,#40994,#40995,#40996,#40997,#40998,#40999,
#41000,#41001,#41002,#41003,#41004,#41005,#41006),.UNSPECIFIED.,.F.,.F.,
(4,2,2,2,2,2,2,2,2,2,2,2,2,2,2,2,2,2,2,2,2,2,2,2,2,2,2,2,2,2,2,2,2,2,2,
2,2,2,2,2,2,2,2,2,2,2,2,2,2,4),(-7.53564154876179,-7.44435895692881,-7.33019444534583,
-7.24560723684192,-7.0497538285448,-6.90940624634637,-6.79677075262341,
-6.7015593268547,-6.52958416487551,-6.39153932403596,-6.28004969084625,
-6.19514425977817,-5.99908544723558,-5.85829995364484,-5.75572199185766,
-5.67149445949106,-5.47569870552628,-5.33574083826483,-5.22938458578421,
-5.14353261448337,-4.94556272004269,-4.80263040407831,-4.69544159686438,
-4.59782648178253,-4.43158586807976,-4.29425923625493,-4.18071001141288,
-3.9881945699854,-3.8272860352096,-3.64697769618344,-3.55122885095793,-3.3828040614263,
-3.24580686616462,-3.13127629889031,-2.93878885368664,-2.77879708127779,
-2.59757913471578,-2.5020689489392,-2.33058784772183,-2.19201882225214,
-2.08183329883684,-1.89039846798437,-1.73322226283244,-1.54238350525133,
-1.43850896943895,-1.27779998733979,-1.13690736638403,-1.03040158727961,
-0.943996000995363,-0.926590328528814),.UNSPECIFIED.);
#370=B_SPLINE_CURVE_WITH_KNOTS('',3,(#41009,#41010,#41011,#41012,#41013,
#41014,#41015,#41016,#41017,#41018,#41019,#41020,#41021,#41022,#41023,#41024,
#41025,#41026,#41027,#41028,#41029,#41030,#41031,#41032,#41033,#41034,#41035,
#41036,#41037,#41038,#41039,#41040,#41041,#41042,#41043,#41044,#41045,#41046,
#41047,#41048,#41049,#41050,#41051,#41052,#41053,#41054,#41055,#41056,#41057,
#41058,#41059,#41060,#41061,#41062,#41063,#41064,#41065,#41066,#41067,#41068,
#41069,#41070,#41071,#41072,#41073,#41074,#41075,#41076,#41077,#41078,#41079,
#41080,#41081,#41082,#41083,#41084,#41085,#41086,#41087,#41088,#41089,#41090,
#41091,#41092,#41093,#41094,#41095,#41096,#41097,#41098,#41099,#41100,#41101,
#41102,#41103,#41104,#41105,#41106,#41107,#41108,#41109,#41110,#41111,#41112,
#41113,#41114,#41115,#41116,#41117,#41118,#41119,#41120,#41121,#41122,#41123,
#41124,#41125,#41126,#41127,#41128,#41129,#41130,#41131,#41132,#41133,#41134,
#41135,#41136,#41137,#41138,#41139,#41140,#41141,#41142,#41143,#41144,#41145,
#41146,#41147,#41148,#41149,#41150,#41151,#41152,#41153,#41154,#41155,#41156,
#41157,#41158,#41159,#41160,#41161,#41162,#41163,#41164,#41165,#41166,#41167,
#41168,#41169,#41170,#41171,#41172,#41173,#41174,#41175,#41176,#41177,#41178,
#41179,#41180,#41181,#41182,#41183),.UNSPECIFIED.,.F.,.F.,(4,3,3,3,3,3,
3,3,3,3,3,3,3,3,3,3,3,3,3,3,3,3,3,3,3,3,3,3,3,3,3,3,3,3,3,3,3,3,3,3,3,3,
3,3,3,3,3,3,3,3,3,3,3,3,3,3,3,3,4),(17.933415291275,18.0034409627842,18.0734602373726,
18.1434856452887,18.2135106587962,18.2835513152064,18.3389617374869,18.4090022932936,
18.4790309522727,18.5490518366316,18.6212778843982,18.6913025104407,18.7646292690693,
18.8379560276978,18.9079966408986,18.9780253579764,19.048046300983,19.1202723052145,
19.1902969905308,19.2636236542198,19.3369503179088,19.406990897852,19.47701958129,
19.5470404903645,19.6192665198033,19.6892911708883,19.762617889504,19.8359446081197,
19.9059852029146,19.9760139013638,20.0460348255693,20.1182608437596,20.1882855100817,
20.2616122042062,20.3349388983306,20.4049794883864,20.4750081820518,20.5450291014412,
20.6172551232163,20.6872797847037,20.7606064866226,20.8339331885415,20.9039737790573,
20.9740024731822,21.0440233930295,21.1162494144602,21.1862740763956,21.259600777574,
21.3329274787524,21.4029680700421,21.4729967649525,21.5430176855947,21.6152437064369,
21.6852683691804,21.7585950690719,21.8319217689634,21.9045986695098,21.9772545252523,
21.9911485750577),.UNSPECIFIED.);
#371=B_SPLINE_CURVE_WITH_KNOTS('',3,(#41184,#41185,#41186,#41187,#41188,
#41189,#41190,#41191,#41192,#41193,#41194,#41195,#41196,#41197,#41198,#41199,
#41200,#41201,#41202,#41203,#41204,#41205,#41206,#41207,#41208,#41209,#41210,
#41211,#41212,#41213,#41214,#41215,#41216,#41217,#41218,#41219,#41220,#41221,
#41222,#41223,#41224,#41225,#41226,#41227,#41228,#41229,#41230,#41231,#41232,
#41233,#41234,#41235,#41236,#41237,#41238,#41239,#41240,#41241,#41242,#41243,
#41244,#41245,#41246,#41247,#41248,#41249,#41250,#41251,#41252,#41253,#41254,
#41255,#41256,#41257,#41258,#41259,#41260,#41261,#41262,#41263,#41264,#41265,
#41266,#41267,#41268,#41269,#41270,#41271,#41272,#41273,#41274,#41275,#41276,
#41277,#41278,#41279,#41280),.UNSPECIFIED.,.F.,.F.,(4,3,3,3,3,3,3,3,3,3,
3,3,3,3,3,3,3,3,3,3,3,3,3,3,3,3,3,3,3,3,3,3,4),(21.9911485751285,22.0611187640108,
22.1310953555668,22.2010715824223,22.2710644969389,22.3309160591743,22.4009566501728,
22.4709853447878,22.541006265131,22.6132322861946,22.683256948635,22.7565836490101,
22.8299103493852,22.8999509401425,22.9699796345137,23.0400005546109,23.1122265758572,
23.18225123805,23.2555779388231,23.3289046395961,23.3989452304404,23.4689739248994,
23.5389948450855,23.6112208662659,23.6812455285476,23.7545722291773,23.8278989298071,
23.8979388431038,23.9679665406906,24.0379905648376,24.1080093565331,24.1780338634582,
24.216566741472),.UNSPECIFIED.);
#372=B_SPLINE_CURVE_WITH_KNOTS('',3,(#41282,#41283,#41284,#41285,#41286,
#41287,#41288,#41289,#41290,#41291,#41292,#41293,#41294,#41295,#41296,#41297,
#41298,#41299,#41300,#41301,#41302,#41303,#41304,#41305,#41306,#41307,#41308,
#41309,#41310,#41311,#41312,#41313,#41314,#41315,#41316,#41317,#41318,#41319,
#41320,#41321,#41322,#41323,#41324,#41325,#41326,#41327,#41328,#41329,#41330,
#41331,#41332,#41333,#41334,#41335,#41336,#41337,#41338,#41339,#41340,#41341,
#41342,#41343,#41344,#41345,#41346,#41347,#41348,#41349,#41350,#41351,#41352,
#41353,#41354,#41355,#41356,#41357,#41358,#41359,#41360,#41361,#41362,#41363,
#41364,#41365,#41366,#41367,#41368,#41369,#41370,#41371,#41372,#41373,#41374,
#41375,#41376,#41377,#41378),.UNSPECIFIED.,.F.,.F.,(4,3,3,3,3,3,3,3,3,3,
3,3,3,3,3,3,3,3,3,3,3,3,3,3,3,3,3,3,3,3,3,3,4),(21.9911485751285,22.0609174698852,
22.1306788205048,22.2004452722809,22.2702117236623,22.339993679049,22.3826110702406,
22.4526516650052,22.522680363424,22.5927012875987,22.6649273058119,22.7349519721031,
22.8082786662773,22.8816053604516,22.9516459505158,23.0216746441895,23.0916955635876,
23.1639215853563,23.2339462468523,23.3072729487574,23.3805996506625,23.4506402411789,
23.5206689353042,23.5906898551522,23.6629158765825,23.7329405385186,23.806267239696,
23.8795939408734,23.9496338916419,24.0196644904711,24.0896860414985,24.1597095893078,
24.2165701374682),.UNSPECIFIED.);
#373=B_SPLINE_CURVE_WITH_KNOTS('',3,(#41379,#41380,#41381,#41382,#41383,
#41384,#41385,#41386,#41387,#41388,#41389,#41390),.UNSPECIFIED.,.F.,.F.,
(4,1,1,1,1,1,1,1,1,4),(17.9334121841373,18.3906567485533,18.8896510387642,
19.3886453289751,19.887639619186,20.386633909397,20.8856281996079,21.3846224898188,
21.8836167800297,21.9911485751285),.UNSPECIFIED.);
#374=B_SPLINE_CURVE_WITH_KNOTS('',3,(#41756,#41757,#41758,#41759,#41760,
#41761,#41762,#41763,#41764,#41765,#41766,#41767,#41768,#41769,#41770,#41771,
#41772,#41773,#41774,#41775,#41776,#41777,#41778,#41779,#41780,#41781,#41782,
#41783,#41784,#41785,#41786,#41787,#41788,#41789,#41790,#41791,#41792,#41793,
#41794,#41795,#41796,#41797,#41798,#41799,#41800,#41801,#41802,#41803,#41804,
#41805,#41806,#41807,#41808,#41809,#41810,#41811,#41812,#41813,#41814,#41815,
#41816,#41817,#41818,#41819,#41820,#41821,#41822,#41823,#41824,#41825,#41826,
#41827,#41828,#41829,#41830,#41831,#41832,#41833,#41834,#41835,#41836,#41837,
#41838,#41839,#41840,#41841,#41842,#41843,#41844,#41845,#41846,#41847,#41848,
#41849,#41850,#41851,#41852,#41853,#41854,#41855,#41856,#41857,#41858,#41859,
#41860,#41861,#41862,#41863,#41864,#41865,#41866,#41867,#41868,#41869,#41870,
#41871,#41872,#41873,#41874,#41875,#41876),.UNSPECIFIED.,.F.,.F.,(4,3,3,
3,3,3,3,3,3,3,3,3,3,3,3,3,3,3,3,3,3,3,3,3,3,3,3,3,3,3,3,3,3,3,3,3,3,3,3,
3,4),(0.,0.0847077516938065,0.170225033901306,0.255907500614097,0.341119279334384,
0.425059357872854,0.455383656591401,0.465770691009882,0.474513364932373,
0.55829834295187,0.600642802906426,0.684662560232657,0.76868652492825,0.851862297560265,
0.912900878915177,0.924214418880625,0.933065505594978,1.0153136859126,1.09836343076413,
1.18141317561567,1.26373325194704,1.3454132435303,1.36175593088453,1.37449997082537,
1.45485338293641,1.53535345085992,1.61538859693277,1.69412331541584,1.74187144182578,
1.78111905912933,1.79651186347856,1.80847555122129,1.88768501760864,1.96689410761267,
2.04543359578892,2.05585238025418,2.07005430058833,2.14795915885765,2.22484263433871,
2.28089532743822,2.31010750305873),.UNSPECIFIED.);
#375=B_SPLINE_CURVE_WITH_KNOTS('',3,(#41877,#41878,#41879,#41880,#41881,
#41882,#41883,#41884,#41885,#41886,#41887,#41888,#41889,#41890,#41891,#41892,
#41893,#41894,#41895,#41896,#41897,#41898,#41899,#41900,#41901,#41902,#41903,
#41904,#41905,#41906,#41907,#41908,#41909,#41910,#41911,#41912,#41913,#41914,
#41915,#41916,#41917,#41918,#41919,#41920,#41921,#41922,#41923,#41924,#41925,
#41926,#41927,#41928,#41929,#41930,#41931,#41932,#41933,#41934,#41935,#41936,
#41937,#41938,#41939,#41940,#41941,#41942,#41943,#41944,#41945,#41946,#41947,
#41948,#41949,#41950,#41951,#41952,#41953,#41954,#41955,#41956,#41957,#41958,
#41959,#41960,#41961,#41962,#41963,#41964,#41965,#41966,#41967,#41968,#41969,
#41970,#41971,#41972,#41973,#41974,#41975,#41976,#41977,#41978,#41979,#41980,
#41981,#41982,#41983,#41984,#41985,#41986,#41987,#41988,#41989,#41990,#41991),
 .UNSPECIFIED.,.F.,.F.,(4,3,3,3,3,3,3,3,3,3,3,3,3,3,3,3,3,3,3,3,3,3,3,3,
3,3,3,3,3,3,3,3,3,3,3,3,3,3,4),(0.,0.0756021000860287,0.152393199413229,
0.230392842039223,0.308644925336307,0.386546669540438,0.408880923643587,
0.422045036141436,0.501691131541529,0.537249170842264,0.616137946028814,
0.695699298413659,0.775607582803438,0.834608203354004,0.843321085046558,
0.924172696188012,1.00955071586659,1.09492873554517,1.18019567138666,1.26546260722815,
1.27900992162839,1.28771744272705,1.3694636855273,1.45259721932159,1.53602421303522,
1.61905253984465,1.6726411664557,1.7128618032572,1.72976589346393,1.74248623587268,
1.82597852348531,1.91057121440841,1.99440626086767,2.0125183165509,2.02643670804109,
2.11207588022372,2.19783429700933,2.26933164573093,2.30291422475425),
 .UNSPECIFIED.);
#376=B_SPLINE_CURVE_WITH_KNOTS('',3,(#41992,#41993,#41994,#41995),
 .UNSPECIFIED.,.F.,.F.,(4,4),(-0.00101470513518961,0.),.UNSPECIFIED.);
#377=B_SPLINE_CURVE_WITH_KNOTS('',3,(#42360,#42361,#42362,#42363,#42364,
#42365,#42366,#42367,#42368,#42369,#42370,#42371,#42372,#42373,#42374,#42375,
#42376,#42377,#42378,#42379,#42380,#42381,#42382,#42383,#42384,#42385,#42386,
#42387,#42388,#42389,#42390,#42391,#42392,#42393,#42394,#42395,#42396,#42397,
#42398,#42399,#42400,#42401,#42402,#42403,#42404,#42405,#42406,#42407,#42408,
#42409,#42410,#42411,#42412,#42413,#42414,#42415,#42416,#42417,#42418,#42419,
#42420,#42421,#42422,#42423,#42424,#42425,#42426,#42427,#42428,#42429,#42430,
#42431,#42432,#42433,#42434,#42435,#42436,#42437,#42438,#42439,#42440,#42441,
#42442,#42443,#42444,#42445,#42446,#42447,#42448,#42449,#42450,#42451,#42452,
#42453,#42454,#42455,#42456,#42457,#42458,#42459,#42460,#42461,#42462,#42463,
#42464,#42465,#42466,#42467,#42468,#42469,#42470,#42471,#42472,#42473,#42474),
 .UNSPECIFIED.,.F.,.F.,(4,3,3,3,3,3,3,3,3,3,3,3,3,3,3,3,3,3,3,3,3,3,3,3,
3,3,3,3,3,3,3,3,3,3,3,3,3,3,4),(0.,0.0756020442574548,0.152393097282484,
0.230392716822797,0.308644794442198,0.386546558051837,0.408880856230141,
0.420928744427606,0.50056989933121,0.537249170842273,0.616073663427341,
0.695678467127519,0.775598187384106,0.815514505904238,0.834608291732455,
0.848410336526209,0.929311979470198,1.01212035750768,1.09492873554516,1.1760664859709,
1.25762667198288,1.27900990554167,1.28771743639829,1.3694636568822,1.45259718086404,
1.53602417093209,1.61905249850157,1.6726411664557,1.73231431654345,1.74174492869213,
1.82529436366377,1.90959642787817,1.99435898893753,2.01251832412271,2.02375496071478,
2.10938057767908,2.19514471613238,2.26933164573094,2.30291844692703),
 .UNSPECIFIED.);
#378=B_SPLINE_CURVE_WITH_KNOTS('',3,(#42475,#42476,#42477,#42478,#42479,
#42480,#42481,#42482,#42483,#42484,#42485,#42486,#42487,#42488,#42489,#42490,
#42491,#42492,#42493,#42494,#42495,#42496,#42497,#42498,#42499,#42500,#42501,
#42502,#42503,#42504,#42505,#42506,#42507,#42508,#42509,#42510,#42511,#42512,
#42513,#42514,#42515,#42516,#42517,#42518,#42519,#42520,#42521,#42522,#42523,
#42524,#42525,#42526,#42527,#42528,#42529,#42530,#42531,#42532,#42533,#42534,
#42535,#42536,#42537,#42538,#42539,#42540,#42541,#42542,#42543,#42544,#42545,
#42546,#42547,#42548,#42549,#42550,#42551,#42552,#42553,#42554,#42555,#42556,
#42557,#42558,#42559,#42560,#42561,#42562,#42563,#42564,#42565,#42566,#42567,
#42568,#42569,#42570,#42571,#42572,#42573,#42574,#42575,#42576,#42577,#42578,
#42579,#42580,#42581,#42582,#42583,#42584,#42585,#42586,#42587,#42588,#42589,
#42590,#42591,#42592,#42593,#42594,#42595,#42596,#42597,#42598),
 .UNSPECIFIED.,.F.,.F.,(4,3,3,3,3,3,3,3,3,3,3,3,3,3,3,3,3,3,3,3,3,3,3,3,
3,3,3,3,3,3,3,3,3,3,3,3,3,3,3,3,3,4),(6.61845341725208E-15,0.0849506171234813,
0.170583039080586,0.256324783642234,0.342404288458281,0.406963917070316,
0.455383638529342,0.468536166026273,0.479421865762467,0.563197401537396,
0.600642802906421,0.684641773439803,0.768646494241719,0.852075754316474,
0.893242931978871,0.912628999576665,0.923529204381824,0.932945920282631,
0.963808296830803,1.04604185775375,1.12763182076683,1.18141317561565,1.26548811560765,
1.34956305559966,1.36175593015859,1.37449997074551,1.45485337915234,1.53535344654489,
1.61538859022719,1.69412330072992,1.74187144182573,1.79625541798791,1.80632110746682,
1.88551239813011,1.96470047938476,2.04374919139812,2.05752087843184,2.07312514683444,
2.15101428972444,2.22787487685276,2.28089532743819,2.31010750305869),
 .UNSPECIFIED.);
#394=FACE_BOUND('',#1042,.T.);
#395=FACE_BOUND('',#1050,.T.);
#484=CYLINDRICAL_SURFACE('',#4431,12.1745);
#485=CYLINDRICAL_SURFACE('',#4433,12.1745);
#486=CYLINDRICAL_SURFACE('',#4434,12.1745);
#487=CYLINDRICAL_SURFACE('',#4435,12.1745);
#488=CYLINDRICAL_SURFACE('',#4436,12.1745);
#489=CYLINDRICAL_SURFACE('',#4437,12.1745);
#490=CYLINDRICAL_SURFACE('',#4438,12.1745);
#491=CYLINDRICAL_SURFACE('',#4440,10.501);
#492=CYLINDRICAL_SURFACE('',#4442,10.501);
#493=CYLINDRICAL_SURFACE('',#4443,10.501);
#494=CYLINDRICAL_SURFACE('',#4444,10.501);
#495=CYLINDRICAL_SURFACE('',#4445,10.501);
#496=CYLINDRICAL_SURFACE('',#4446,10.501);
#497=CYLINDRICAL_SURFACE('',#4447,10.501);
#498=CYLINDRICAL_SURFACE('',#4449,10.501);
#499=CYLINDRICAL_SURFACE('',#4450,12.1745);
#634=CIRCLE('',#4432,12.1745);
#635=CIRCLE('',#4439,12.1745);
#636=CIRCLE('',#4441,10.501);
#637=CIRCLE('',#4448,10.501);
#810=FACE_OUTER_BOUND('',#1023,.T.);
#811=FACE_OUTER_BOUND('',#1024,.T.);
#812=FACE_OUTER_BOUND('',#1025,.T.);
#813=FACE_OUTER_BOUND('',#1026,.T.);
#814=FACE_OUTER_BOUND('',#1027,.T.);
#815=FACE_OUTER_BOUND('',#1028,.T.);
#816=FACE_OUTER_BOUND('',#1029,.T.);
#817=FACE_OUTER_BOUND('',#1030,.T.);
#818=FACE_OUTER_BOUND('',#1031,.T.);
#819=FACE_OUTER_BOUND('',#1032,.T.);
#820=FACE_OUTER_BOUND('',#1033,.T.);
#821=FACE_OUTER_BOUND('',#1034,.T.);
#822=FACE_OUTER_BOUND('',#1035,.T.);
#823=FACE_OUTER_BOUND('',#1036,.T.);
#824=FACE_OUTER_BOUND('',#1037,.T.);
#825=FACE_OUTER_BOUND('',#1038,.T.);
#826=FACE_OUTER_BOUND('',#1039,.T.);
#827=FACE_OUTER_BOUND('',#1040,.T.);
#828=FACE_OUTER_BOUND('',#1041,.T.);
#829=FACE_OUTER_BOUND('',#1043,.T.);
#830=FACE_OUTER_BOUND('',#1044,.T.);
#831=FACE_OUTER_BOUND('',#1045,.T.);
#832=FACE_OUTER_BOUND('',#1046,.T.);
#833=FACE_OUTER_BOUND('',#1047,.T.);
#834=FACE_OUTER_BOUND('',#1048,.T.);
#835=FACE_OUTER_BOUND('',#1049,.T.);
#1023=EDGE_LOOP('',(#3588,#3589,#3590,#3591));
#1024=EDGE_LOOP('',(#3592,#3593,#3594,#3595,#3596,#3597));
#1025=EDGE_LOOP('',(#3598,#3599,#3600,#3601,#3602,#3603));
#1026=EDGE_LOOP('',(#3604,#3605,#3606,#3607,#3608,#3609));
#1027=EDGE_LOOP('',(#3610,#3611,#3612,#3613,#3614,#3615));
#1028=EDGE_LOOP('',(#3616,#3617,#3618,#3619,#3620,#3621));
#1029=EDGE_LOOP('',(#3622,#3623,#3624,#3625,#3626,#3627));
#1030=EDGE_LOOP('',(#3628,#3629,#3630,#3631));
#1031=EDGE_LOOP('',(#3632,#3633,#3634,#3635,#3636));
#1032=EDGE_LOOP('',(#3637,#3638,#3639,#3640,#3641));
#1033=EDGE_LOOP('',(#3642,#3643,#3644,#3645));
#1034=EDGE_LOOP('',(#3646,#3647,#3648,#3649,#3650));
#1035=EDGE_LOOP('',(#3651,#3652,#3653,#3654));
#1036=EDGE_LOOP('',(#3655,#3656,#3657,#3658));
#1037=EDGE_LOOP('',(#3659,#3660,#3661,#3662,#3663));
#1038=EDGE_LOOP('',(#3664,#3665,#3666,#3667,#3668,#3669));
#1039=EDGE_LOOP('',(#3670,#3671,#3672,#3673,#3674,#3675,#3676,#3677,#3678,
#3679,#3680,#3681,#3682,#3683,#3684,#3685,#3686,#3687,#3688,#3689,#3690,
#3691,#3692,#3693,#3694,#3695));
#1040=EDGE_LOOP('',(#3696,#3697,#3698,#3699,#3700,#3701,#3702,#3703,#3704,
#3705,#3706,#3707,#3708,#3709,#3710,#3711,#3712,#3713,#3714,#3715,#3716,
#3717,#3718,#3719,#3720,#3721,#3722,#3723,#3724));
#1041=EDGE_LOOP('',(#3725,#3726,#3727,#3728,#3729,#3730));
#1042=EDGE_LOOP('',(#3731,#3732,#3733,#3734,#3735));
#1043=EDGE_LOOP('',(#3736,#3737,#3738,#3739));
#1044=EDGE_LOOP('',(#3740,#3741,#3742,#3743));
#1045=EDGE_LOOP('',(#3744,#3745,#3746,#3747));
#1046=EDGE_LOOP('',(#3748,#3749,#3750,#3751));
#1047=EDGE_LOOP('',(#3752,#3753,#3754,#3755));
#1048=EDGE_LOOP('',(#3756,#3757,#3758,#3759));
#1049=EDGE_LOOP('',(#3760,#3761,#3762,#3763,#3764,#3765));
#1050=EDGE_LOOP('',(#3766,#3767,#3768,#3769));
#1232=LINE('',#36921,#1445);
#1233=LINE('',#36937,#1446);
#1234=LINE('',#37306,#1447);
#1235=LINE('',#37853,#1448);
#1236=LINE('',#38241,#1449);
#1237=LINE('',#38702,#1450);
#1238=LINE('',#39252,#1451);
#1239=LINE('',#39455,#1452);
#1240=LINE('',#39584,#1453);
#1241=LINE('',#39843,#1454);
#1242=LINE('',#39999,#1455);
#1243=LINE('',#40203,#1456);
#1244=LINE('',#40402,#1457);
#1245=LINE('',#40598,#1458);
#1246=LINE('',#42602,#1459);
#1247=LINE('',#42604,#1460);
#1248=LINE('',#42606,#1461);
#1249=LINE('',#42608,#1462);
#1250=LINE('',#42610,#1463);
#1251=LINE('',#42611,#1464);
#1252=LINE('',#42615,#1465);
#1253=LINE('',#42616,#1466);
#1254=LINE('',#42617,#1467);
#1255=LINE('',#42620,#1468);
#1256=LINE('',#42621,#1469);
#1257=LINE('',#42624,#1470);
#1258=LINE('',#42625,#1471);
#1259=LINE('',#42628,#1472);
#1260=LINE('',#42629,#1473);
#1261=LINE('',#42632,#1474);
#1262=LINE('',#42633,#1475);
#1263=LINE('',#42635,#1476);
#1445=VECTOR('',#5231,12.1745);
#1446=VECTOR('',#5236,12.1745);
#1447=VECTOR('',#5239,12.1745);
#1448=VECTOR('',#5242,12.1745);
#1449=VECTOR('',#5245,12.1745);
#1450=VECTOR('',#5248,12.1745);
#1451=VECTOR('',#5251,12.1745);
#1452=VECTOR('',#5256,10.501);
#1453=VECTOR('',#5261,10.501);
#1454=VECTOR('',#5264,10.501);
#1455=VECTOR('',#5267,10.501);
#1456=VECTOR('',#5270,10.501);
#1457=VECTOR('',#5273,10.501);
#1458=VECTOR('',#5276,10.501);
#1459=VECTOR('',#5285,10.);
#1460=VECTOR('',#5286,10.);
#1461=VECTOR('',#5287,10.);
#1462=VECTOR('',#5288,10.);
#1463=VECTOR('',#5289,10.);
#1464=VECTOR('',#5290,10.);
#1465=VECTOR('',#5293,10.);
#1466=VECTOR('',#5294,10.);
#1467=VECTOR('',#5295,10.);
#1468=VECTOR('',#5298,10.);
#1469=VECTOR('',#5299,10.);
#1470=VECTOR('',#5302,10.);
#1471=VECTOR('',#5303,10.);
#1472=VECTOR('',#5306,10.);
#1473=VECTOR('',#5307,10.);
#1474=VECTOR('',#5310,10.);
#1475=VECTOR('',#5311,10.);
#1476=VECTOR('',#5314,10.);
#1852=VERTEX_POINT('',#36919);
#1853=VERTEX_POINT('',#36920);
#1854=VERTEX_POINT('',#36922);
#1855=VERTEX_POINT('',#36927);
#1856=VERTEX_POINT('',#36935);
#1857=VERTEX_POINT('',#36936);
#1858=VERTEX_POINT('',#36938);
#1859=VERTEX_POINT('',#37119);
#1860=VERTEX_POINT('',#37304);
#1861=VERTEX_POINT('',#37305);
#1862=VERTEX_POINT('',#37307);
#1863=VERTEX_POINT('',#37580);
#1864=VERTEX_POINT('',#37851);
#1865=VERTEX_POINT('',#37852);
#1866=VERTEX_POINT('',#37854);
#1867=VERTEX_POINT('',#37965);
#1868=VERTEX_POINT('',#38239);
#1869=VERTEX_POINT('',#38240);
#1870=VERTEX_POINT('',#38242);
#1871=VERTEX_POINT('',#38426);
#1872=VERTEX_POINT('',#38700);
#1873=VERTEX_POINT('',#38701);
#1874=VERTEX_POINT('',#38703);
#1875=VERTEX_POINT('',#38976);
#1876=VERTEX_POINT('',#39250);
#1877=VERTEX_POINT('',#39251);
#1878=VERTEX_POINT('',#39253);
#1879=VERTEX_POINT('',#39263);
#1880=VERTEX_POINT('',#39270);
#1881=VERTEX_POINT('',#39272);
#1882=VERTEX_POINT('',#39453);
#1883=VERTEX_POINT('',#39454);
#1884=VERTEX_POINT('',#39456);
#1885=VERTEX_POINT('',#39527);
#1886=VERTEX_POINT('',#39582);
#1887=VERTEX_POINT('',#39583);
#1888=VERTEX_POINT('',#39585);
#1889=VERTEX_POINT('',#39841);
#1890=VERTEX_POINT('',#39842);
#1891=VERTEX_POINT('',#39844);
#1892=VERTEX_POINT('',#39997);
#1893=VERTEX_POINT('',#39998);
#1894=VERTEX_POINT('',#40201);
#1895=VERTEX_POINT('',#40202);
#1896=VERTEX_POINT('',#40204);
#1897=VERTEX_POINT('',#40400);
#1898=VERTEX_POINT('',#40401);
#1899=VERTEX_POINT('',#40596);
#1900=VERTEX_POINT('',#40597);
#1901=VERTEX_POINT('',#40599);
#1902=VERTEX_POINT('',#40614);
#1903=VERTEX_POINT('',#40729);
#1904=VERTEX_POINT('',#41008);
#1905=VERTEX_POINT('',#41281);
#1906=VERTEX_POINT('',#41755);
#1907=VERTEX_POINT('',#42600);
#1908=VERTEX_POINT('',#42601);
#1909=VERTEX_POINT('',#42603);
#1910=VERTEX_POINT('',#42605);
#1911=VERTEX_POINT('',#42607);
#1912=VERTEX_POINT('',#42609);
#1913=VERTEX_POINT('',#42613);
#1914=VERTEX_POINT('',#42614);
#1915=VERTEX_POINT('',#42619);
#1916=VERTEX_POINT('',#42623);
#1917=VERTEX_POINT('',#42627);
#1918=VERTEX_POINT('',#42631);
#2445=EDGE_CURVE('',#1852,#1853,#1232,.T.);
#2446=EDGE_CURVE('',#1853,#1854,#324,.T.);
#2447=EDGE_CURVE('',#1855,#1854,#634,.T.);
#2448=EDGE_CURVE('',#1852,#1855,#325,.T.);
#2449=EDGE_CURVE('',#1856,#1857,#1233,.T.);
#2450=EDGE_CURVE('',#1857,#1858,#326,.T.);
#2451=EDGE_CURVE('',#1858,#1853,#327,.T.);
#2452=EDGE_CURVE('',#1859,#1852,#328,.T.);
#2453=EDGE_CURVE('',#1856,#1859,#329,.T.);
#2454=EDGE_CURVE('',#1860,#1861,#1234,.T.);
#2455=EDGE_CURVE('',#1861,#1862,#330,.T.);
#2456=EDGE_CURVE('',#1862,#1857,#331,.T.);
#2457=EDGE_CURVE('',#1863,#1856,#332,.T.);
#2458=EDGE_CURVE('',#1860,#1863,#333,.T.);
#2459=EDGE_CURVE('',#1864,#1865,#1235,.T.);
#2460=EDGE_CURVE('',#1865,#1866,#334,.T.);
#2461=EDGE_CURVE('',#1866,#1861,#335,.T.);
#2462=EDGE_CURVE('',#1867,#1860,#336,.T.);
#2463=EDGE_CURVE('',#1864,#1867,#337,.T.);
#2464=EDGE_CURVE('',#1868,#1869,#1236,.T.);
#2465=EDGE_CURVE('',#1869,#1870,#338,.T.);
#2466=EDGE_CURVE('',#1870,#1865,#339,.T.);
#2467=EDGE_CURVE('',#1871,#1864,#340,.T.);
#2468=EDGE_CURVE('',#1868,#1871,#341,.T.);
#2469=EDGE_CURVE('',#1872,#1873,#1237,.T.);
#2470=EDGE_CURVE('',#1873,#1874,#342,.T.);
#2471=EDGE_CURVE('',#1874,#1869,#343,.T.);
#2472=EDGE_CURVE('',#1875,#1868,#344,.T.);
#2473=EDGE_CURVE('',#1872,#1875,#345,.T.);
#2474=EDGE_CURVE('',#1876,#1877,#1238,.T.);
#2475=EDGE_CURVE('',#1878,#1876,#346,.T.);
#2476=EDGE_CURVE('',#1879,#1878,#347,.T.);
#2477=EDGE_CURVE('',#1880,#1879,#635,.T.);
#2478=EDGE_CURVE('',#1880,#1881,#348,.T.);
#2479=EDGE_CURVE('',#1881,#1877,#349,.T.);
#2480=EDGE_CURVE('',#1882,#1883,#1239,.T.);
#2481=EDGE_CURVE('',#1883,#1884,#350,.T.);
#2482=EDGE_CURVE('',#1885,#1884,#636,.F.);
#2483=EDGE_CURVE('',#1885,#1882,#351,.T.);
#2484=EDGE_CURVE('',#1886,#1887,#1240,.T.);
#2485=EDGE_CURVE('',#1887,#1888,#352,.T.);
#2486=EDGE_CURVE('',#1888,#1883,#353,.T.);
#2487=EDGE_CURVE('',#1882,#1886,#354,.T.);
#2488=EDGE_CURVE('',#1889,#1890,#1241,.T.);
#2489=EDGE_CURVE('',#1890,#1891,#355,.T.);
#2490=EDGE_CURVE('',#1891,#1887,#356,.T.);
#2491=EDGE_CURVE('',#1886,#1889,#357,.T.);
#2492=EDGE_CURVE('',#1892,#1893,#1242,.T.);
#2493=EDGE_CURVE('',#1893,#1890,#358,.T.);
#2494=EDGE_CURVE('',#1889,#1892,#359,.T.);
#2495=EDGE_CURVE('',#1894,#1895,#1243,.T.);
#2496=EDGE_CURVE('',#1895,#1896,#360,.T.);
#2497=EDGE_CURVE('',#1896,#1893,#361,.T.);
#2498=EDGE_CURVE('',#1892,#1894,#362,.T.);
#2499=EDGE_CURVE('',#1897,#1898,#1244,.T.);
#2500=EDGE_CURVE('',#1898,#1895,#363,.T.);
#2501=EDGE_CURVE('',#1894,#1897,#364,.T.);
#2502=EDGE_CURVE('',#1899,#1900,#1245,.T.);
#2503=EDGE_CURVE('',#1899,#1901,#365,.T.);
#2504=EDGE_CURVE('',#1901,#1902,#637,.F.);
#2505=EDGE_CURVE('',#1902,#1900,#366,.T.);
#2506=EDGE_CURVE('',#1900,#1903,#367,.T.);
#2507=EDGE_CURVE('',#1903,#1898,#368,.T.);
#2508=EDGE_CURVE('',#1897,#1899,#369,.T.);
#2509=EDGE_CURVE('',#1877,#1904,#370,.T.);
#2510=EDGE_CURVE('',#1904,#1873,#371,.T.);
#2511=EDGE_CURVE('',#1905,#1872,#372,.T.);
#2512=EDGE_CURVE('',#1876,#1905,#373,.T.);
#2513=EDGE_CURVE('',#1854,#1906,#374,.T.);
#2514=EDGE_CURVE('',#1901,#1880,#375,.T.);
#2515=EDGE_CURVE('',#1906,#1885,#376,.T.);
#2516=EDGE_CURVE('',#1884,#1855,#377,.T.);
#2517=EDGE_CURVE('',#1879,#1902,#378,.T.);
#2518=EDGE_CURVE('',#1907,#1908,#1246,.T.);
#2519=EDGE_CURVE('',#1908,#1909,#1247,.T.);
#2520=EDGE_CURVE('',#1909,#1910,#1248,.T.);
#2521=EDGE_CURVE('',#1910,#1911,#1249,.T.);
#2522=EDGE_CURVE('',#1911,#1912,#1250,.T.);
#2523=EDGE_CURVE('',#1912,#1907,#1251,.T.);
#2524=EDGE_CURVE('',#1913,#1914,#1252,.T.);
#2525=EDGE_CURVE('',#1914,#1907,#1253,.T.);
#2526=EDGE_CURVE('',#1913,#1912,#1254,.T.);
#2527=EDGE_CURVE('',#1915,#1913,#1255,.T.);
#2528=EDGE_CURVE('',#1915,#1911,#1256,.T.);
#2529=EDGE_CURVE('',#1916,#1915,#1257,.T.);
#2530=EDGE_CURVE('',#1916,#1910,#1258,.T.);
#2531=EDGE_CURVE('',#1917,#1916,#1259,.T.);
#2532=EDGE_CURVE('',#1917,#1909,#1260,.T.);
#2533=EDGE_CURVE('',#1918,#1917,#1261,.T.);
#2534=EDGE_CURVE('',#1918,#1908,#1262,.T.);
#2535=EDGE_CURVE('',#1914,#1918,#1263,.T.);
#3588=ORIENTED_EDGE('',*,*,#2445,.T.);
#3589=ORIENTED_EDGE('',*,*,#2446,.T.);
#3590=ORIENTED_EDGE('',*,*,#2447,.F.);
#3591=ORIENTED_EDGE('',*,*,#2448,.F.);
#3592=ORIENTED_EDGE('',*,*,#2449,.T.);
#3593=ORIENTED_EDGE('',*,*,#2450,.T.);
#3594=ORIENTED_EDGE('',*,*,#2451,.T.);
#3595=ORIENTED_EDGE('',*,*,#2445,.F.);
#3596=ORIENTED_EDGE('',*,*,#2452,.F.);
#3597=ORIENTED_EDGE('',*,*,#2453,.F.);
#3598=ORIENTED_EDGE('',*,*,#2454,.T.);
#3599=ORIENTED_EDGE('',*,*,#2455,.T.);
#3600=ORIENTED_EDGE('',*,*,#2456,.T.);
#3601=ORIENTED_EDGE('',*,*,#2449,.F.);
#3602=ORIENTED_EDGE('',*,*,#2457,.F.);
#3603=ORIENTED_EDGE('',*,*,#2458,.F.);
#3604=ORIENTED_EDGE('',*,*,#2459,.T.);
#3605=ORIENTED_EDGE('',*,*,#2460,.T.);
#3606=ORIENTED_EDGE('',*,*,#2461,.T.);
#3607=ORIENTED_EDGE('',*,*,#2454,.F.);
#3608=ORIENTED_EDGE('',*,*,#2462,.F.);
#3609=ORIENTED_EDGE('',*,*,#2463,.F.);
#3610=ORIENTED_EDGE('',*,*,#2464,.T.);
#3611=ORIENTED_EDGE('',*,*,#2465,.T.);
#3612=ORIENTED_EDGE('',*,*,#2466,.T.);
#3613=ORIENTED_EDGE('',*,*,#2459,.F.);
#3614=ORIENTED_EDGE('',*,*,#2467,.F.);
#3615=ORIENTED_EDGE('',*,*,#2468,.F.);
#3616=ORIENTED_EDGE('',*,*,#2469,.T.);
#3617=ORIENTED_EDGE('',*,*,#2470,.T.);
#3618=ORIENTED_EDGE('',*,*,#2471,.T.);
#3619=ORIENTED_EDGE('',*,*,#2464,.F.);
#3620=ORIENTED_EDGE('',*,*,#2472,.F.);
#3621=ORIENTED_EDGE('',*,*,#2473,.F.);
#3622=ORIENTED_EDGE('',*,*,#2474,.F.);
#3623=ORIENTED_EDGE('',*,*,#2475,.F.);
#3624=ORIENTED_EDGE('',*,*,#2476,.F.);
#3625=ORIENTED_EDGE('',*,*,#2477,.F.);
#3626=ORIENTED_EDGE('',*,*,#2478,.T.);
#3627=ORIENTED_EDGE('',*,*,#2479,.T.);
#3628=ORIENTED_EDGE('',*,*,#2480,.T.);
#3629=ORIENTED_EDGE('',*,*,#2481,.T.);
#3630=ORIENTED_EDGE('',*,*,#2482,.F.);
#3631=ORIENTED_EDGE('',*,*,#2483,.T.);
#3632=ORIENTED_EDGE('',*,*,#2484,.T.);
#3633=ORIENTED_EDGE('',*,*,#2485,.T.);
#3634=ORIENTED_EDGE('',*,*,#2486,.T.);
#3635=ORIENTED_EDGE('',*,*,#2480,.F.);
#3636=ORIENTED_EDGE('',*,*,#2487,.T.);
#3637=ORIENTED_EDGE('',*,*,#2488,.T.);
#3638=ORIENTED_EDGE('',*,*,#2489,.T.);
#3639=ORIENTED_EDGE('',*,*,#2490,.T.);
#3640=ORIENTED_EDGE('',*,*,#2484,.F.);
#3641=ORIENTED_EDGE('',*,*,#2491,.T.);
#3642=ORIENTED_EDGE('',*,*,#2492,.T.);
#3643=ORIENTED_EDGE('',*,*,#2493,.T.);
#3644=ORIENTED_EDGE('',*,*,#2488,.F.);
#3645=ORIENTED_EDGE('',*,*,#2494,.T.);
#3646=ORIENTED_EDGE('',*,*,#2495,.T.);
#3647=ORIENTED_EDGE('',*,*,#2496,.T.);
#3648=ORIENTED_EDGE('',*,*,#2497,.T.);
#3649=ORIENTED_EDGE('',*,*,#2492,.F.);
#3650=ORIENTED_EDGE('',*,*,#2498,.T.);
#3651=ORIENTED_EDGE('',*,*,#2499,.T.);
#3652=ORIENTED_EDGE('',*,*,#2500,.T.);
#3653=ORIENTED_EDGE('',*,*,#2495,.F.);
#3654=ORIENTED_EDGE('',*,*,#2501,.T.);
#3655=ORIENTED_EDGE('',*,*,#2502,.F.);
#3656=ORIENTED_EDGE('',*,*,#2503,.T.);
#3657=ORIENTED_EDGE('',*,*,#2504,.T.);
#3658=ORIENTED_EDGE('',*,*,#2505,.T.);
#3659=ORIENTED_EDGE('',*,*,#2502,.T.);
#3660=ORIENTED_EDGE('',*,*,#2506,.T.);
#3661=ORIENTED_EDGE('',*,*,#2507,.T.);
#3662=ORIENTED_EDGE('',*,*,#2499,.F.);
#3663=ORIENTED_EDGE('',*,*,#2508,.T.);
#3664=ORIENTED_EDGE('',*,*,#2474,.T.);
#3665=ORIENTED_EDGE('',*,*,#2509,.T.);
#3666=ORIENTED_EDGE('',*,*,#2510,.T.);
#3667=ORIENTED_EDGE('',*,*,#2469,.F.);
#3668=ORIENTED_EDGE('',*,*,#2511,.F.);
#3669=ORIENTED_EDGE('',*,*,#2512,.F.);
#3670=ORIENTED_EDGE('',*,*,#2513,.F.);
#3671=ORIENTED_EDGE('',*,*,#2446,.F.);
#3672=ORIENTED_EDGE('',*,*,#2451,.F.);
#3673=ORIENTED_EDGE('',*,*,#2450,.F.);
#3674=ORIENTED_EDGE('',*,*,#2456,.F.);
#3675=ORIENTED_EDGE('',*,*,#2455,.F.);
#3676=ORIENTED_EDGE('',*,*,#2461,.F.);
#3677=ORIENTED_EDGE('',*,*,#2460,.F.);
#3678=ORIENTED_EDGE('',*,*,#2466,.F.);
#3679=ORIENTED_EDGE('',*,*,#2465,.F.);
#3680=ORIENTED_EDGE('',*,*,#2471,.F.);
#3681=ORIENTED_EDGE('',*,*,#2470,.F.);
#3682=ORIENTED_EDGE('',*,*,#2510,.F.);
#3683=ORIENTED_EDGE('',*,*,#2509,.F.);
#3684=ORIENTED_EDGE('',*,*,#2479,.F.);
#3685=ORIENTED_EDGE('',*,*,#2478,.F.);
#3686=ORIENTED_EDGE('',*,*,#2514,.F.);
#3687=ORIENTED_EDGE('',*,*,#2503,.F.);
#3688=ORIENTED_EDGE('',*,*,#2508,.F.);
#3689=ORIENTED_EDGE('',*,*,#2501,.F.);
#3690=ORIENTED_EDGE('',*,*,#2498,.F.);
#3691=ORIENTED_EDGE('',*,*,#2494,.F.);
#3692=ORIENTED_EDGE('',*,*,#2491,.F.);
#3693=ORIENTED_EDGE('',*,*,#2487,.F.);
#3694=ORIENTED_EDGE('',*,*,#2483,.F.);
#3695=ORIENTED_EDGE('',*,*,#2515,.F.);
#3696=ORIENTED_EDGE('',*,*,#2516,.F.);
#3697=ORIENTED_EDGE('',*,*,#2481,.F.);
#3698=ORIENTED_EDGE('',*,*,#2486,.F.);
#3699=ORIENTED_EDGE('',*,*,#2485,.F.);
#3700=ORIENTED_EDGE('',*,*,#2490,.F.);
#3701=ORIENTED_EDGE('',*,*,#2489,.F.);
#3702=ORIENTED_EDGE('',*,*,#2493,.F.);
#3703=ORIENTED_EDGE('',*,*,#2497,.F.);
#3704=ORIENTED_EDGE('',*,*,#2496,.F.);
#3705=ORIENTED_EDGE('',*,*,#2500,.F.);
#3706=ORIENTED_EDGE('',*,*,#2507,.F.);
#3707=ORIENTED_EDGE('',*,*,#2506,.F.);
#3708=ORIENTED_EDGE('',*,*,#2505,.F.);
#3709=ORIENTED_EDGE('',*,*,#2517,.F.);
#3710=ORIENTED_EDGE('',*,*,#2476,.T.);
#3711=ORIENTED_EDGE('',*,*,#2475,.T.);
#3712=ORIENTED_EDGE('',*,*,#2512,.T.);
#3713=ORIENTED_EDGE('',*,*,#2511,.T.);
#3714=ORIENTED_EDGE('',*,*,#2473,.T.);
#3715=ORIENTED_EDGE('',*,*,#2472,.T.);
#3716=ORIENTED_EDGE('',*,*,#2468,.T.);
#3717=ORIENTED_EDGE('',*,*,#2467,.T.);
#3718=ORIENTED_EDGE('',*,*,#2463,.T.);
#3719=ORIENTED_EDGE('',*,*,#2462,.T.);
#3720=ORIENTED_EDGE('',*,*,#2458,.T.);
#3721=ORIENTED_EDGE('',*,*,#2457,.T.);
#3722=ORIENTED_EDGE('',*,*,#2453,.T.);
#3723=ORIENTED_EDGE('',*,*,#2452,.T.);
#3724=ORIENTED_EDGE('',*,*,#2448,.T.);
#3725=ORIENTED_EDGE('',*,*,#2518,.T.);
#3726=ORIENTED_EDGE('',*,*,#2519,.T.);
#3727=ORIENTED_EDGE('',*,*,#2520,.T.);
#3728=ORIENTED_EDGE('',*,*,#2521,.T.);
#3729=ORIENTED_EDGE('',*,*,#2522,.T.);
#3730=ORIENTED_EDGE('',*,*,#2523,.T.);
#3731=ORIENTED_EDGE('',*,*,#2516,.T.);
#3732=ORIENTED_EDGE('',*,*,#2447,.T.);
#3733=ORIENTED_EDGE('',*,*,#2513,.T.);
#3734=ORIENTED_EDGE('',*,*,#2515,.T.);
#3735=ORIENTED_EDGE('',*,*,#2482,.T.);
#3736=ORIENTED_EDGE('',*,*,#2524,.T.);
#3737=ORIENTED_EDGE('',*,*,#2525,.T.);
#3738=ORIENTED_EDGE('',*,*,#2523,.F.);
#3739=ORIENTED_EDGE('',*,*,#2526,.F.);
#3740=ORIENTED_EDGE('',*,*,#2527,.T.);
#3741=ORIENTED_EDGE('',*,*,#2526,.T.);
#3742=ORIENTED_EDGE('',*,*,#2522,.F.);
#3743=ORIENTED_EDGE('',*,*,#2528,.F.);
#3744=ORIENTED_EDGE('',*,*,#2529,.T.);
#3745=ORIENTED_EDGE('',*,*,#2528,.T.);
#3746=ORIENTED_EDGE('',*,*,#2521,.F.);
#3747=ORIENTED_EDGE('',*,*,#2530,.F.);
#3748=ORIENTED_EDGE('',*,*,#2531,.T.);
#3749=ORIENTED_EDGE('',*,*,#2530,.T.);
#3750=ORIENTED_EDGE('',*,*,#2520,.F.);
#3751=ORIENTED_EDGE('',*,*,#2532,.F.);
#3752=ORIENTED_EDGE('',*,*,#2533,.T.);
#3753=ORIENTED_EDGE('',*,*,#2532,.T.);
#3754=ORIENTED_EDGE('',*,*,#2519,.F.);
#3755=ORIENTED_EDGE('',*,*,#2534,.F.);
#3756=ORIENTED_EDGE('',*,*,#2535,.T.);
#3757=ORIENTED_EDGE('',*,*,#2534,.T.);
#3758=ORIENTED_EDGE('',*,*,#2518,.F.);
#3759=ORIENTED_EDGE('',*,*,#2525,.F.);
#3760=ORIENTED_EDGE('',*,*,#2535,.F.);
#3761=ORIENTED_EDGE('',*,*,#2524,.F.);
#3762=ORIENTED_EDGE('',*,*,#2527,.F.);
#3763=ORIENTED_EDGE('',*,*,#2529,.F.);
#3764=ORIENTED_EDGE('',*,*,#2531,.F.);
#3765=ORIENTED_EDGE('',*,*,#2533,.F.);
#3766=ORIENTED_EDGE('',*,*,#2517,.T.);
#3767=ORIENTED_EDGE('',*,*,#2504,.F.);
#3768=ORIENTED_EDGE('',*,*,#2514,.T.);
#3769=ORIENTED_EDGE('',*,*,#2477,.T.);
#3826=PLANE('',#4451);
#3827=PLANE('',#4452);
#3828=PLANE('',#4453);
#3829=PLANE('',#4454);
#3830=PLANE('',#4455);
#3831=PLANE('',#4456);
#3832=PLANE('',#4457);
#3833=PLANE('',#4458);
#4006=ADVANCED_FACE('',(#810),#484,.F.);
#4007=ADVANCED_FACE('',(#811),#485,.F.);
#4008=ADVANCED_FACE('',(#812),#486,.F.);
#4009=ADVANCED_FACE('',(#813),#487,.F.);
#4010=ADVANCED_FACE('',(#814),#488,.F.);
#4011=ADVANCED_FACE('',(#815),#489,.F.);
#4012=ADVANCED_FACE('',(#816),#490,.F.);
#4013=ADVANCED_FACE('',(#817),#491,.F.);
#4014=ADVANCED_FACE('',(#818),#492,.F.);
#4015=ADVANCED_FACE('',(#819),#493,.F.);
#4016=ADVANCED_FACE('',(#820),#494,.F.);
#4017=ADVANCED_FACE('',(#821),#495,.F.);
#4018=ADVANCED_FACE('',(#822),#496,.F.);
#4019=ADVANCED_FACE('',(#823),#497,.F.);
#4020=ADVANCED_FACE('',(#824),#498,.F.);
#4021=ADVANCED_FACE('',(#825),#499,.F.);
#4022=ADVANCED_FACE('',(#826),#92,.F.);
#4023=ADVANCED_FACE('',(#827),#93,.F.);
#4024=ADVANCED_FACE('',(#828,#394),#3826,.T.);
#4025=ADVANCED_FACE('',(#829),#3827,.T.);
#4026=ADVANCED_FACE('',(#830),#3828,.T.);
#4027=ADVANCED_FACE('',(#831),#3829,.T.);
#4028=ADVANCED_FACE('',(#832),#3830,.T.);
#4029=ADVANCED_FACE('',(#833),#3831,.T.);
#4030=ADVANCED_FACE('',(#834),#3832,.T.);
#4031=ADVANCED_FACE('',(#835,#395),#3833,.F.);
#4040=CLOSED_SHELL('',(#4006,#4007,#4008,#4009,#4010,#4011,#4012,#4013,
#4014,#4015,#4016,#4017,#4018,#4019,#4020,#4021,#4022,#4023,#4024,#4025,
#4026,#4027,#4028,#4029,#4030,#4031));
#4430=AXIS2_PLACEMENT_3D('',#36917,#5227,#5228);
#4431=AXIS2_PLACEMENT_3D('',#36918,#5229,#5230);
#4432=AXIS2_PLACEMENT_3D('',#36928,#5232,#5233);
#4433=AXIS2_PLACEMENT_3D('',#36934,#5234,#5235);
#4434=AXIS2_PLACEMENT_3D('',#37303,#5237,#5238);
#4435=AXIS2_PLACEMENT_3D('',#37850,#5240,#5241);
#4436=AXIS2_PLACEMENT_3D('',#38238,#5243,#5244);
#4437=AXIS2_PLACEMENT_3D('',#38699,#5246,#5247);
#4438=AXIS2_PLACEMENT_3D('',#39249,#5249,#5250);
#4439=AXIS2_PLACEMENT_3D('',#39271,#5252,#5253);
#4440=AXIS2_PLACEMENT_3D('',#39452,#5254,#5255);
#4441=AXIS2_PLACEMENT_3D('',#39528,#5257,#5258);
#4442=AXIS2_PLACEMENT_3D('',#39581,#5259,#5260);
#4443=AXIS2_PLACEMENT_3D('',#39840,#5262,#5263);
#4444=AXIS2_PLACEMENT_3D('',#39996,#5265,#5266);
#4445=AXIS2_PLACEMENT_3D('',#40200,#5268,#5269);
#4446=AXIS2_PLACEMENT_3D('',#40399,#5271,#5272);
#4447=AXIS2_PLACEMENT_3D('',#40595,#5274,#5275);
#4448=AXIS2_PLACEMENT_3D('',#40615,#5277,#5278);
#4449=AXIS2_PLACEMENT_3D('',#40728,#5279,#5280);
#4450=AXIS2_PLACEMENT_3D('',#41007,#5281,#5282);
#4451=AXIS2_PLACEMENT_3D('',#42599,#5283,#5284);
#4452=AXIS2_PLACEMENT_3D('',#42612,#5291,#5292);
#4453=AXIS2_PLACEMENT_3D('',#42618,#5296,#5297);
#4454=AXIS2_PLACEMENT_3D('',#42622,#5300,#5301);
#4455=AXIS2_PLACEMENT_3D('',#42626,#5304,#5305);
#4456=AXIS2_PLACEMENT_3D('',#42630,#5308,#5309);
#4457=AXIS2_PLACEMENT_3D('',#42634,#5312,#5313);
#4458=AXIS2_PLACEMENT_3D('',#42636,#5315,#5316);
#5227=DIRECTION('axis',(0.,0.,1.));
#5228=DIRECTION('refdir',(1.,0.,0.));
#5229=DIRECTION('center_axis',(0.,-1.,0.));
#5230=DIRECTION('ref_axis',(-0.608872791442031,0.,0.793267876471491));
#5231=DIRECTION('',(0.,-1.,0.));
#5232=DIRECTION('center_axis',(0.,1.,0.));
#5233=DIRECTION('ref_axis',(1.,0.,1.81309624337467E-14));
#5234=DIRECTION('center_axis',(0.,-1.,0.));
#5235=DIRECTION('ref_axis',(-0.608872791442031,0.,0.793267876471491));
#5236=DIRECTION('',(0.,-1.,0.));
#5237=DIRECTION('center_axis',(0.,-1.,0.));
#5238=DIRECTION('ref_axis',(-0.608872791442031,0.,0.793267876471491));
#5239=DIRECTION('',(0.,-1.,0.));
#5240=DIRECTION('center_axis',(0.,-1.,0.));
#5241=DIRECTION('ref_axis',(-0.608872791442031,0.,0.793267876471491));
#5242=DIRECTION('',(0.,-1.,0.));
#5243=DIRECTION('center_axis',(0.,-1.,0.));
#5244=DIRECTION('ref_axis',(-0.608872791442031,0.,0.793267876471491));
#5245=DIRECTION('',(0.,-1.,0.));
#5246=DIRECTION('center_axis',(0.,-1.,0.));
#5247=DIRECTION('ref_axis',(-0.608872791442031,0.,0.793267876471491));
#5248=DIRECTION('',(0.,-1.,0.));
#5249=DIRECTION('center_axis',(0.,-1.,0.));
#5250=DIRECTION('ref_axis',(-0.608872791442031,0.,0.793267876471491));
#5251=DIRECTION('',(0.,-1.,0.));
#5252=DIRECTION('center_axis',(0.,-1.,0.));
#5253=DIRECTION('ref_axis',(1.,0.,1.81309624337467E-14));
#5254=DIRECTION('center_axis',(0.,-1.,0.));
#5255=DIRECTION('ref_axis',(-0.986183607793452,0.,-0.165655943809726));
#5256=DIRECTION('',(0.,-1.,0.));
#5257=DIRECTION('center_axis',(0.,-1.,0.));
#5258=DIRECTION('ref_axis',(1.,0.,0.));
#5259=DIRECTION('center_axis',(0.,-1.,0.));
#5260=DIRECTION('ref_axis',(-0.986183607793452,0.,-0.165655943809726));
#5261=DIRECTION('',(0.,-1.,0.));
#5262=DIRECTION('center_axis',(0.,-1.,0.));
#5263=DIRECTION('ref_axis',(-0.986183607793452,0.,-0.165655943809726));
#5264=DIRECTION('',(0.,-1.,0.));
#5265=DIRECTION('center_axis',(0.,-1.,0.));
#5266=DIRECTION('ref_axis',(-0.986183607793452,0.,-0.165655943809726));
#5267=DIRECTION('',(0.,-1.,0.));
#5268=DIRECTION('center_axis',(0.,-1.,0.));
#5269=DIRECTION('ref_axis',(-0.986183607793452,0.,-0.165655943809726));
#5270=DIRECTION('',(0.,-1.,0.));
#5271=DIRECTION('center_axis',(0.,-1.,0.));
#5272=DIRECTION('ref_axis',(-0.986183607793452,0.,-0.165655943809726));
#5273=DIRECTION('',(0.,-1.,0.));
#5274=DIRECTION('center_axis',(0.,-1.,0.));
#5275=DIRECTION('ref_axis',(-0.986183607793452,0.,-0.165655943809726));
#5276=DIRECTION('',(0.,-1.,0.));
#5277=DIRECTION('center_axis',(0.,-1.,0.));
#5278=DIRECTION('ref_axis',(1.,0.,0.));
#5279=DIRECTION('center_axis',(0.,-1.,0.));
#5280=DIRECTION('ref_axis',(-0.986183607793452,0.,-0.165655943809726));
#5281=DIRECTION('center_axis',(0.,-1.,0.));
#5282=DIRECTION('ref_axis',(-0.608872791442031,0.,0.793267876471491));
#5283=DIRECTION('center_axis',(0.,-1.,0.));
#5284=DIRECTION('ref_axis',(1.,0.,0.));
#5285=DIRECTION('',(-1.,0.,4.69353744302978E-16));
#5286=DIRECTION('',(-0.5,0.,-0.866025403784439));
#5287=DIRECTION('',(0.5,0.,-0.866025403784439));
#5288=DIRECTION('',(1.,0.,-4.69353744302978E-16));
#5289=DIRECTION('',(0.500000000000001,0.,0.866025403784438));
#5290=DIRECTION('',(-0.499999999999999,0.,0.866025403784439));
#5291=DIRECTION('center_axis',(0.866025403784439,0.,0.499999999999999));
#5292=DIRECTION('ref_axis',(-0.499999999999999,0.,0.866025403784439));
#5293=DIRECTION('',(-0.499999999999999,0.,0.866025403784439));
#5294=DIRECTION('',(0.,-1.,0.));
#5295=DIRECTION('',(0.,-1.,0.));
#5296=DIRECTION('center_axis',(0.866025403784438,0.,-0.500000000000001));
#5297=DIRECTION('ref_axis',(0.500000000000001,0.,0.866025403784438));
#5298=DIRECTION('',(0.500000000000001,0.,0.866025403784438));
#5299=DIRECTION('',(0.,-1.,0.));
#5300=DIRECTION('center_axis',(-4.69353744302978E-16,0.,-1.));
#5301=DIRECTION('ref_axis',(1.,0.,-4.69353744302978E-16));
#5302=DIRECTION('',(1.,0.,-4.69353744302978E-16));
#5303=DIRECTION('',(0.,-1.,0.));
#5304=DIRECTION('center_axis',(-0.866025403784439,0.,-0.5));
#5305=DIRECTION('ref_axis',(0.5,0.,-0.866025403784439));
#5306=DIRECTION('',(0.5,0.,-0.866025403784439));
#5307=DIRECTION('',(0.,-1.,0.));
#5308=DIRECTION('center_axis',(-0.866025403784439,0.,0.5));
#5309=DIRECTION('ref_axis',(-0.5,0.,-0.866025403784439));
#5310=DIRECTION('',(-0.5,0.,-0.866025403784439));
#5311=DIRECTION('',(0.,-1.,0.));
#5312=DIRECTION('center_axis',(4.69353744302978E-16,0.,1.));
#5313=DIRECTION('ref_axis',(-1.,0.,4.69353744302978E-16));
#5314=DIRECTION('',(-1.,0.,4.69353744302978E-16));
#5315=DIRECTION('center_axis',(0.,-1.,0.));
#5316=DIRECTION('ref_axis',(1.,0.,0.));
#36917=CARTESIAN_POINT('',(0.,0.,0.));
#36918=CARTESIAN_POINT('Origin',(0.,-13.3748739960349,0.));
#36919=CARTESIAN_POINT('',(7.41225940988737,-39.6876842086708,-9.65703625032018));
#36920=CARTESIAN_POINT('',(7.4120723883382,-39.9374428050303,-9.6567920162102));
#36921=CARTESIAN_POINT('',(7.41272179941101,-13.3748739960349,-9.65763976210217));
#36922=CARTESIAN_POINT('',(8.61094305413662,-40.,-8.60639936142963));
#36923=CARTESIAN_POINT('Ctrl Pts',(7.4120723883382,-39.9374428050303,-9.6567920162102));
#36924=CARTESIAN_POINT('Ctrl Pts',(7.83414093874789,-39.9582952033535,-9.33338243380816));
#36925=CARTESIAN_POINT('Ctrl Pts',(8.23507438987139,-39.9791476016768,-8.98246646311764));
#36926=CARTESIAN_POINT('Ctrl Pts',(8.61094305413662,-40.,-8.60639936142963));
#36927=CARTESIAN_POINT('',(11.7598063682261,-40.,-3.15424737243508));
#36928=CARTESIAN_POINT('Origin',(0.,-40.,0.));
#36929=CARTESIAN_POINT('Ctrl Pts',(7.41225940988737,-39.6876842086708,-9.65703625032018));
#36930=CARTESIAN_POINT('Ctrl Pts',(8.0009299948616,-39.7167676583016,-9.20584367320952));
#36931=CARTESIAN_POINT('Ctrl Pts',(9.96140840545013,-39.820872922078,-7.4001799654877));
#36932=CARTESIAN_POINT('Ctrl Pts',(11.263434788298,-39.9249781858544,-5.00116413859683));
#36933=CARTESIAN_POINT('Ctrl Pts',(11.7598063682261,-40.,-3.15424737243508));
#36934=CARTESIAN_POINT('Origin',(0.,-13.3748739960349,0.));
#36935=CARTESIAN_POINT('',(7.41272179941099,-36.6876961535581,-9.65763976210219));
#36936=CARTESIAN_POINT('',(7.41272179941099,-36.9374484774433,-9.65763976210219));
#36937=CARTESIAN_POINT('',(7.41272179941101,-13.3748739960349,-9.65763976210217));
#36938=CARTESIAN_POINT('',(-12.1744916248676,-38.8748739948544,0.000309104184771874));
#36939=CARTESIAN_POINT('Ctrl Pts',(7.41272179941099,-36.9374484774433,-9.65763976210219));
#36940=CARTESIAN_POINT('Ctrl Pts',(7.63813777186494,-36.9485938361832,-9.48462172310865));
#36941=CARTESIAN_POINT('Ctrl Pts',(7.85751736927417,-36.959739194923,-9.3036899163584));
#36942=CARTESIAN_POINT('Ctrl Pts',(8.07031067017878,-36.9708845536629,-9.11529132484523));
#36943=CARTESIAN_POINT('Ctrl Pts',(8.28308082857198,-36.98202870028,-8.92691322277667));
#36944=CARTESIAN_POINT('Ctrl Pts',(8.48926592113985,-36.9931728468971,-8.73107013428625));
#36945=CARTESIAN_POINT('Ctrl Pts',(8.68835034828689,-37.0043169935143,-8.5282482653487));
#36946=CARTESIAN_POINT('Ctrl Pts',(8.89179157179527,-37.0157050204697,-8.3209878092587));
#36947=CARTESIAN_POINT('Ctrl Pts',(9.08781759960384,-37.027093047425,-8.10643984428187));
#36948=CARTESIAN_POINT('Ctrl Pts',(9.27591824460373,-37.0384810743804,-7.88516271039651));
#36949=CARTESIAN_POINT('Ctrl Pts',(9.46000106079451,-37.0496258531386,-7.66861205495211));
#36950=CARTESIAN_POINT('Ctrl Pts',(9.63649341936148,-37.0607706318969,-7.44561696503954));
#36951=CARTESIAN_POINT('Ctrl Pts',(9.80495738553523,-37.0719154106551,-7.21673478228473));
#36952=CARTESIAN_POINT('Ctrl Pts',(9.9789367446495,-37.083425061709,-6.98035915625153));
#36953=CARTESIAN_POINT('Ctrl Pts',(10.1443529947712,-37.094934712763,-6.73770471196109));
#36954=CARTESIAN_POINT('Ctrl Pts',(10.3007711278883,-37.106444363817,-6.48941942093926));
#36955=CARTESIAN_POINT('Ctrl Pts',(10.4571892610053,-37.1179540148709,-6.24113412991742));
#36956=CARTESIAN_POINT('Ctrl Pts',(10.6046091172304,-37.1294636659249,-5.98721826140925));
#36957=CARTESIAN_POINT('Ctrl Pts',(10.742646351938,-37.1409733169788,-5.72835051364639));
#36958=CARTESIAN_POINT('Ctrl Pts',(10.8763379661845,-37.1521206268483,-5.47763231324153));
#36959=CARTESIAN_POINT('Ctrl Pts',(11.0012686005856,-37.1632679367179,-5.22219436487314));
#36960=CARTESIAN_POINT('Ctrl Pts',(11.1171200677777,-37.1744152465874,-4.9626698105571));
#36961=CARTESIAN_POINT('Ctrl Pts',(11.2329518581578,-37.1855606631402,-4.70318933523264));
#36962=CARTESIAN_POINT('Ctrl Pts',(11.3397074513444,-37.196706079693,-4.43962388319863));
#36963=CARTESIAN_POINT('Ctrl Pts',(11.4371160292913,-37.2078514962458,-4.17262833026484));
#36964=CARTESIAN_POINT('Ctrl Pts',(11.5345137937413,-37.2189956755263,-3.90566241697496));
#36965=CARTESIAN_POINT('Ctrl Pts',(11.6225665235307,-37.2301398548069,-3.63526741367178));
#36966=CARTESIAN_POINT('Ctrl Pts',(11.7010522555776,-37.2412840340875,-3.3621163516812));
#36967=CARTESIAN_POINT('Ctrl Pts',(11.782009616388,-37.2527791596272,-3.08036336926517));
#36968=CARTESIAN_POINT('Ctrl Pts',(11.8527875672035,-37.2642742851669,-2.79567821335521));
#36969=CARTESIAN_POINT('Ctrl Pts',(11.9131983041429,-37.2757694107066,-2.50881573977965));
#36970=CARTESIAN_POINT('Ctrl Pts',(11.971767831112,-37.2869141856162,-2.23069631542371));
#36971=CARTESIAN_POINT('Ctrl Pts',(12.0205926768578,-37.2980589605257,-1.95053060259384));
#36972=CARTESIAN_POINT('Ctrl Pts',(12.0595535357516,-37.3092037354353,-1.6690173061836));
#36973=CARTESIAN_POINT('Ctrl Pts',(12.1003515732662,-37.3208740362901,-1.37422939970866));
#36974=CARTESIAN_POINT('Ctrl Pts',(12.1303329348627,-37.3325443371448,-1.07796407739402));
#36975=CARTESIAN_POINT('Ctrl Pts',(12.1494213968046,-37.3442146379996,-0.781031352038081));
#36976=CARTESIAN_POINT('Ctrl Pts',(12.1685098587465,-37.3558849388544,-0.484098626682174));
#36977=CARTESIAN_POINT('Ctrl Pts',(12.1767054082705,-37.3675552397091,-0.186498833656002));
#36978=CARTESIAN_POINT('Ctrl Pts',(12.1739943825377,-37.3792255405639,0.110955053691345));
#36979=CARTESIAN_POINT('Ctrl Pts',(12.1714048572777,-37.3903728116839,0.395077902726157));
#36980=CARTESIAN_POINT('Ctrl Pts',(12.1588640971083,-37.4015200828038,0.679152499465869));
#36981=CARTESIAN_POINT('Ctrl Pts',(12.1363956968827,-37.4126673539238,0.962470643026071));
#36982=CARTESIAN_POINT('Ctrl Pts',(12.1139311132748,-37.4238127315012,1.24574066046157));
#36983=CARTESIAN_POINT('Ctrl Pts',(12.0815422775253,-37.4349581090787,1.52825421544422));
#36984=CARTESIAN_POINT('Ctrl Pts',(12.0393047783483,-37.4461034866561,1.80930669153689));
#36985=CARTESIAN_POINT('Ctrl Pts',(11.9970719685101,-37.4572476268389,2.09032796430773));
#36986=CARTESIAN_POINT('Ctrl Pts',(11.9449927182814,-37.4683917670218,2.36988821838241));
#36987=CARTESIAN_POINT('Ctrl Pts',(11.8831942023772,-37.4795359072047,2.64729027471258));
#36988=CARTESIAN_POINT('Ctrl Pts',(11.8194491765883,-37.49103106195,2.93342985227278));
#36989=CARTESIAN_POINT('Ctrl Pts',(11.7453627483409,-37.5025262166954,3.21727278043161));
#36990=CARTESIAN_POINT('Ctrl Pts',(11.6611312464288,-37.5140213714408,3.49806636637472));
#36991=CARTESIAN_POINT('Ctrl Pts',(11.5794674609318,-37.525166107437,3.77030022960688));
#36992=CARTESIAN_POINT('Ctrl Pts',(11.4882680468647,-37.5363108434333,4.0396676423719));
#36993=CARTESIAN_POINT('Ctrl Pts',(11.387762605013,-37.5474555794296,4.30549800857771));
#36994=CARTESIAN_POINT('Ctrl Pts',(11.282516944386,-37.5591259435495,4.58386594558306));
#36995=CARTESIAN_POINT('Ctrl Pts',(11.1670664275532,-37.5707963076694,4.85835486815289));
#36996=CARTESIAN_POINT('Ctrl Pts',(11.0417317581506,-37.5824666717893,5.12821704211602));
#36997=CARTESIAN_POINT('Ctrl Pts',(10.916397088748,-37.5941370359092,5.39807921607914));
#36998=CARTESIAN_POINT('Ctrl Pts',(10.7811784160682,-37.6058074000291,5.66331434083362));
#36999=CARTESIAN_POINT('Ctrl Pts',(10.6364527948914,-37.617477764149,5.92320202188377));
#37000=CARTESIAN_POINT('Ctrl Pts',(10.4982123241924,-37.6286251796242,6.171444144219));
#37001=CARTESIAN_POINT('Ctrl Pts',(10.3512569086563,-37.6397725950994,6.41488166047602));
#37002=CARTESIAN_POINT('Ctrl Pts',(10.1959461834747,-37.6509200105746,6.65290400304169));
#37003=CARTESIAN_POINT('Ctrl Pts',(10.0406618319041,-37.6620655330859,6.89088592657842));
#37004=CARTESIAN_POINT('Ctrl Pts',(9.87702514909113,-37.6732110555971,7.12345428902473));
#37005=CARTESIAN_POINT('Ctrl Pts',(9.70543970866531,-37.6843565781084,7.35002655175222));
#37006=CARTESIAN_POINT('Ctrl Pts',(9.53387331491804,-37.6955008634215,7.57657366404126));
#37007=CARTESIAN_POINT('Ctrl Pts',(9.35436008645349,-37.7066451487347,7.79712579310562));
#37008=CARTESIAN_POINT('Ctrl Pts',(9.16734533347103,-37.7177894340478,8.0111316171242));
#37009=CARTESIAN_POINT('Ctrl Pts',(8.97444438432209,-37.7292844801883,8.23187316782131));
#37010=CARTESIAN_POINT('Ctrl Pts',(8.77356223729388,-37.7407795263289,8.44564942636426));
#37011=CARTESIAN_POINT('Ctrl Pts',(8.56523145482445,-37.7522745724694,8.65189345607572));
#37012=CARTESIAN_POINT('Ctrl Pts',(8.36324692134804,-37.7634194522824,8.85185480422493));
#37013=CARTESIAN_POINT('Ctrl Pts',(8.15426104066128,-37.7745643320955,9.04473583466629));
#37014=CARTESIAN_POINT('Ctrl Pts',(7.93879633762431,-37.7857092119086,9.23005758160386));
#37015=CARTESIAN_POINT('Ctrl Pts',(7.71317695122263,-37.7973793412128,9.42411339790046));
#37016=CARTESIAN_POINT('Ctrl Pts',(7.48045361358976,-37.8090494705171,9.60988006186248));
#37017=CARTESIAN_POINT('Ctrl Pts',(7.24126569578255,-37.8207195998213,9.78685451884735));
#37018=CARTESIAN_POINT('Ctrl Pts',(7.00207777797537,-37.8323897291256,9.96382897583221));
#37019=CARTESIAN_POINT('Ctrl Pts',(6.75642555486916,-37.8440598584298,10.1320110333703));
#37020=CARTESIAN_POINT('Ctrl Pts',(6.50498479025111,-37.8557299877341,10.2909486019804));
#37021=CARTESIAN_POINT('Ctrl Pts',(6.26481384489021,-37.8668770505095,10.4427624344129));
#37022=CARTESIAN_POINT('Ctrl Pts',(6.01929011209589,-37.8780241132849,10.5861875973639));
#37023=CARTESIAN_POINT('Ctrl Pts',(5.76902151508655,-37.8891711760602,10.7208600871604));
#37024=CARTESIAN_POINT('Ctrl Pts',(5.51879544336716,-37.9003163447423,10.8555096935958));
#37025=CARTESIAN_POINT('Ctrl Pts',(5.26382635192,-37.9114615134244,10.9814094697884));
#37026=CARTESIAN_POINT('Ctrl Pts',(5.0047473324093,-37.9226066821064,11.0982410493169));
#37027=CARTESIAN_POINT('Ctrl Pts',(4.74569707726916,-37.9337506133909,11.215059657564));
#37028=CARTESIAN_POINT('Ctrl Pts',(4.48253804836199,-37.9448945446753,11.3228119699299));
#37029=CARTESIAN_POINT('Ctrl Pts',(4.21592504663252,-37.9560384759598,11.4212270028739));
#37030=CARTESIAN_POINT('Ctrl Pts',(3.94090545364192,-37.9675337872397,11.5227451663875));
#37031=CARTESIAN_POINT('Ctrl Pts',(3.66221081418894,-37.9790290985197,11.6143275567594));
#37032=CARTESIAN_POINT('Ctrl Pts',(3.38058013274304,-37.9905244097996,11.6957311962999));
#37033=CARTESIAN_POINT('Ctrl Pts',(3.10754346510028,-38.0016689394698,11.774650788299));
#37034=CARTESIAN_POINT('Ctrl Pts',(2.83174755468966,-38.0128134691399,11.8440035547903));
#37035=CARTESIAN_POINT('Ctrl Pts',(2.55388037739943,-38.02395799881,11.9036189987724));
#37036=CARTESIAN_POINT('Ctrl Pts',(2.26289411406654,-38.0356287008949,11.9660490973915));
#37037=CARTESIAN_POINT('Ctrl Pts',(1.96963659936645,-38.0472994029797,12.0178001895381));
#37038=CARTESIAN_POINT('Ctrl Pts',(1.67491012193627,-38.0589701050646,12.0587365148027));
#37039=CARTESIAN_POINT('Ctrl Pts',(1.38018364450609,-38.0706408071495,12.0996728400673));
#37040=CARTESIAN_POINT('Ctrl Pts',(1.08398853798748,-38.0823115092343,12.1297943609895));
#37041=CARTESIAN_POINT('Ctrl Pts',(0.787134657080782,-38.0939822113192,
12.1490275035339));
#37042=CARTESIAN_POINT('Ctrl Pts',(0.503583140229768,-38.1051299358117,
12.1673987868252));
#37043=CARTESIAN_POINT('Ctrl Pts',(0.219345890921422,-38.1162776603042,
12.1758415742294));
#37044=CARTESIAN_POINT('Ctrl Pts',(-0.0648690228389137,-38.1274253847967,
12.1743271789399));
#37045=CARTESIAN_POINT('Ctrl Pts',(-0.349035688152791,-38.1385712168467,
12.1728130407349));
#37046=CARTESIAN_POINT('Ctrl Pts',(-0.633179758886583,-38.1497170488967,
12.1613450960154));
#37047=CARTESIAN_POINT('Ctrl Pts',(-0.916592908336909,-38.1608628809466,
12.1399467746109));
#37048=CARTESIAN_POINT('Ctrl Pts',(-1.19997459133722,-38.1720074755108,
12.1185508289933));
#37049=CARTESIAN_POINT('Ctrl Pts',(-1.48262524921969,-38.1831520700749,
12.0872267283601));
#37050=CARTESIAN_POINT('Ctrl Pts',(-1.76384016867791,-38.194296664639,12.0460498965162));
#37051=CARTESIAN_POINT('Ctrl Pts',(-2.05389228566501,-38.2057914788278,
12.0035790799957));
#37052=CARTESIAN_POINT('Ctrl Pts',(-2.34241667380791,-38.2172862930165,
11.9506263064734));
#37053=CARTESIAN_POINT('Ctrl Pts',(-2.62864831310905,-38.2287811072053,
11.8873318409132));
#37054=CARTESIAN_POINT('Ctrl Pts',(-2.90617384669823,-38.2399262917455,
11.8259625584302));
#37055=CARTESIAN_POINT('Ctrl Pts',(-3.18154377189134,-38.2510714762857,
11.7548714598031));
#37056=CARTESIAN_POINT('Ctrl Pts',(-3.45407233157046,-38.2622166608259,
11.6742380727086));
#37057=CARTESIAN_POINT('Ctrl Pts',(-3.73942491370659,-38.2738862898389,
11.5898104250489));
#37058=CARTESIAN_POINT('Ctrl Pts',(-4.02166199993082,-38.285555918852,11.4949209773659));
#37059=CARTESIAN_POINT('Ctrl Pts',(-4.30001441364412,-38.2972255478651,
11.3898343399916));
#37060=CARTESIAN_POINT('Ctrl Pts',(-4.57836682735739,-38.3088951768782,
11.2847477026174));
#37061=CARTESIAN_POINT('Ctrl Pts',(-4.85283425796642,-38.3205648058912,
11.1694640021579));
#37062=CARTESIAN_POINT('Ctrl Pts',(-5.12267062571763,-38.3322344349043,
11.0443060402367));
#37063=CARTESIAN_POINT('Ctrl Pts',(-5.38041794246529,-38.343381248029,10.9247553320664));
#37064=CARTESIAN_POINT('Ctrl Pts',(-5.63401694334377,-38.3545280611537,
10.796160008172));
#37065=CARTESIAN_POINT('Ctrl Pts',(-5.88283226064311,-38.3656748742783,
10.6588336530381));
#37066=CARTESIAN_POINT('Ctrl Pts',(-6.1316053072015,-38.376819793693,10.5215306280063));
#37067=CARTESIAN_POINT('Ctrl Pts',(-6.37559605922401,-38.3879647131077,
10.3754996620031));
#37068=CARTESIAN_POINT('Ctrl Pts',(-6.61419386041611,-38.3991096325224,
10.2211002258482));
#37069=CARTESIAN_POINT('Ctrl Pts',(-6.85276519254124,-38.4102533155651,
10.066717918137));
#37070=CARTESIAN_POINT('Ctrl Pts',(-7.08594454455926,-38.4213969986079,
9.90396913897554));
#37071=CARTESIAN_POINT('Ctrl Pts',(-7.31314931363975,-38.4325406816507,
9.7332572845071));
#37072=CARTESIAN_POINT('Ctrl Pts',(-7.54752711982908,-38.4440361797206,
9.55715591963368));
#37073=CARTESIAN_POINT('Ctrl Pts',(-7.77554672721654,-38.4555316777905,
9.37258068116194));
#37074=CARTESIAN_POINT('Ctrl Pts',(-7.99660336458607,-38.4670271758604,
9.18002096291129));
#37075=CARTESIAN_POINT('Ctrl Pts',(-8.21090626771047,-38.4781714628565,
8.99334433950392));
#37076=CARTESIAN_POINT('Ctrl Pts',(-8.41866514053532,-38.4893157498526,
8.79916406173953));
#37077=CARTESIAN_POINT('Ctrl Pts',(-8.61936384853658,-38.5004600368487,
8.59796586970085));
#37078=CARTESIAN_POINT('Ctrl Pts',(-8.82955005566236,-38.5121311404555,
8.38725656675452));
#37079=CARTESIAN_POINT('Ctrl Pts',(-9.03199227177261,-38.5238022440623,
8.16885006407581));
#37080=CARTESIAN_POINT('Ctrl Pts',(-9.22614151152845,-38.535473347669,7.94334709421989));
#37081=CARTESIAN_POINT('Ctrl Pts',(-9.42029075128428,-38.5471444512758,
7.71784412436397));
#37082=CARTESIAN_POINT('Ctrl Pts',(-9.60614680231032,-38.5588155548826,
7.4852449475224));
#37083=CARTESIAN_POINT('Ctrl Pts',(-9.78320885115772,-38.5704866584894,
7.24619036629795));
#37084=CARTESIAN_POINT('Ctrl Pts',(-9.95232519265855,-38.5816340181642,
7.01786342408272));
#37085=CARTESIAN_POINT('Ctrl Pts',(-10.1134700589456,-38.592781377839,6.78357934184873));
#37086=CARTESIAN_POINT('Ctrl Pts',(-10.2662355845482,-38.6039287375138,
6.54391757073364));
#37087=CARTESIAN_POINT('Ctrl Pts',(-10.4189751284731,-38.6150742012955,
6.30429656022115));
#37088=CARTESIAN_POINT('Ctrl Pts',(-10.5633380336435,-38.6262196650772,
6.05929991170006));
#37089=CARTESIAN_POINT('Ctrl Pts',(-10.6989600913802,-38.6373651288589,
5.80953554193913));
#37090=CARTESIAN_POINT('Ctrl Pts',(-10.8345670610239,-38.6485093526963,
5.55979895872045));
#37091=CARTESIAN_POINT('Ctrl Pts',(-10.9614349977632,-38.6596535765337,
5.30529594776737));
#37092=CARTESIAN_POINT('Ctrl Pts',(-11.0792453455692,-38.6707978003711,
5.04665957071439));
#37093=CARTESIAN_POINT('Ctrl Pts',(-11.20076485087,-38.682292890513,4.77988024973298));
#37094=CARTESIAN_POINT('Ctrl Pts',(-11.3126470548315,-38.693787980655,4.50870334116523));
#37095=CARTESIAN_POINT('Ctrl Pts',(-11.4145951579047,-38.7052830707969,
4.23384785167571));
#37096=CARTESIAN_POINT('Ctrl Pts',(-11.5134367040608,-38.7164278831925,
3.96736774334894));
#37097=CARTESIAN_POINT('Ctrl Pts',(-11.6029405119847,-38.7275726955881,
3.69743018378309));
#37098=CARTESIAN_POINT('Ctrl Pts',(-11.6828857891978,-38.7387175079836,
3.42470873017855));
#37099=CARTESIAN_POINT('Ctrl Pts',(-11.7666000466156,-38.7503877369988,
3.13912995972093));
#37100=CARTESIAN_POINT('Ctrl Pts',(-11.8398327384508,-38.7620579660139,
2.85049879505899));
#37101=CARTESIAN_POINT('Ctrl Pts',(-11.9023893162427,-38.7737281950291,
2.55960520678335));
#37102=CARTESIAN_POINT('Ctrl Pts',(-11.9649458940345,-38.7853984240442,
2.26871161850769));
#37103=CARTESIAN_POINT('Ctrl Pts',(-12.0168262958164,-38.7970686530593,
1.97555593644156));
#37104=CARTESIAN_POINT('Ctrl Pts',(-12.0578974154622,-38.8087388820745,
1.68094026312326));
#37105=CARTESIAN_POINT('Ctrl Pts',(-12.0989059319874,-38.8203913226104,
1.38677366109214));
#37106=CARTESIAN_POINT('Ctrl Pts',(-12.1291472088389,-38.8320437631464,
1.0910923577));
#37107=CARTESIAN_POINT('Ctrl Pts',(-12.1485371754145,-38.8436962036824,
0.794666437929197));
#37108=CARTESIAN_POINT('Ctrl Pts',(-12.1658307293892,-38.8540888007279,
0.530289621029534));
#37109=CARTESIAN_POINT('Ctrl Pts',(-12.1744932675459,-38.8644813977734,
0.265320699870421));
#37110=CARTESIAN_POINT('Ctrl Pts',(-12.174499996076,-38.8748739948188,0.000309105303522327));
#37111=CARTESIAN_POINT('Ctrl Pts',(-12.1742135449704,-38.8748739960349,
0.000309067021438125));
#37112=CARTESIAN_POINT('Ctrl Pts',(-12.1728218038936,-38.9322463659098,
-1.46265402061263));
#37113=CARTESIAN_POINT('Ctrl Pts',(-11.5435367915227,-39.0690361436464,
-4.95189231269601));
#37114=CARTESIAN_POINT('Ctrl Pts',(-8.28522524716096,-39.2852433292447,
-9.61375508410346));
#37115=CARTESIAN_POINT('Ctrl Pts',(-2.67484068581488,-39.5234955528298,
-12.4063460053113));
#37116=CARTESIAN_POINT('Ctrl Pts',(3.04101717371279,-39.7408953780917,-12.1939464673343));
#37117=CARTESIAN_POINT('Ctrl Pts',(6.22667163503174,-39.8788777954918,-10.5651040954537));
#37118=CARTESIAN_POINT('Ctrl Pts',(7.4120723883382,-39.9374428050303,-9.6567920162102));
#37119=CARTESIAN_POINT('',(-12.1744999965607,-38.6251260039651,0.00028938649696687));
#37120=CARTESIAN_POINT('Ctrl Pts',(-12.1748649577908,-38.6251260151384,
0.000289110302658423));
#37121=CARTESIAN_POINT('Ctrl Pts',(-12.1731836483798,-38.6907258978333,
-1.67221371080106));
#37122=CARTESIAN_POINT('Ctrl Pts',(-11.4051697641933,-38.8357431883897,
-5.37100026957135));
#37123=CARTESIAN_POINT('Ctrl Pts',(-7.77755196994913,-39.060177886808,-10.0290176561892));
#37124=CARTESIAN_POINT('Ctrl Pts',(-2.02988957584845,-39.2984301103931,
-12.5280053565324));
#37125=CARTESIAN_POINT('Ctrl Pts',(3.45078694475986,-39.5075988843473,-12.0396942716201));
#37126=CARTESIAN_POINT('Ctrl Pts',(6.39346277427829,-39.6373502504399,-10.4379033282841));
#37127=CARTESIAN_POINT('Ctrl Pts',(7.41225940988737,-39.6876842086708,-9.65703625032018));
#37128=CARTESIAN_POINT('Ctrl Pts',(7.41272179941099,-36.6876961535581,-9.65763976210219));
#37129=CARTESIAN_POINT('Ctrl Pts',(7.6381238842813,-36.6988428223107,-9.48463238252406));
#37130=CARTESIAN_POINT('Ctrl Pts',(7.85749734347105,-36.7099894910634,-9.30370683240145));
#37131=CARTESIAN_POINT('Ctrl Pts',(8.07029112440213,-36.721136159816,-9.11530862984881));
#37132=CARTESIAN_POINT('Ctrl Pts',(8.28305252155186,-36.7322811322254,-8.92693909846396));
#37133=CARTESIAN_POINT('Ctrl Pts',(8.48923604000689,-36.7434261046349,-8.73109936195701));
#37134=CARTESIAN_POINT('Ctrl Pts',(8.68832482272221,-36.7545710770443,-8.52827427003079));
#37135=CARTESIAN_POINT('Ctrl Pts',(8.88739501900923,-36.7657150089871,-8.3254681133453));
#37136=CARTESIAN_POINT('Ctrl Pts',(9.07937161545807,-36.7768589409299,-8.11567809388224));
#37137=CARTESIAN_POINT('Ctrl Pts',(9.26377477876949,-36.7880028728728,-7.89942574483958));
#37138=CARTESIAN_POINT('Ctrl Pts',(9.44819392555212,-36.7991477707357,-7.68315465174105));
#37139=CARTESIAN_POINT('Ctrl Pts',(9.62503815201837,-36.8102926685985,-7.46042031079913));
#37140=CARTESIAN_POINT('Ctrl Pts',(9.7938671124219,-36.8214375664614,-7.23177828989667));
#37141=CARTESIAN_POINT('Ctrl Pts',(9.96269478289764,-36.8325823791724,-7.00313801592018));
#37142=CARTESIAN_POINT('Ctrl Pts',(10.1235071530054,-36.8437271918833,-6.76859036814335));
#37143=CARTESIAN_POINT('Ctrl Pts',(10.2759059800293,-36.8548720045943,-6.52872166197928));
#37144=CARTESIAN_POINT('Ctrl Pts',(10.4283392073848,-36.8660193329758,-6.28879881128406));
#37145=CARTESIAN_POINT('Ctrl Pts',(10.5723549522108,-36.8771666613574,-6.04355272653906));
#37146=CARTESIAN_POINT('Ctrl Pts',(10.7075990492278,-36.888313989739,-5.7935975741309));
#37147=CARTESIAN_POINT('Ctrl Pts',(10.8191926049702,-36.89751195134,-5.58735282963866));
#37148=CARTESIAN_POINT('Ctrl Pts',(10.9248148936261,-36.9067099129411,-5.37790254937361));
#37149=CARTESIAN_POINT('Ctrl Pts',(11.0242906417777,-36.9159078745421,-5.16560413655685));
#37150=CARTESIAN_POINT('Ctrl Pts',(11.144848515391,-36.9270551814265,-4.90831282991919));
#37151=CARTESIAN_POINT('Ctrl Pts',(11.2564132397565,-36.9382024883108,-4.64676077901745));
#37152=CARTESIAN_POINT('Ctrl Pts',(11.3586997682256,-36.9493497951952,-4.38159672098096));
#37153=CARTESIAN_POINT('Ctrl Pts',(11.460968923368,-36.9604952087139,-4.11647770095578));
#37154=CARTESIAN_POINT('Ctrl Pts',(11.5539629329279,-36.9716406222325,-3.8477481474228));
#37155=CARTESIAN_POINT('Ctrl Pts',(11.6374451793146,-36.9827860357512,-3.57607605462277));
#37156=CARTESIAN_POINT('Ctrl Pts',(11.7209181578843,-36.993930211957,-3.30443412161567));
#37157=CARTESIAN_POINT('Ctrl Pts',(11.794881403517,-37.0050743881628,-3.02985055655883));
#37158=CARTESIAN_POINT('Ctrl Pts',(11.8591480264476,-37.0162185643687,-2.7530089605381));
#37159=CARTESIAN_POINT('Ctrl Pts',(11.9254385293136,-37.0277136921819,-2.46744908859315));
#37160=CARTESIAN_POINT('Ctrl Pts',(11.9814117057185,-37.0392088199951,-2.17948694843876));
#37161=CARTESIAN_POINT('Ctrl Pts',(12.0269190072913,-37.0507039478083,-1.88988609234936));
#37162=CARTESIAN_POINT('Ctrl Pts',(12.0710393075009,-37.061848719582,-1.60911188095839));
#37163=CARTESIAN_POINT('Ctrl Pts',(12.1053222141113,-37.0729934913558,-1.32679764184976));
#37164=CARTESIAN_POINT('Ctrl Pts',(12.129684684297,-37.0841382631295,-1.04364731089154));
#37165=CARTESIAN_POINT('Ctrl Pts',(12.1551959718931,-37.0958085689624,-0.747144966467237));
#37166=CARTESIAN_POINT('Ctrl Pts',(12.1698286831205,-37.1074788747954,-0.449726097386763));
#37167=CARTESIAN_POINT('Ctrl Pts',(12.1735485509352,-37.1191491806283,-0.152203574279836));
#37168=CARTESIAN_POINT('Ctrl Pts',(12.1772684187499,-37.1308194864613,0.145318948827091));
#37169=CARTESIAN_POINT('Ctrl Pts',(12.170075447735,-37.1424897922942,0.442944790376381));
#37170=CARTESIAN_POINT('Ctrl Pts',(12.1519980013252,-37.1541600981272,0.73986135578836));
#37171=CARTESIAN_POINT('Ctrl Pts',(12.134730690394,-37.1653074026142,1.02347169207873));
#37172=CARTESIAN_POINT('Ctrl Pts',(12.1075278724749,-37.1764547071013,1.30651963043172));
#37173=CARTESIAN_POINT('Ctrl Pts',(12.0704497066061,-37.1876020115883,1.58829913123846));
#37174=CARTESIAN_POINT('Ctrl Pts',(12.0333778384804,-37.1987474227007,1.87003077167098));
#37175=CARTESIAN_POINT('Ctrl Pts',(11.9864340059855,-37.2098928338131,2.15049414032514));
#37176=CARTESIAN_POINT('Ctrl Pts',(11.9297301073365,-37.2210382449255,2.4289894639765));
#37177=CARTESIAN_POINT('Ctrl Pts',(11.8730325037096,-37.2321824187225,2.70745387027918));
#37178=CARTESIAN_POINT('Ctrl Pts',(11.806577050753,-37.2433265925194,2.98395040653923));
#37179=CARTESIAN_POINT('Ctrl Pts',(11.730526779452,-37.2544707663164,3.25778939260328));
#37180=CARTESIAN_POINT('Ctrl Pts',(11.6520815091351,-37.2659658959327,3.5402522019744));
#37181=CARTESIAN_POINT('Ctrl Pts',(11.563427371625,-37.277461025549,3.81988707545358));
#37182=CARTESIAN_POINT('Ctrl Pts',(11.4647993244373,-37.2889561551654,4.09595247779841));
#37183=CARTESIAN_POINT('Ctrl Pts',(11.3691773629799,-37.3001009245536,4.36360367860211));
#37184=CARTESIAN_POINT('Ctrl Pts',(11.2641805724472,-37.3112456939418,4.6278995113326));
#37185=CARTESIAN_POINT('Ctrl Pts',(11.1500728991938,-37.3223904633301,4.88818213579082));
#37186=CARTESIAN_POINT('Ctrl Pts',(11.0305843891053,-37.3340607730604,5.16073859156343));
#37187=CARTESIAN_POINT('Ctrl Pts',(10.9011051867154,-37.3457310827908,5.4288939487069));
#37188=CARTESIAN_POINT('Ctrl Pts',(10.7619941971752,-37.3574013925212,5.6919180554509));
#37189=CARTESIAN_POINT('Ctrl Pts',(10.622883207635,-37.3690717022515,5.95494216219492));
#37190=CARTESIAN_POINT('Ctrl Pts',(10.4741405955607,-37.3807420119819,6.21283472606724));
#37191=CARTESIAN_POINT('Ctrl Pts',(10.3161801276997,-37.3924123217123,6.46489580912594));
#37192=CARTESIAN_POINT('Ctrl Pts',(10.1652985893882,-37.4035596315964,6.70566088456128));
#37193=CARTESIAN_POINT('Ctrl Pts',(10.0059621610874,-37.4147069414806,6.94117756831538));
#37194=CARTESIAN_POINT('Ctrl Pts',(9.83856153689548,-37.4258542513647,7.17085470043292));
#37195=CARTESIAN_POINT('Ctrl Pts',(9.67118934551754,-37.4369996678904,7.40049282213932));
#37196=CARTESIAN_POINT('Ctrl Pts',(9.49575584989997,-37.448145084416,7.62429315693641));
#37197=CARTESIAN_POINT('Ctrl Pts',(9.31269417572409,-37.4592905009417,7.84169480657305));
#37198=CARTESIAN_POINT('Ctrl Pts',(9.12965282422267,-37.4704346801539,8.05907232126732));
#37199=CARTESIAN_POINT('Ctrl Pts',(8.93898515694899,-37.4815788593662,8.27005236527149));
#37200=CARTESIAN_POINT('Ctrl Pts',(8.74116436747312,-37.4927230385784,8.47410737191938));
#37201=CARTESIAN_POINT('Ctrl Pts',(8.53711391475841,-37.5042181641383,8.68458836633621));
#37202=CARTESIAN_POINT('Ctrl Pts',(8.32545271468955,-37.5157132896982,8.88770087711783));
#37203=CARTESIAN_POINT('Ctrl Pts',(8.10674193044602,-37.5272084152581,9.08290622670676));
#37204=CARTESIAN_POINT('Ctrl Pts',(7.89469705879956,-37.5383531899996,9.27216206720614));
#37205=CARTESIAN_POINT('Ctrl Pts',(7.67602616543338,-37.549497964741,9.45398541568634));
#37206=CARTESIAN_POINT('Ctrl Pts',(7.45127581728972,-37.5606427394824,9.62792495528883));
#37207=CARTESIAN_POINT('Ctrl Pts',(7.21592747991917,-37.5723130404516,9.81006652608755));
#37208=CARTESIAN_POINT('Ctrl Pts',(6.97391279638077,-37.5839833414207,9.98356268944984));
#37209=CARTESIAN_POINT('Ctrl Pts',(6.72589631532803,-37.5956536423899,10.1479440777656));
#37210=CARTESIAN_POINT('Ctrl Pts',(6.47787983427525,-37.6073239433591,10.3123254660813));
#37211=CARTESIAN_POINT('Ctrl Pts',(6.22386184020973,-37.6189942443282,10.4675919013181));
#37212=CARTESIAN_POINT('Ctrl Pts',(5.96454059505376,-37.6306645452974,10.6133267988862));
#37213=CARTESIAN_POINT('Ctrl Pts',(5.71684074067779,-37.6418118458159,10.7525306380603));
#37214=CARTESIAN_POINT('Ctrl Pts',(5.46422853582719,-37.6529591463344,10.8830800410514));
#37215=CARTESIAN_POINT('Ctrl Pts',(5.20732992919923,-37.6641064468529,11.0046428955449));
#37216=CARTESIAN_POINT('Ctrl Pts',(4.95047495704132,-37.675251853992,11.1261851024731));
#37217=CARTESIAN_POINT('Ctrl Pts',(4.68933527768077,-37.686397261131,11.238743694257));
#37218=CARTESIAN_POINT('Ctrl Pts',(4.42455961597228,-37.69754266827,11.3420334356194));
#37219=CARTESIAN_POINT('Ctrl Pts',(4.159813348394,-37.7086868380991,11.4453117102476));
#37220=CARTESIAN_POINT('Ctrl Pts',(3.8914321529359,-37.7198310079283,11.5393230922518));
#37221=CARTESIAN_POINT('Ctrl Pts',(3.62008398605781,-37.7309751777574,11.6238307878207));
#37222=CARTESIAN_POINT('Ctrl Pts',(3.34019026538018,-37.7424703103512,11.7109998798798));
#37223=CARTESIAN_POINT('Ctrl Pts',(3.05713994801186,-37.7539654429449,11.7880568895911));
#37224=CARTESIAN_POINT('Ctrl Pts',(2.77168355359457,-37.7654605755387,11.8547973634615));
#37225=CARTESIAN_POINT('Ctrl Pts',(2.4949277575709,-37.7766053410216,11.919503613993));
#37226=CARTESIAN_POINT('Ctrl Pts',(2.21591065681822,-37.7877501065045,11.9745128402229));
#37227=CARTESIAN_POINT('Ctrl Pts',(1.93532814556136,-37.7988948719875,12.0196903129406));
#37228=CARTESIAN_POINT('Ctrl Pts',(1.64151428134749,-37.8105651881366,12.0669982074175));
#37229=CARTESIAN_POINT('Ctrl Pts',(1.34598412860745,-37.8222355042858,12.1035247188786));
#37230=CARTESIAN_POINT('Ctrl Pts',(1.04954582011979,-37.833905820435,12.1291757272071));
#37231=CARTESIAN_POINT('Ctrl Pts',(0.753107511632138,-37.8455761365842,
12.1548267355356));
#37232=CARTESIAN_POINT('Ctrl Pts',(0.455761382408362,-37.8572464527333,
12.1696022205541));
#37233=CARTESIAN_POINT('Ctrl Pts',(0.158319908679642,-37.8689167688825,
12.173470542804));
#37234=CARTESIAN_POINT('Ctrl Pts',(-0.12579174714374,-37.8800640806665,
12.1771655064749));
#37235=CARTESIAN_POINT('Ctrl Pts',(-0.410075244090248,-37.8912113924504,
12.1709105297779));
#37236=CARTESIAN_POINT('Ctrl Pts',(-0.693822027690313,-37.9023587042343,
12.1547135401823));
#37237=CARTESIAN_POINT('Ctrl Pts',(-0.977520616905607,-37.9135041226476,
12.138519301645));
#37238=CARTESIAN_POINT('Ctrl Pts',(-1.26068240856468,-37.9246495410609,
12.1123864367958));
#37239=CARTESIAN_POINT('Ctrl Pts',(-1.54260128195007,-37.9357949594741,
12.076374933519));
#37240=CARTESIAN_POINT('Ctrl Pts',(-1.82448885756125,-37.946939140557,12.0403674281296));
#37241=CARTESIAN_POINT('Ctrl Pts',(-2.10513352590396,-37.9580833216399,
11.994483508031));
#37242=CARTESIAN_POINT('Ctrl Pts',(-2.38383546099295,-37.9692275027228,
11.938834898972));
#37243=CARTESIAN_POINT('Ctrl Pts',(-2.67131404013532,-37.9807226268682,
11.8814338512957));
#37244=CARTESIAN_POINT('Ctrl Pts',(-2.95672525267067,-37.9922177510136,
11.8136431952161));
#37245=CARTESIAN_POINT('Ctrl Pts',(-3.23931225686239,-38.003712875159,11.7356425624054));
#37246=CARTESIAN_POINT('Ctrl Pts',(-3.5132865939056,-38.0148576517066,11.660019227481));
#37247=CARTESIAN_POINT('Ctrl Pts',(-3.78460605649515,-38.0260024282542,
11.574799132407));
#37248=CARTESIAN_POINT('Ctrl Pts',(-4.05259512972714,-38.0371472048018,
11.4801969915377));
#37249=CARTESIAN_POINT('Ctrl Pts',(-4.33322097422808,-38.0488175027461,
11.3811339761959));
#37250=CARTESIAN_POINT('Ctrl Pts',(-4.61019448973457,-38.0604878006904,
11.2717829285037));
#37251=CARTESIAN_POINT('Ctrl Pts',(-4.88276104735159,-38.0721580986347,
11.1524479287942));
#37252=CARTESIAN_POINT('Ctrl Pts',(-5.15532760496862,-38.083828396579,11.0331129290847));
#37253=CARTESIAN_POINT('Ctrl Pts',(-5.42348690088356,-38.0954986945234,
10.903794119955));
#37254=CARTESIAN_POINT('Ctrl Pts',(-5.68651039168178,-38.1071689924677,
10.7648525217624));
#37255=CARTESIAN_POINT('Ctrl Pts',(-5.93774685158698,-38.1183163022865,
10.6321373975067));
#37256=CARTESIAN_POINT('Ctrl Pts',(-6.18437272836615,-38.1294636121054,
10.4906033555107));
#37257=CARTESIAN_POINT('Ctrl Pts',(-6.42576965953203,-38.1406109219243,
10.340596430218));
#37258=CARTESIAN_POINT('Ctrl Pts',(-6.66712559058785,-38.1517563384261,
10.1906149828815));
#37259=CARTESIAN_POINT('Ctrl Pts',(-6.9032541226648,-38.1629017549279,10.0321636661054));
#37260=CARTESIAN_POINT('Ctrl Pts',(-7.13356394341092,-38.1740471714297,
9.86563306206286));
#37261=CARTESIAN_POINT('Ctrl Pts',(-7.36384819705636,-38.1851913506591,
9.69912094487725));
#37262=CARTESIAN_POINT('Ctrl Pts',(-7.58831481311788,-38.1963355298885,
9.52453148764227));
#37263=CARTESIAN_POINT('Ctrl Pts',(-7.80640276521373,-38.2074797091179,
9.34229768939438));
#37264=CARTESIAN_POINT('Ctrl Pts',(-8.03135862286497,-38.2189748346958,
9.15432508483766));
#37265=CARTESIAN_POINT('Ctrl Pts',(-8.24952732595125,-38.2304699602737,
8.95821905765051));
#37266=CARTESIAN_POINT('Ctrl Pts',(-8.46033028003315,-38.2419650858516,
8.75449951754835));
#37267=CARTESIAN_POINT('Ctrl Pts',(-8.66470833983174,-38.2531098607101,
8.55698898203202));
#37268=CARTESIAN_POINT('Ctrl Pts',(-8.86216279097333,-38.2642546355686,
8.35232234771498));
#37269=CARTESIAN_POINT('Ctrl Pts',(-9.05220323824906,-38.2753994104272,
8.14101141034904));
#37270=CARTESIAN_POINT('Ctrl Pts',(-9.25120494426631,-38.2870697113648,
7.91973621531168));
#37271=CARTESIAN_POINT('Ctrl Pts',(-9.44207640298544,-38.2987400123023,
7.69117525897117));
#37272=CARTESIAN_POINT('Ctrl Pts',(-9.6243005169155,-38.3104103132399,7.45595666632393));
#37273=CARTESIAN_POINT('Ctrl Pts',(-9.80652463084557,-38.3220806141775,
7.22073807367666));
#37274=CARTESIAN_POINT('Ctrl Pts',(-9.98010120145821,-38.3337509151151,
6.97886211532039));
#37275=CARTESIAN_POINT('Ctrl Pts',(-10.144563284333,-38.3454212160527,6.73099443025792));
#37276=CARTESIAN_POINT('Ctrl Pts',(-10.3016546456759,-38.3565684873844,
6.49423546795641));
#37277=CARTESIAN_POINT('Ctrl Pts',(-10.4504774518845,-38.367715758716,6.25193932153469));
#37278=CARTESIAN_POINT('Ctrl Pts',(-10.5906543344632,-38.3788630300476,
6.00470573949428));
#37279=CARTESIAN_POINT('Ctrl Pts',(-10.7308074057654,-38.3900084078376,
5.7575141540162));
#37280=CARTESIAN_POINT('Ctrl Pts',(-10.8623173540756,-38.4011537856276,
5.50538703934738));
#37281=CARTESIAN_POINT('Ctrl Pts',(-10.9848518805822,-38.4122991634176,
5.24895031522197));
#37282=CARTESIAN_POINT('Ctrl Pts',(-11.1073728029286,-38.4234433038135,
4.99254206149096));
#37283=CARTESIAN_POINT('Ctrl Pts',(-11.2209201783031,-38.4345874442093,
4.73182539434702));
#37284=CARTESIAN_POINT('Ctrl Pts',(-11.3252085991643,-38.4457315846052,
4.46744898520573));
#37285=CARTESIAN_POINT('Ctrl Pts',(-11.4327818597973,-38.4572267391913,
4.19474534149411));
#37286=CARTESIAN_POINT('Ctrl Pts',(-11.5305033242619,-38.4687218937773,
3.91814794521018));
#37287=CARTESIAN_POINT('Ctrl Pts',(-11.6181137451896,-38.4802170483634,
3.63839020087693));
#37288=CARTESIAN_POINT('Ctrl Pts',(-11.7030534493892,-38.4913617845709,
3.36716059371813));
#37289=CARTESIAN_POINT('Ctrl Pts',(-11.7784893469094,-38.5025065207784,
3.09296073127381));
#37290=CARTESIAN_POINT('Ctrl Pts',(-11.8442357567959,-38.513651256986,2.81647467367221));
#37291=CARTESIAN_POINT('Ctrl Pts',(-11.9130830140131,-38.5253216207613,
2.52694849638708));
#37292=CARTESIAN_POINT('Ctrl Pts',(-11.9713047289161,-38.5369919845366,
2.23491559225353));
#37293=CARTESIAN_POINT('Ctrl Pts',(-12.0187474391742,-38.5486623483119,
1.94117496463956));
#37294=CARTESIAN_POINT('Ctrl Pts',(-12.0661901494323,-38.5603327120872,
1.64743433702562));
#37295=CARTESIAN_POINT('Ctrl Pts',(-12.1028538102164,-38.5720030758626,
1.35198631855737));
#37296=CARTESIAN_POINT('Ctrl Pts',(-12.1286469510863,-38.5836734396379,
1.05563885202526));
#37297=CARTESIAN_POINT('Ctrl Pts',(-12.1549901730804,-38.5955926931028,
0.752971288674556));
#37298=CARTESIAN_POINT('Ctrl Pts',(-12.1700001024465,-38.6075119465678,
0.449311157315627));
#37299=CARTESIAN_POINT('Ctrl Pts',(-12.173630879507,-38.6194312000327,0.145469789009793));
#37300=CARTESIAN_POINT('Ctrl Pts',(-12.1742091193982,-38.6213294680102,
0.0970798171563845));
#37301=CARTESIAN_POINT('Ctrl Pts',(-12.1744988461963,-38.6232277359876,
0.0486852550215822));
#37302=CARTESIAN_POINT('Ctrl Pts',(-12.1744999965607,-38.6251260039651,
0.00028938649696687));
#37303=CARTESIAN_POINT('Origin',(0.,-13.3748739960349,0.));
#37304=CARTESIAN_POINT('',(7.412721799411,-33.6876951030527,-9.65763976210218));
#37305=CARTESIAN_POINT('',(7.412721799411,-33.9374387645002,-9.65763976210218));
#37306=CARTESIAN_POINT('',(7.41272179941101,-13.3748739960349,-9.65763976210217));
#37307=CARTESIAN_POINT('',(-12.1744999966649,-35.8748739960676,-0.000284967810357368));
#37308=CARTESIAN_POINT('Ctrl Pts',(7.41272179941099,-33.9374387645002,-9.65763976210218));
#37309=CARTESIAN_POINT('Ctrl Pts',(7.638184643001,-33.9485835323456,-9.48458574716623));
#37310=CARTESIAN_POINT('Ctrl Pts',(7.857581029635,-33.959728300191,-9.30363583840648));
#37311=CARTESIAN_POINT('Ctrl Pts',(8.07036553404239,-33.9708730680363,-9.11524275030241));
#37312=CARTESIAN_POINT('Ctrl Pts',(8.28315653782117,-33.9820181762918,-8.92684390784772));
#37313=CARTESIAN_POINT('Ctrl Pts',(8.48933505810636,-33.9931632845472,-8.73100161084966));
#37314=CARTESIAN_POINT('Ctrl Pts',(8.68839053721542,-34.0043083928026,-8.52820732175441));
#37315=CARTESIAN_POINT('Ctrl Pts',(8.88748351632993,-34.0154556006818,-8.32537482830037));
#37316=CARTESIAN_POINT('Ctrl Pts',(9.07945058689651,-34.0266028085611,-8.11558791699093));
#37317=CARTESIAN_POINT('Ctrl Pts',(9.26381869082178,-34.0377500164403,-7.89937424822885));
#37318=CARTESIAN_POINT('Ctrl Pts',(9.29659092252151,-34.0397314810844,-7.8609413289849));
#37319=CARTESIAN_POINT('Ctrl Pts',(9.3291231530178,-34.0417129457284,-7.82230543318109));
#37320=CARTESIAN_POINT('Ctrl Pts',(9.36141285701634,-34.0436944103725,-7.78346963574017));
#37321=CARTESIAN_POINT('Ctrl Pts',(9.54306798782381,-34.0548417166199,-7.56498755041469));
#37322=CARTESIAN_POINT('Ctrl Pts',(9.71709831636431,-34.0659890228673,-7.34011069825187));
#37323=CARTESIAN_POINT('Ctrl Pts',(9.88306413050628,-34.0771363291147,-7.10939474514534));
#37324=CARTESIAN_POINT('Ctrl Pts',(10.0490017553756,-34.0882817419936,-6.87871797911443));
#37325=CARTESIAN_POINT('Ctrl Pts',(10.2068774448553,-34.0994271548724,-6.64220430866852));
#37326=CARTESIAN_POINT('Ctrl Pts',(10.356293478878,-34.1105725677512,-6.40044026839951));
#37327=CARTESIAN_POINT('Ctrl Pts',(10.5056929254,-34.1217167433161,-6.15870306769419));
#37328=CARTESIAN_POINT('Ctrl Pts',(10.6466344516049,-34.132860918881,-5.91171688792128));
#37329=CARTESIAN_POINT('Ctrl Pts',(10.7787645084179,-34.1440050944459,-5.66009592869868));
#37330=CARTESIAN_POINT('Ctrl Pts',(10.9150556091399,-34.1555002227386,-5.40055091430638));
#37331=CARTESIAN_POINT('Ctrl Pts',(11.0419711186301,-34.1669953510312,-5.13607473106142));
#37332=CARTESIAN_POINT('Ctrl Pts',(11.1591743840538,-34.1784904793239,-4.86736862342242));
#37333=CARTESIAN_POINT('Ctrl Pts',(11.2728054403154,-34.1896352504617,-4.6068523423738));
#37334=CARTESIAN_POINT('Ctrl Pts',(11.3773074082564,-34.2007800215995,-4.34236042018621));
#37335=CARTESIAN_POINT('Ctrl Pts',(11.4724220783378,-34.2119247927374,-4.07455297013887));
#37336=CARTESIAN_POINT('Ctrl Pts',(11.5720219152447,-34.2235950996074,-3.79411696248277));
#37337=CARTESIAN_POINT('Ctrl Pts',(11.6613277225685,-34.2352654064774,-3.5100455127723));
#37338=CARTESIAN_POINT('Ctrl Pts',(11.7401009596519,-34.2469357133475,-3.22311645883009));
#37339=CARTESIAN_POINT('Ctrl Pts',(11.8188741967353,-34.2586060202175,-2.93618740488788));
#37340=CARTESIAN_POINT('Ctrl Pts',(11.8871147832216,-34.2702763270876,-2.64640107256773));
#37341=CARTESIAN_POINT('Ctrl Pts',(11.9446448465681,-34.2819466339576,-2.35455085724545));
#37342=CARTESIAN_POINT('Ctrl Pts',(11.9995967207427,-34.2930939402076,-2.07577980473253));
#37343=CARTESIAN_POINT('Ctrl Pts',(12.0447933593859,-34.3042412464575,-1.79504252936051));
#37344=CARTESIAN_POINT('Ctrl Pts',(12.0801145768396,-34.3153885527074,-1.51303736253506));
#37345=CARTESIAN_POINT('Ctrl Pts',(12.1154297949892,-34.3265339655889,-1.23108009425072));
#37346=CARTESIAN_POINT('Ctrl Pts',(12.1408729076176,-34.3376793784703,-0.947855629040423));
#37347=CARTESIAN_POINT('Ctrl Pts',(12.1563753727891,-34.3488247913517,-0.664069308015263));
#37348=CARTESIAN_POINT('Ctrl Pts',(12.1718761169461,-34.3599689669192,-0.380314491679434));
#37349=CARTESIAN_POINT('Ctrl Pts',(12.1774384027462,-34.3711131424867,-0.0959982103629502));
#37350=CARTESIAN_POINT('Ctrl Pts',(12.1730457121208,-34.3822573180542,0.188171040858175));
#37351=CARTESIAN_POINT('Ctrl Pts',(12.1685146867457,-34.3937524463449,0.481289358968064));
#37352=CARTESIAN_POINT('Ctrl Pts',(12.1533915147295,-34.4052475746356,0.774250939540593));
#37353=CARTESIAN_POINT('Ctrl Pts',(12.1277161686617,-34.4167427029263,1.06627894210765));
#37354=CARTESIAN_POINT('Ctrl Pts',(12.1028233750677,-34.4278874740667,1.34940629596561));
#37355=CARTESIAN_POINT('Ctrl Pts',(12.0680121410407,-34.4390322452072,1.63165585970076));
#37356=CARTESIAN_POINT('Ctrl Pts',(12.0233716344006,-34.4501770163476,1.91232444713011));
#37357=CARTESIAN_POINT('Ctrl Pts',(11.9766260884783,-34.4618473232134,2.20622806360036));
#37358=CARTESIAN_POINT('Ctrl Pts',(11.9191020086131,-34.4735176300793,2.49839769914427));
#37359=CARTESIAN_POINT('Ctrl Pts',(11.8509621693877,-34.4851879369452,2.78803621026358));
#37360=CARTESIAN_POINT('Ctrl Pts',(11.7828223301624,-34.496858243811,3.07767472138287));
#37361=CARTESIAN_POINT('Ctrl Pts',(11.7040668169537,-34.5085285506769,3.36478178350285));
#37362=CARTESIAN_POINT('Ctrl Pts',(11.6149191198025,-34.5201988575427,3.64857562487699));
#37363=CARTESIAN_POINT('Ctrl Pts',(11.5297665448279,-34.5313461637786,3.91965134670903));
#37364=CARTESIAN_POINT('Ctrl Pts',(11.4351073244025,-34.5424934700145,4.18778524183307));
#37365=CARTESIAN_POINT('Ctrl Pts',(11.3311701091902,-34.5536407762504,4.45230661641746));
#37366=CARTESIAN_POINT('Ctrl Pts',(11.2272505477016,-34.5647861891177,4.71678306207768));
#37367=CARTESIAN_POINT('Ctrl Pts',(11.1140562351574,-34.575931601985,4.97764796404744));
#37368=CARTESIAN_POINT('Ctrl Pts',(10.9918645231726,-34.5870770148522,5.2342491872493));
#37369=CARTESIAN_POINT('Ctrl Pts',(10.8696863763659,-34.5982211904055,5.49082192372942));
#37370=CARTESIAN_POINT('Ctrl Pts',(10.7385129393202,-34.6093653659588,5.743131685842));
#37371=CARTESIAN_POINT('Ctrl Pts',(10.5986687532571,-34.6205095415121,5.99054846476783));
#37372=CARTESIAN_POINT('Ctrl Pts',(10.4544205894249,-34.6320046698134,6.24575690114288));
#37373=CARTESIAN_POINT('Ctrl Pts',(10.3009468455545,-34.6434997981147,6.49575891739394));
#37374=CARTESIAN_POINT('Ctrl Pts',(10.1386543714878,-34.6549949264161,6.73989152624218));
#37375=CARTESIAN_POINT('Ctrl Pts',(9.98130836963331,-34.6661396975425,6.97658327763416));
#37376=CARTESIAN_POINT('Ctrl Pts',(9.81567339958986,-34.6772844686689,7.20775787559392));
#37377=CARTESIAN_POINT('Ctrl Pts',(9.64216426105065,-34.6884292397953,7.43284054806221));
#37378=CARTESIAN_POINT('Ctrl Pts',(9.46047323556585,-34.7000995466841,7.66853707634841));
#37379=CARTESIAN_POINT('Ctrl Pts',(9.27014774830922,-34.7117698535728,7.89755306912699));
#37380=CARTESIAN_POINT('Ctrl Pts',(9.07171219303635,-34.7234401604616,8.11926647775005));
#37381=CARTESIAN_POINT('Ctrl Pts',(8.87327663776348,-34.7351104673503,8.3409798863731));
#37382=CARTESIAN_POINT('Ctrl Pts',(8.66673124476339,-34.7467807742391,8.55539046669953));
#37383=CARTESIAN_POINT('Ctrl Pts',(8.45264636382744,-34.7584510811278,8.76191872240749));
#37384=CARTESIAN_POINT('Ctrl Pts',(8.24815561997432,-34.769598387403,8.95919148847938));
#37385=CARTESIAN_POINT('Ctrl Pts',(8.03672521997992,-34.7807456936781,9.14933180573395));
#37386=CARTESIAN_POINT('Ctrl Pts',(7.81887688946857,-34.7918929999533,9.33186018097862));
#37387=CARTESIAN_POINT('Ctrl Pts',(7.60106556046648,-34.80303841286,9.51435755380363));
#37388=CARTESIAN_POINT('Ctrl Pts',(7.37683868168765,-34.8141838257667,9.68924539461877));
#37389=CARTESIAN_POINT('Ctrl Pts',(7.14675186016544,-34.8253292386734,9.85608381149541));
#37390=CARTESIAN_POINT('Ctrl Pts',(6.91669058185361,-34.8364734142662,10.0229037067168));
#37391=CARTESIAN_POINT('Ctrl Pts',(6.68077087572726,-34.8476175898589,10.1816758058515));
#37392=CARTESIAN_POINT('Ctrl Pts',(6.43957919596821,-34.8587617654517,10.3320022274898));
#37393=CARTESIAN_POINT('Ctrl Pts',(6.19079190131112,-34.8702568937235,10.4870627328614));
#37394=CARTESIAN_POINT('Ctrl Pts',(5.93639544874569,-34.8817520219953,10.6331368327272));
#37395=CARTESIAN_POINT('Ctrl Pts',(5.67706434630255,-34.893247150267,10.7698370766665));
#37396=CARTESIAN_POINT('Ctrl Pts',(5.42563733091963,-34.9043919214325,10.9023708684562));
#37397=CARTESIAN_POINT('Ctrl Pts',(5.16957226212979,-34.9155366925979,11.0260936195817));
#37398=CARTESIAN_POINT('Ctrl Pts',(4.90950841370616,-34.9266814637634,11.1406991425919));
#37399=CARTESIAN_POINT('Ctrl Pts',(4.63718116174956,-34.9383517705883,11.2607089299177));
#37400=CARTESIAN_POINT('Ctrl Pts',(4.3604692188947,-34.9500220774132,11.3707208190715));
#37401=CARTESIAN_POINT('Ctrl Pts',(4.08013071339311,-34.9616923842381,11.4704395561646));
#37402=CARTESIAN_POINT('Ctrl Pts',(3.7997922078915,-34.973362691063,11.5701582932578));
#37403=CARTESIAN_POINT('Ctrl Pts',(3.51582745878365,-34.985032997888,11.6595837741217));
#37404=CARTESIAN_POINT('Ctrl Pts',(3.22901458356905,-34.9967033047129,11.7384801004686));
#37405=CARTESIAN_POINT('Ctrl Pts',(2.95505512490198,-35.0078506109063,11.8138407161336));
#37406=CARTESIAN_POINT('Ctrl Pts',(2.67841538341678,-35.0189979170997,11.8796176615914));
#37407=CARTESIAN_POINT('Ctrl Pts',(2.39978292570686,-35.0301452232932,11.9356395789872));
#37408=CARTESIAN_POINT('Ctrl Pts',(2.1211977936875,-35.0412906361179,11.9916519810668));
#37409=CARTESIAN_POINT('Ctrl Pts',(1.8406208825985,-35.0524360489427,12.0379126105056));
#37410=CARTESIAN_POINT('Ctrl Pts',(1.55875055819259,-35.0635814617674,12.0743010956053));
#37411=CARTESIAN_POINT('Ctrl Pts',(1.27691152577331,-35.0747256372782,12.1106855410175));
#37412=CARTESIAN_POINT('Ctrl Pts',(0.9937796312455,-35.0858698127889,12.1371999964074));
#37413=CARTESIAN_POINT('Ctrl Pts',(0.710060222313936,-35.0970139882996,
12.1537757396904));
#37414=CARTESIAN_POINT('Ctrl Pts',(0.417405910368738,-35.1085091166328,
12.1708734869462));
#37415=CARTESIAN_POINT('Ctrl Pts',(0.124126775978267,-35.120004244966,12.1773963708101));
#37416=CARTESIAN_POINT('Ctrl Pts',(-0.168999507858268,-35.1314993732992,
12.1733269658029));
#37417=CARTESIAN_POINT('Ctrl Pts',(-0.453191666266195,-35.1426441443837,
12.1693815912111));
#37418=CARTESIAN_POINT('Ctrl Pts',(-0.737239874493748,-35.1537889154681,
12.155480050062));
#37419=CARTESIAN_POINT('Ctrl Pts',(-1.02043628531443,-35.1649336865525,
12.1316594098917));
#37420=CARTESIAN_POINT('Ctrl Pts',(-1.31698692942595,-35.1766039935101,
12.1067154984728));
#37421=CARTESIAN_POINT('Ctrl Pts',(-1.61260319276483,-35.1882743004677,
12.0708945277011));
#37422=CARTESIAN_POINT('Ctrl Pts',(-1.9064780983657,-35.1999446074253,12.0243000424329));
#37423=CARTESIAN_POINT('Ctrl Pts',(-2.20035300396654,-35.2116149143829,
11.9777055571647));
#37424=CARTESIAN_POINT('Ctrl Pts',(-2.49248622184222,-35.2232852213404,
11.920337618608));
#37425=CARTESIAN_POINT('Ctrl Pts',(-2.78208162737388,-35.234955528298,11.8523614553653));
#37426=CARTESIAN_POINT('Ctrl Pts',(-3.05869891833767,-35.2461028346215,
11.7874316195767));
#37427=CARTESIAN_POINT('Ctrl Pts',(-3.33308347439242,-35.2572501409449,
11.7128040752966));
#37428=CARTESIAN_POINT('Ctrl Pts',(-3.60454956580632,-35.2683974472683,
11.6286573892967));
#37429=CARTESIAN_POINT('Ctrl Pts',(-3.87596954874084,-35.2795428602233,
11.5445249956003));
#37430=CARTESIAN_POINT('Ctrl Pts',(-4.14447180201004,-35.2906882731782,
11.4508767671215));
#37431=CARTESIAN_POINT('Ctrl Pts',(-4.40938551257941,-35.3018336861332,
11.3479412076136));
#37432=CARTESIAN_POINT('Ctrl Pts',(-4.67426981361183,-35.3129778617742,
11.2450170755518));
#37433=CARTESIAN_POINT('Ctrl Pts',(-4.9355661188806,-35.3241220374152,11.1328077678662));
#37434=CARTESIAN_POINT('Ctrl Pts',(-5.19262220129437,-35.3352662130561,
11.0115904811532));
#37435=CARTESIAN_POINT('Ctrl Pts',(-5.45777349882198,-35.3467613412917,
10.8865558173052));
#37436=CARTESIAN_POINT('Ctrl Pts',(-5.71841290697284,-35.3582564695273,
10.7519367395923));
#37437=CARTESIAN_POINT('Ctrl Pts',(-5.97384924005429,-35.3697515977629,
10.6080900970487));
#37438=CARTESIAN_POINT('Ctrl Pts',(-6.22150019559604,-35.3808963689756,
10.4686277188989));
#37439=CARTESIAN_POINT('Ctrl Pts',(-6.46426030265879,-35.3920411401884,
10.3204920726344));
#37440=CARTESIAN_POINT('Ctrl Pts',(-6.70152576426091,-35.4031859114011,
10.1640544410657));
#37441=CARTESIAN_POINT('Ctrl Pts',(-6.94997956062028,-35.4148562181481,
10.0002399389706));
#37442=CARTESIAN_POINT('Ctrl Pts',(-7.19240777343318,-35.4265265248951,
9.82732182100891));
#37443=CARTESIAN_POINT('Ctrl Pts',(-7.42815137572672,-35.4381968316421,
9.64577717912296));
#37444=CARTESIAN_POINT('Ctrl Pts',(-7.66389497802024,-35.4498671383891,
9.46423253723702));
#37445=CARTESIAN_POINT('Ctrl Pts',(-7.89295370933516,-35.4615374451361,
9.27406158308419));
#37446=CARTESIAN_POINT('Ctrl Pts',(-8.11470759005776,-35.4732077518831,
9.0757903775847));
#37447=CARTESIAN_POINT('Ctrl Pts',(-8.32652365126632,-35.4843550580777,
8.88640462404963));
#37448=CARTESIAN_POINT('Ctrl Pts',(-8.53173846022696,-35.4955023642722,
8.68957211823678));
#37449=CARTESIAN_POINT('Ctrl Pts',(-8.72983535399109,-35.5066496704667,
8.48577780419729));
#37450=CARTESIAN_POINT('Ctrl Pts',(-8.92789860102508,-35.5177950832929,
8.28201810459399));
#37451=CARTESIAN_POINT('Ctrl Pts',(-9.11884616072902,-35.528940496119,8.07129914875044));
#37452=CARTESIAN_POINT('Ctrl Pts',(-9.30219836495137,-35.5400859089451,
7.85414259032112));
#37453=CARTESIAN_POINT('Ctrl Pts',(-9.48553021423546,-35.5512300844576,
7.63701013963763));
#37454=CARTESIAN_POINT('Ctrl Pts',(-9.66126821973614,-35.56237425997,7.41344171722012));
#37455=CARTESIAN_POINT('Ctrl Pts',(-9.82897233455958,-35.5735184354825,
7.18399283800189));
#37456=CARTESIAN_POINT('Ctrl Pts',(-10.0019577940555,-35.5850135638146,
6.94731814552835));
#37457=CARTESIAN_POINT('Ctrl Pts',(-10.1663949731909,-35.5965086921468,
6.70438685320291));
#37458=CARTESIAN_POINT('Ctrl Pts',(-10.3218477339838,-35.6080038204789,
6.45584305931104));
#37459=CARTESIAN_POINT('Ctrl Pts',(-10.4725624875548,-35.6191485915657,
6.21487457179775));
#37460=CARTESIAN_POINT('Ctrl Pts',(-10.6148322327911,-35.6302933626525,
5.96863087732274));
#37461=CARTESIAN_POINT('Ctrl Pts',(-10.7483044718205,-35.6414381337393,
5.71772692868804));
#37462=CARTESIAN_POINT('Ctrl Pts',(-10.8880706444308,-35.6531084406941,
5.45499151008326));
#37463=CARTESIAN_POINT('Ctrl Pts',(-11.0181894980664,-35.6647787476489,
5.18714603041487));
#37464=CARTESIAN_POINT('Ctrl Pts',(-11.1383106735327,-35.6764490546037,
4.91492477967551));
#37465=CARTESIAN_POINT('Ctrl Pts',(-11.2584318489989,-35.6881193615585,
4.64270352893615));
#37466=CARTESIAN_POINT('Ctrl Pts',(-11.3685552188829,-35.6997896685134,
4.36610681761556));
#37467=CARTESIAN_POINT('Ctrl Pts',(-11.4683881438355,-35.7114599754682,
4.08589324778976));
#37468=CARTESIAN_POINT('Ctrl Pts',(-11.5636605180159,-35.7225971614369,
3.81848034680994));
#37469=CARTESIAN_POINT('Ctrl Pts',(-11.6495908466594,-35.7337343474056,
3.54769134091233));
#37470=CARTESIAN_POINT('Ctrl Pts',(-11.7259574475739,-35.7448715333744,
3.27419794570916));
#37471=CARTESIAN_POINT('Ctrl Pts',(-11.8023132777083,-35.7560071485493,
3.00074312413884));
#37472=CARTESIAN_POINT('Ctrl Pts',(-11.8691079996121,-35.7671427637243,
2.72458493211118));
#37473=CARTESIAN_POINT('Ctrl Pts',(-11.9261699500892,-35.7782783788992,
2.44640973093008));
#37474=CARTESIAN_POINT('Ctrl Pts',(-11.9832242232964,-35.7894124958583,
2.16827195619616));
#37475=CARTESIAN_POINT('Ctrl Pts',(-12.0305482866717,-35.8005466128173,
1.88811797652426));
#37476=CARTESIAN_POINT('Ctrl Pts',(-12.0680214761787,-35.8116807297764,
1.60664492047536));
#37477=CARTESIAN_POINT('Ctrl Pts',(-12.1054959778234,-35.8228152366007,
1.32516200854266));
#37478=CARTESIAN_POINT('Ctrl Pts',(-12.1331188783859,-35.833949743425,1.04236019299949));
#37479=CARTESIAN_POINT('Ctrl Pts',(-12.1508211493447,-35.8450842502493,
0.758943770405247));
#37480=CARTESIAN_POINT('Ctrl Pts',(-12.1666082922634,-35.8550141655112,
0.506188879272841));
#37481=CARTESIAN_POINT('Ctrl Pts',(-12.1745059239959,-35.864944080773,0.252945394476219));
#37482=CARTESIAN_POINT('Ctrl Pts',(-12.1744999966649,-35.8748739960349,
-0.000284966977105543));
#37483=CARTESIAN_POINT('Ctrl Pts',(-12.1744999966649,-35.8748739960676,
-0.000284967810371163));
#37484=CARTESIAN_POINT('Ctrl Pts',(-12.1744930883501,-35.8864472961776,
-0.295424542797684));
#37485=CARTESIAN_POINT('Ctrl Pts',(-12.163749488268,-35.8980205962875,-0.590512724686085));
#37486=CARTESIAN_POINT('Ctrl Pts',(-12.1423063610032,-35.9095938963975,
-0.884786124179511));
#37487=CARTESIAN_POINT('Ctrl Pts',(-12.1208567139894,-35.9211707153511,
-1.17914899703588));
#37488=CARTESIAN_POINT('Ctrl Pts',(-12.0887010545349,-35.9327475343047,
-1.47269637376915));
#37489=CARTESIAN_POINT('Ctrl Pts',(-12.0459284961632,-35.9443243532583,
-1.76466906680104));
#37490=CARTESIAN_POINT('Ctrl Pts',(-12.0392930536843,-35.9461203018566,
-1.80996371560749));
#37491=CARTESIAN_POINT('Ctrl Pts',(-12.0324022028897,-35.9479162504549,
-1.85522048095315));
#37492=CARTESIAN_POINT('Ctrl Pts',(-12.0252563877582,-35.9497121990533,
-1.90043654423916));
#37493=CARTESIAN_POINT('Ctrl Pts',(-11.9809028943906,-35.9608595059425,
-2.18108897173295));
#37494=CARTESIAN_POINT('Ctrl Pts',(-11.9267134419172,-35.9720068128318,
-2.46022991528048));
#37495=CARTESIAN_POINT('Ctrl Pts',(-11.8628155407781,-35.9831541197211,
-2.73716234364608));
#37496=CARTESIAN_POINT('Ctrl Pts',(-11.7989284926723,-35.9942995332446,
-3.01404773514772));
#37497=CARTESIAN_POINT('Ctrl Pts',(-11.7253363480305,-36.0054449467682,
-3.28872510056579));
#37498=CARTESIAN_POINT('Ctrl Pts',(-11.6422175183502,-36.0165903602918,
-3.56050860207074));
#37499=CARTESIAN_POINT('Ctrl Pts',(-11.559107916142,-36.0277345365026,-3.8322619314151));
#37500=CARTESIAN_POINT('Ctrl Pts',(-11.466473818764,-36.0388787127133,-4.10112178333928));
#37501=CARTESIAN_POINT('Ctrl Pts',(-11.3645435686143,-36.0500228889241,
-4.36641726442477));
#37502=CARTESIAN_POINT('Ctrl Pts',(-11.2594033383302,-36.0615180167336,
-4.64006741179234));
#37503=CARTESIAN_POINT('Ctrl Pts',(-11.1443720573033,-36.0730131445432,
-4.90992477220224));
#37504=CARTESIAN_POINT('Ctrl Pts',(-11.0197546303388,-36.0845082723527,
-5.17527372581657));
#37505=CARTESIAN_POINT('Ctrl Pts',(-10.8989353748965,-36.0956530441313,
-5.43253520030673));
#37506=CARTESIAN_POINT('Ctrl Pts',(-10.7691057848687,-36.1067978159099,
-5.68555876622977));
#37507=CARTESIAN_POINT('Ctrl Pts',(-10.6305916042168,-36.1179425876886,
-5.93371488987754));
#37508=CARTESIAN_POINT('Ctrl Pts',(-10.4855457583789,-36.1296128935136,
-6.19357286748642));
#37509=CARTESIAN_POINT('Ctrl Pts',(-10.3309767217692,-36.1412831993385,
-6.44809302920758));
#37510=CARTESIAN_POINT('Ctrl Pts',(-10.1673116861847,-36.1529535051635,
-6.69658295894055));
#37511=CARTESIAN_POINT('Ctrl Pts',(-10.0036466506002,-36.1646238109885,
-6.9450728886735));
#37512=CARTESIAN_POINT('Ctrl Pts',(-9.83088580791383,-36.1762941168134,
-7.18753231105948));
#37513=CARTESIAN_POINT('Ctrl Pts',(-9.64950806513854,-36.1879644226384,
-7.42330413972284));
#37514=CARTESIAN_POINT('Ctrl Pts',(-9.47625871296853,-36.199111727114,-7.6485099226974));
#37515=CARTESIAN_POINT('Ctrl Pts',(-9.29509606919364,-36.2102590315895,
-7.8676816020831));
#37516=CARTESIAN_POINT('Ctrl Pts',(-9.10646565514324,-36.221406336065,-8.0802681590215));
#37517=CARTESIAN_POINT('Ctrl Pts',(-8.91786728005395,-36.2325517471659,
-8.2928186080371));
#37518=CARTESIAN_POINT('Ctrl Pts',(-8.72180384403198,-36.2436971582667,
-8.49878596821237));
#37519=CARTESIAN_POINT('Ctrl Pts',(-8.51876020628826,-36.2548425693675,
-8.69765340754388));
#37520=CARTESIAN_POINT('Ctrl Pts',(-8.31573910957317,-36.2659867431529,
-8.89649876947028));
#37521=CARTESIAN_POINT('Ctrl Pts',(-8.10573954903184,-36.2771309169383,
-9.08824559786713));
#37522=CARTESIAN_POINT('Ctrl Pts',(-7.88928307487955,-36.2882750907237,
-9.27241407694993));
#37523=CARTESIAN_POINT('Ctrl Pts',(-7.66600988509742,-36.2997702203486,
-9.46238244792694));
#37524=CARTESIAN_POINT('Ctrl Pts',(-7.43586672490532,-36.3112653499736,
-9.64428721563409));
#37525=CARTESIAN_POINT('Ctrl Pts',(-7.19946377540692,-36.3227604795986,
-9.81764592947839));
#37526=CARTESIAN_POINT('Ctrl Pts',(-6.97026615536178,-36.3339052489754,
-9.98572084018279));
#37527=CARTESIAN_POINT('Ctrl Pts',(-6.73518490496334,-36.3450500183522,
-10.1457627683423));
#37528=CARTESIAN_POINT('Ctrl Pts',(-6.49480730688629,-36.3561947877291,
-10.2973748254794));
#37529=CARTESIAN_POINT('Ctrl Pts',(-6.24309451396523,-36.3678650974781,
-10.4561362685081));
#37530=CARTESIAN_POINT('Ctrl Pts',(-5.98557411618706,-36.3795354072272,
-10.6056535064113));
#37531=CARTESIAN_POINT('Ctrl Pts',(-5.7229525669938,-36.3912057169763,-10.7455229824304));
#37532=CARTESIAN_POINT('Ctrl Pts',(-5.46033101780052,-36.4028760267254,
-10.8853924584494));
#37533=CARTESIAN_POINT('Ctrl Pts',(-5.19260861744099,-36.4145463364744,
-11.0156140226206));
#37534=CARTESIAN_POINT('Ctrl Pts',(-4.9205203219068,-36.4262166462235,-11.1358398880238));
#37535=CARTESIAN_POINT('Ctrl Pts',(-4.66062554473769,-36.4373639561281,
-11.2506778836736));
#37536=CARTESIAN_POINT('Ctrl Pts',(-4.39666996201338,-36.4485112660327,
-11.3564306914372));
#37537=CARTESIAN_POINT('Ctrl Pts',(-4.12930845682457,-36.4596585759373,
-11.4528276822101));
#37538=CARTESIAN_POINT('Ctrl Pts',(-3.86199236269481,-36.4708039924835,
-11.5492083000596));
#37539=CARTESIAN_POINT('Ctrl Pts',(-3.59127175189979,-36.4819494090297,
-11.6362361830668));
#37540=CARTESIAN_POINT('Ctrl Pts',(-3.31781968883708,-36.4930948255759,
-11.7136895452443));
#37541=CARTESIAN_POINT('Ctrl Pts',(-3.04439798317911,-36.5042390048086,
-11.7911343089017));
#37542=CARTESIAN_POINT('Ctrl Pts',(-2.76824568734694,-36.5153831840413,
-11.8590066015354));
#37543=CARTESIAN_POINT('Ctrl Pts',(-2.49005036894981,-36.526527363274,-11.9171346979923));
#37544=CARTESIAN_POINT('Ctrl Pts',(-2.20309427787332,-36.5380224888186,
-11.9770933322249));
#37545=CARTESIAN_POINT('Ctrl Pts',(-1.91396469214712,-36.5495176143631,
-12.0266840376984));
#37546=CARTESIAN_POINT('Ctrl Pts',(-1.62342826198514,-36.5610127399077,
-12.065775189692));
#37547=CARTESIAN_POINT('Ctrl Pts',(-1.34174686044864,-36.5721575146694,
-12.1036749135756));
#37548=CARTESIAN_POINT('Ctrl Pts',(-1.05874337738828,-36.5833022894311,
-12.1317055846882));
#37549=CARTESIAN_POINT('Ctrl Pts',(-0.775123413472737,-36.5944470641928,
-12.149799749127));
#37550=CARTESIAN_POINT('Ctrl Pts',(-0.478129494697926,-36.6061173651288,
-12.1687471346687));
#37551=CARTESIAN_POINT('Ctrl Pts',(-0.180459873677726,-36.6177876660647,
-12.1767983435379));
#37552=CARTESIAN_POINT('Ctrl Pts',(0.11707202117144,-36.6294579670007,-12.1739370949524));
#37553=CARTESIAN_POINT('Ctrl Pts',(0.414603916020578,-36.6411282679367,
-12.1710758463669));
#37554=CARTESIAN_POINT('Ctrl Pts',(0.711997749299544,-36.6527985688726,
-12.1573021523303));
#37555=CARTESIAN_POINT('Ctrl Pts',(1.00844175372276,-36.6644688698086,-12.1326623409435));
#37556=CARTESIAN_POINT('Ctrl Pts',(1.29160072405077,-36.6756161703009,-12.1091267540628));
#37557=CARTESIAN_POINT('Ctrl Pts',(1.57397769503675,-36.6867634707932,-12.0756705357027));
#37558=CARTESIAN_POINT('Ctrl Pts',(1.85486813075634,-36.6979107712855,-12.0323694452716));
#37559=CARTESIAN_POINT('Ctrl Pts',(2.13571085696984,-36.7090561783983,-11.9890757095716));
#37560=CARTESIAN_POINT('Ctrl Pts',(2.41506728847831,-36.720201585511,-11.9359404808946));
#37561=CARTESIAN_POINT('Ctrl Pts',(2.69224029849889,-36.7313469926238,-11.8730911065796));
#37562=CARTESIAN_POINT('Ctrl Pts',(2.96938253809598,-36.7424911624267,-11.8102487095019));
#37563=CARTESIAN_POINT('Ctrl Pts',(3.24434158014842,-36.7536353322296,-11.7376943791884));
#37564=CARTESIAN_POINT('Ctrl Pts',(3.51643151935759,-36.7647795020325,-11.655606360017));
#37565=CARTESIAN_POINT('Ctrl Pts',(3.79709037410433,-36.776274634646,-11.5709331467551));
#37566=CARTESIAN_POINT('Ctrl Pts',(4.07469619766536,-36.7877697672594,-11.4761161021925));
#37567=CARTESIAN_POINT('Ctrl Pts',(4.34851283179752,-36.7992648998728,-11.3714065269734));
#37568=CARTESIAN_POINT('Ctrl Pts',(4.61398364177174,-36.8104096653299,-11.2698884587465));
#37569=CARTESIAN_POINT('Ctrl Pts',(4.87589256715123,-36.821554430787,-11.159072070423));
#37570=CARTESIAN_POINT('Ctrl Pts',(5.13358776672708,-36.8326991962441,-11.039235792903));
#37571=CARTESIAN_POINT('Ctrl Pts',(5.40343503015256,-36.8443695124357,-10.9137484279808));
#37572=CARTESIAN_POINT('Ctrl Pts',(5.66866130576691,-36.8560398286273,-10.7783701409865));
#37573=CARTESIAN_POINT('Ctrl Pts',(5.92854455678638,-36.8677101448189,-10.6334758986983));
#37574=CARTESIAN_POINT('Ctrl Pts',(6.18842780780583,-36.8793804610105,-10.4885816564102));
#37575=CARTESIAN_POINT('Ctrl Pts',(6.4429677454689,-36.8910507772021,-10.3341716298738));
#37576=CARTESIAN_POINT('Ctrl Pts',(6.69147375292597,-36.9027210933937,-10.1706749659943));
#37577=CARTESIAN_POINT('Ctrl Pts',(6.93796703319707,-36.9142968880769,-10.008502512276));
#37578=CARTESIAN_POINT('Ctrl Pts',(7.17860021783118,-36.9258726827601,-9.83733979174084));
#37579=CARTESIAN_POINT('Ctrl Pts',(7.41272179941099,-36.9374484774433,-9.65763976210219));
#37580=CARTESIAN_POINT('',(-12.1744999990795,-35.6251260039956,-0.000149711562892353));
#37581=CARTESIAN_POINT('Ctrl Pts',(-12.1744999990795,-35.6251260039956,
-0.000149711562934393));
#37582=CARTESIAN_POINT('Ctrl Pts',(-12.174496426179,-35.6365176701443,-0.290696921273105));
#37583=CARTESIAN_POINT('Ctrl Pts',(-12.1640875501384,-35.647909336293,-0.58120652559487));
#37584=CARTESIAN_POINT('Ctrl Pts',(-12.1433074390434,-35.6593010024416,
-0.870938970808622));
#37585=CARTESIAN_POINT('Ctrl Pts',(-12.1225204619165,-35.670696432552,-1.16076714756995));
#37586=CARTESIAN_POINT('Ctrl Pts',(-12.0913554174435,-35.6820918626624,
-1.44981741179922));
#37587=CARTESIAN_POINT('Ctrl Pts',(-12.0498983619847,-35.6934872927729,
-1.73735422865857));
#37588=CARTESIAN_POINT('Ctrl Pts',(-12.0121118806754,-35.7038737807208,
-1.99943276838512));
#37589=CARTESIAN_POINT('Ctrl Pts',(-11.9657758328564,-35.7142602686687,
-2.26025391982292));
#37590=CARTESIAN_POINT('Ctrl Pts',(-11.9109926366114,-35.7246467566166,
-2.51926669104116));
#37591=CARTESIAN_POINT('Ctrl Pts',(-11.8521965285982,-35.7357940628915,
-2.79725234936639));
#37592=CARTESIAN_POINT('Ctrl Pts',(-11.783655703664,-35.7469413691664,-3.0732202996823));
#37593=CARTESIAN_POINT('Ctrl Pts',(-11.7055335188614,-35.7580886754414,
-3.34648103069664));
#37594=CARTESIAN_POINT('Ctrl Pts',(-11.6274246031012,-35.7692340883479,
-3.61969534841323));
#37595=CARTESIAN_POINT('Ctrl Pts',(-11.5397376498562,-35.7803795012544,
-3.89020310848564));
#37596=CARTESIAN_POINT('Ctrl Pts',(-11.4426862708534,-35.7915249141608,
-4.15732860823185));
#37597=CARTESIAN_POINT('Ctrl Pts',(-11.3456456660616,-35.8026690897533,
-4.42442445289702));
#37598=CARTESIAN_POINT('Ctrl Pts',(-11.2392428024865,-35.8138132653458,
-4.68813853636811));
#37599=CARTESIAN_POINT('Ctrl Pts',(-11.1237403838462,-35.8249574409383,
-4.94781266043789));
#37600=CARTESIAN_POINT('Ctrl Pts',(-11.004600559911,-35.8364525692102,-5.21566444905335));
#37601=CARTESIAN_POINT('Ctrl Pts',(-10.8757788785789,-35.8479476974822,
-5.47921742693672));
#37602=CARTESIAN_POINT('Ctrl Pts',(-10.7376168148967,-35.8594428257542,
-5.73777268514943));
#37603=CARTESIAN_POINT('Ctrl Pts',(-10.6036657578032,-35.8705875969194,
-5.98844750305287));
#37604=CARTESIAN_POINT('Ctrl Pts',(-10.4609353850308,-35.8817323680846,
-6.23442449239448));
#37605=CARTESIAN_POINT('Ctrl Pts',(-10.30978353461,-35.8928771392499,-6.47509179235978));
#37606=CARTESIAN_POINT('Ctrl Pts',(-10.1515040647607,-35.9045474460752,
-6.72710784471055));
#37607=CARTESIAN_POINT('Ctrl Pts',(-9.98398994001832,-35.9162177529005,
-6.97330112872041));
#37608=CARTESIAN_POINT('Ctrl Pts',(-9.80770356017696,-35.9278880597258,
-7.21300222692966));
#37609=CARTESIAN_POINT('Ctrl Pts',(-9.63141718033562,-35.9395583665511,
-7.45270332513889));
#37610=CARTESIAN_POINT('Ctrl Pts',(-9.4463587512404,-35.9512286733765,-7.68591197247079));
#37611=CARTESIAN_POINT('Ctrl Pts',(-9.25304049328369,-35.9628989802018,
-7.91199670624631));
#37612=CARTESIAN_POINT('Ctrl Pts',(-9.06838572400005,-35.9740462863956,
-8.12794953343979));
#37613=CARTESIAN_POINT('Ctrl Pts',(-8.87614002640509,-35.9851935925894,
-8.33746742022859));
#37614=CARTESIAN_POINT('Ctrl Pts',(-8.67677679908099,-35.9963408987832,
-8.54002310470703));
#37615=CARTESIAN_POINT('Ctrl Pts',(-8.47744743357855,-36.0074863116083,
-8.74254438512533));
#37616=CARTESIAN_POINT('Ctrl Pts',(-8.27100313898243,-36.0186317244334,
-8.93810563411376));
#37617=CARTESIAN_POINT('Ctrl Pts',(-8.05795483269958,-36.0297771372585,
-9.1262157636215));
#37618=CARTESIAN_POINT('Ctrl Pts',(-7.84493017808824,-36.0409213127697,
-9.31430500998273));
#37619=CARTESIAN_POINT('Ctrl Pts',(-7.62530317567703,-36.0520654882808,
-9.49494461212312));
#37620=CARTESIAN_POINT('Ctrl Pts',(-7.39961947215846,-36.063209663792,-9.66768234466014));
#37621=CARTESIAN_POINT('Ctrl Pts',(-7.16682852840535,-36.0747047921249,
-9.84585994079197));
#37622=CARTESIAN_POINT('Ctrl Pts',(-6.9275934559246,-36.0861999204578,-10.0156297224767));
#37623=CARTESIAN_POINT('Ctrl Pts',(-6.68254854954543,-36.0976950487907,
-10.1765414131211));
#37624=CARTESIAN_POINT('Ctrl Pts',(-6.44497230785367,-36.1088398198755,
-10.3325487150986));
#37625=CARTESIAN_POINT('Ctrl Pts',(-6.2019353743058,-36.1199845909603,-10.4802297442823));
#37626=CARTESIAN_POINT('Ctrl Pts',(-5.95404475521485,-36.1311293620451,
-10.6192184883304));
#37627=CARTESIAN_POINT('Ctrl Pts',(-5.69446476074719,-36.1427996690021,
-10.7647612988788));
#37628=CARTESIAN_POINT('Ctrl Pts',(-5.429562588848,-36.154469975959,-10.9007721676023));
#37629=CARTESIAN_POINT('Ctrl Pts',(-5.16006460113188,-36.166140282916,-11.0268845809751));
#37630=CARTESIAN_POINT('Ctrl Pts',(-4.89056661341578,-36.1778105898729,
-11.1529969943479));
#37631=CARTESIAN_POINT('Ctrl Pts',(-4.61647311747857,-36.1894808968299,
-11.2692108181213));
#37632=CARTESIAN_POINT('Ctrl Pts',(-4.33853605764074,-36.2011512037868,
-11.3752167067951));
#37633=CARTESIAN_POINT('Ctrl Pts',(-4.07305464777408,-36.2122985101097,
-11.4764719794663));
#37634=CARTESIAN_POINT('Ctrl Pts',(-3.80398730860846,-36.2234458164327,
-11.5684443772484));
#37635=CARTESIAN_POINT('Ctrl Pts',(-3.53200203188287,-36.2345931227556,
-11.6508974717305));
#37636=CARTESIAN_POINT('Ctrl Pts',(-3.26006295181857,-36.2457385357101,
-11.7333365615659));
#37637=CARTESIAN_POINT('Ctrl Pts',(-2.98520717886023,-36.2568839486646,
-11.8062594987885));
#37638=CARTESIAN_POINT('Ctrl Pts',(-2.70811833795219,-36.2680293616191,
-11.8694795723169));
#37639=CARTESIAN_POINT('Ctrl Pts',(-2.43106025821149,-36.2791735372596,
-11.9326926274346));
#37640=CARTESIAN_POINT('Ctrl Pts',(-2.1517698655459,-36.2903177129001,-11.9862049104721));
#37641=CARTESIAN_POINT('Ctrl Pts',(-1.87094268199846,-36.3014618885405,
-12.0298804537151));
#37642=CARTESIAN_POINT('Ctrl Pts',(-1.5812716833385,-36.3129570167765,-12.0749314280132));
#37643=CARTESIAN_POINT('Ctrl Pts',(-1.28996582371931,-36.3244521450124,
-12.1095160101662));
#37644=CARTESIAN_POINT('Ctrl Pts',(-0.997797531322615,-36.3359472732484,
-12.1335423655455));
#37645=CARTESIAN_POINT('Ctrl Pts',(-0.714534160316956,-36.3470920444607,
-12.1568364278884));
#37646=CARTESIAN_POINT('Ctrl Pts',(-0.430460427915619,-36.358236815673,
-12.1702063130348));
#37647=CARTESIAN_POINT('Ctrl Pts',(-0.146284477231075,-36.3693815868853,
-12.1736211170597));
#37648=CARTESIAN_POINT('Ctrl Pts',(0.151291888549954,-36.3810518936331,
-12.1771969473476));
#37649=CARTESIAN_POINT('Ctrl Pts',(0.448980027019182,-36.3927222003809,
-12.169856231212));
#37650=CARTESIAN_POINT('Ctrl Pts',(0.745966753667841,-36.4043925071286,
-12.1516247412608));
#37651=CARTESIAN_POINT('Ctrl Pts',(1.04295348031647,-36.4160628138764,-12.1333932513097));
#37652=CARTESIAN_POINT('Ctrl Pts',(1.33923846081193,-36.4277331206241,-12.1042710168617));
#37653=CARTESIAN_POINT('Ctrl Pts',(1.63401340472503,-36.4394034273719,-12.0643462501363));
#37654=CARTESIAN_POINT('Ctrl Pts',(1.91557811671966,-36.4505507335666,-12.0262106973134));
#37655=CARTESIAN_POINT('Ctrl Pts',(2.19584925314808,-36.4616980397613,-11.9782081635445));
#37656=CARTESIAN_POINT('Ctrl Pts',(2.47412713324821,-36.4728453459559,-11.9204507120547));
#37657=CARTESIAN_POINT('Ctrl Pts',(2.75235774788912,-36.4839907587822,-11.8627030706599));
#37658=CARTESIAN_POINT('Ctrl Pts',(3.02859552104343,-36.4951361716085,-11.7952038736759));
#37659=CARTESIAN_POINT('Ctrl Pts',(3.30215083685498,-36.5062815844348,-11.7181163204953));
#37660=CARTESIAN_POINT('Ctrl Pts',(3.57567578378372,-36.5174257599474,-11.6410373252286));
#37661=CARTESIAN_POINT('Ctrl Pts',(3.84651861133585,-36.52856993546,-11.5543721716479));
#37662=CARTESIAN_POINT('Ctrl Pts',(4.11400354010584,-36.5397141109726,-11.4583343083538));
#37663=CARTESIAN_POINT('Ctrl Pts',(4.38991211491443,-36.5512092393046,-11.3592720168407));
#37664=CARTESIAN_POINT('Ctrl Pts',(4.66224758709874,-36.5627043676366,-11.250237209273));
#37665=CARTESIAN_POINT('Ctrl Pts',(4.93028776824498,-36.5741994959687,-11.1315188888262));
#37666=CARTESIAN_POINT('Ctrl Pts',(5.19015841733053,-36.5853442670556,-11.0164189554471));
#37667=CARTESIAN_POINT('Ctrl Pts',(5.44599147331901,-36.5964890381425,-10.8922171642219));
#37668=CARTESIAN_POINT('Ctrl Pts',(5.69715035220492,-36.6076338092294,-10.7592252562334));
#37669=CARTESIAN_POINT('Ctrl Pts',(5.96015272238509,-36.619304116184,-10.6199620648587));
#37670=CARTESIAN_POINT('Ctrl Pts',(6.21802920235262,-36.6309744231386,-10.4710599556509));
#37671=CARTESIAN_POINT('Ctrl Pts',(6.47007809708769,-36.6426447300932,-10.3129307021615));
#37672=CARTESIAN_POINT('Ctrl Pts',(6.72212699182275,-36.6543150370478,-10.1548014486722));
#37673=CARTESIAN_POINT('Ctrl Pts',(6.96834802179005,-36.6659853440024,-9.98744523663738));
#37674=CARTESIAN_POINT('Ctrl Pts',(7.20807366931145,-36.677655650957,-9.81132632358027));
#37675=CARTESIAN_POINT('Ctrl Pts',(7.27682267471017,-36.6810024851574,-9.76081858596533));
#37676=CARTESIAN_POINT('Ctrl Pts',(7.34504387489234,-36.6843493193577,-9.70958595586962));
#37677=CARTESIAN_POINT('Ctrl Pts',(7.41272179941099,-36.6876961535581,-9.65763976210219));
#37678=CARTESIAN_POINT('Ctrl Pts',(7.412721799411,-33.6876951030527,-9.65763976210218));
#37679=CARTESIAN_POINT('Ctrl Pts',(7.63818831033701,-33.6988400412174,-9.48458293230233));
#37680=CARTESIAN_POINT('Ctrl Pts',(7.85759515882196,-33.7099849793821,-9.30362458373371));
#37681=CARTESIAN_POINT('Ctrl Pts',(8.07039566856871,-33.7211299175467,-9.11521606999788));
#37682=CARTESIAN_POINT('Ctrl Pts',(8.28319341563403,-33.7322747110223,-8.92681000227451));
#37683=CARTESIAN_POINT('Ctrl Pts',(8.48938479699339,-33.7434195044979,-8.73095414112008));
#37684=CARTESIAN_POINT('Ctrl Pts',(8.68845788705469,-33.7545642979734,-8.52813870635775));
#37685=CARTESIAN_POINT('Ctrl Pts',(8.88757719156055,-33.7657116786919,-8.32527618837254));
#37686=CARTESIAN_POINT('Ctrl Pts',(9.079574714239,-33.7768590594104,-8.11545105737663));
#37687=CARTESIAN_POINT('Ctrl Pts',(9.26397579995409,-33.7880064401288,-7.8991899982128));
#37688=CARTESIAN_POINT('Ctrl Pts',(9.43282943823787,-33.7982139493978,-7.70116260310658));
#37689=CARTESIAN_POINT('Ctrl Pts',(9.59531392857967,-33.8084214586668,-7.49773932359984));
#37690=CARTESIAN_POINT('Ctrl Pts',(9.75109440402036,-33.8186289679358,-7.28934895404814));
#37691=CARTESIAN_POINT('Ctrl Pts',(9.92121745963441,-33.8297762741829,-7.06177225466792));
#37692=CARTESIAN_POINT('Ctrl Pts',(10.0833954685513,-33.8409235804299,-6.82820331985483));
#37693=CARTESIAN_POINT('Ctrl Pts',(10.2372180184084,-33.852070886677,-6.58921979399485));
#37694=CARTESIAN_POINT('Ctrl Pts',(10.3910144415251,-33.8632162995555,-6.35027685945625));
#37695=CARTESIAN_POINT('Ctrl Pts',(10.5364580946448,-33.874361712434,-6.10592139420259));
#37696=CARTESIAN_POINT('Ctrl Pts',(10.6731820964192,-33.8855071253125,-5.85675970026745));
#37697=CARTESIAN_POINT('Ctrl Pts',(10.8098909197055,-33.8966513008771,-5.60762566715101));
#37698=CARTESIAN_POINT('Ctrl Pts',(10.9378818963315,-33.9077954764416,-5.35368670459258));
#37699=CARTESIAN_POINT('Ctrl Pts',(11.0568336864415,-33.9189396520062,-5.09557446029123));
#37700=CARTESIAN_POINT('Ctrl Pts',(11.1795315100773,-33.9304347802991,-4.82933373705164));
#37701=CARTESIAN_POINT('Ctrl Pts',(11.2926114639303,-33.941929908592,-4.55865288790692));
#37702=CARTESIAN_POINT('Ctrl Pts',(11.3957735795932,-33.9534250368849,-4.28424961605236));
#37703=CARTESIAN_POINT('Ctrl Pts',(11.4957914427987,-33.9645698080224,-4.01820981325164));
#37704=CARTESIAN_POINT('Ctrl Pts',(11.5864869838508,-33.97571457916,-3.74867139848463));
#37705=CARTESIAN_POINT('Ctrl Pts',(11.6676364475165,-33.9868593502975,-3.47630694539264));
#37706=CARTESIAN_POINT('Ctrl Pts',(11.7526125436312,-33.9985296571681,-3.19109904753701));
#37707=CARTESIAN_POINT('Ctrl Pts',(11.8271205113252,-34.0101999640387,-2.90279247716342));
#37708=CARTESIAN_POINT('Ctrl Pts',(11.8909623210325,-34.0218702709092,-2.61217635885952));
#37709=CARTESIAN_POINT('Ctrl Pts',(11.9548041307399,-34.0335405777798,-2.32156024055564));
#37710=CARTESIAN_POINT('Ctrl Pts',(12.0079797190489,-34.0452108846504,-2.02863490389215));
#37711=CARTESIAN_POINT('Ctrl Pts',(12.0503524473524,-34.056881191521,-1.73420187538456));
#37712=CARTESIAN_POINT('Ctrl Pts',(12.0908262570107,-34.0680284977683,-1.45296375761318));
#37713=CARTESIAN_POINT('Ctrl Pts',(12.1214562644126,-34.0791758040156,-1.17026611606645));
#37714=CARTESIAN_POINT('Ctrl Pts',(12.142158528628,-34.0903231102629,-0.886812559488088));
#37715=CARTESIAN_POINT('Ctrl Pts',(12.1628572765665,-34.1014685231416,-0.603407147460176));
#37716=CARTESIAN_POINT('Ctrl Pts',(12.1736316284451,-34.1126139360204,-0.319246342673114));
#37717=CARTESIAN_POINT('Ctrl Pts',(12.1744495802706,-34.1237593488991,-0.0350380856780686));
#37718=CARTESIAN_POINT('Ctrl Pts',(12.1752674412908,-34.1349035244639,0.249138619785386));
#37719=CARTESIAN_POINT('Ctrl Pts',(12.1661311086289,-34.1460477000287,0.533362500259884));
#37720=CARTESIAN_POINT('Ctrl Pts',(12.1470606956327,-34.1571918755935,0.816925153619469));
#37721=CARTESIAN_POINT('Ctrl Pts',(12.1273897165896,-34.1686870038862,1.10941777099075));
#37722=CARTESIAN_POINT('Ctrl Pts',(12.0971488397799,-34.1801821321789,1.40120654292002));
#37723=CARTESIAN_POINT('Ctrl Pts',(12.0564181252866,-34.1916772604716,1.69151773217481));
#37724=CARTESIAN_POINT('Ctrl Pts',(12.0169288321053,-34.2028220316094,1.97298059892988));
#37725=CARTESIAN_POINT('Ctrl Pts',(11.9675797055986,-34.2139668027472,2.25305434264466));
#37726=CARTESIAN_POINT('Ctrl Pts',(11.9084961294965,-34.225111573885,2.53104132399424));
#37727=CARTESIAN_POINT('Ctrl Pts',(11.8466264458957,-34.2367818807552,2.82213688245413));
#37728=CARTESIAN_POINT('Ctrl Pts',(11.7740822255187,-34.2484521876253,3.11094382810151));
#37729=CARTESIAN_POINT('Ctrl Pts',(11.6910672154904,-34.2601224944955,3.39667449321921));
#37730=CARTESIAN_POINT('Ctrl Pts',(11.608052205462,-34.2717928013657,3.68240515833693));
#37731=CARTESIAN_POINT('Ctrl Pts',(11.5145665078164,-34.2834631082358,3.96505922319547));
#37732=CARTESIAN_POINT('Ctrl Pts',(11.4108737097382,-34.295133415106,4.24386750858299));
#37733=CARTESIAN_POINT('Ctrl Pts',(11.3118278672755,-34.3062807213527,4.51018110049645));
#37734=CARTESIAN_POINT('Ctrl Pts',(11.2034400892115,-34.3174280275994,4.77306556836597));
#37735=CARTESIAN_POINT('Ctrl Pts',(11.0859733768434,-34.3285753338461,5.03186292916634));
#37736=CARTESIAN_POINT('Ctrl Pts',(10.9685266161816,-34.3397207467242,5.29061633326782));
#37737=CARTESIAN_POINT('Ctrl Pts',(10.8420041101378,-34.3508661596023,5.54528377345437));
#37738=CARTESIAN_POINT('Ctrl Pts',(10.7067165369335,-34.3620115724805,5.79522831713764));
#37739=CARTESIAN_POINT('Ctrl Pts',(10.5714439827516,-34.3731557480446,6.04514511309366));
#37740=CARTESIAN_POINT('Ctrl Pts',(10.4274084313955,-34.3842999236088,6.29033982499244));
#37741=CARTESIAN_POINT('Ctrl Pts',(10.2749665443453,-34.395444099173,6.53020005532642));
#37742=CARTESIAN_POINT('Ctrl Pts',(10.117723952571,-34.4069392274662,6.77761397161364));
#37743=CARTESIAN_POINT('Ctrl Pts',(9.95153713121388,-34.4184343557593,7.01935171891168));
#37744=CARTESIAN_POINT('Ctrl Pts',(9.77684664447996,-34.4299294840525,7.25477221836227));
#37745=CARTESIAN_POINT('Ctrl Pts',(9.60748050563951,-34.4410742551897,7.48301739496749));
#37746=CARTESIAN_POINT('Ctrl Pts',(9.43012155403504,-34.4522190263269,7.7053244809599));
#37747=CARTESIAN_POINT('Ctrl Pts',(9.24521373484962,-34.4633637974641,7.92114090563651));
#37748=CARTESIAN_POINT('Ctrl Pts',(9.05158652023803,-34.4750341043353,8.14713423226626));
#37749=CARTESIAN_POINT('Ctrl Pts',(8.84968157512732,-34.4867044112064,8.36600978804986));
#37750=CARTESIAN_POINT('Ctrl Pts',(8.64005473522879,-34.4983747180776,8.5771734517993));
#37751=CARTESIAN_POINT('Ctrl Pts',(8.43042789533026,-34.5100450249488,8.78833711554873));
#37752=CARTESIAN_POINT('Ctrl Pts',(8.21307940324054,-34.52171533182,8.99178865534857));
#37753=CARTESIAN_POINT('Ctrl Pts',(7.98860879055077,-34.5333856386912,9.18697882013097));
#37754=CARTESIAN_POINT('Ctrl Pts',(7.77419774798598,-34.5445329449391,9.37342160757606));
#37755=CARTESIAN_POINT('Ctrl Pts',(7.55322486774204,-34.5556802511869,9.55238288856828));
#37756=CARTESIAN_POINT('Ctrl Pts',(7.32623595483955,-34.5668275574348,9.72341076906742));
#37757=CARTESIAN_POINT('Ctrl Pts',(7.09928559597489,-34.5779729703142,9.89440960050293));
#37758=CARTESIAN_POINT('Ctrl Pts',(6.8663214574821,-34.5891183831935,10.0574775612436));
#37759=CARTESIAN_POINT('Ctrl Pts',(6.62792113425293,-34.6002637960728,10.21220405633));
#37760=CARTESIAN_POINT('Ctrl Pts',(6.38954727716309,-34.6114079716382,10.3669133743719));
#37761=CARTESIAN_POINT('Ctrl Pts',(6.14573866412767,-34.6225521472036,10.5132829307161));
#37762=CARTESIAN_POINT('Ctrl Pts',(5.89710152521148,-34.6336963227689,10.6509456787343));
#37763=CARTESIAN_POINT('Ctrl Pts',(5.64063429770763,-34.6451914510612,10.7929437063366));
#37764=CARTESIAN_POINT('Ctrl Pts',(5.37902975093787,-34.6566865793535,10.9256774968982));
#37765=CARTESIAN_POINT('Ctrl Pts',(5.11298151220427,-34.6681817076457,11.0487949707585));
#37766=CARTESIAN_POINT('Ctrl Pts',(4.85504209151592,-34.6793264787841,11.1681599777786));
#37767=CARTESIAN_POINT('Ctrl Pts',(4.59292609736638,-34.6904712499225,11.2784860573086));
#37768=CARTESIAN_POINT('Ctrl Pts',(4.32728777084149,-34.7016160210608,11.3795004634793));
#37769=CARTESIAN_POINT('Ctrl Pts',(4.04912317254769,-34.71328632793,11.4852782406621));
#37770=CARTESIAN_POINT('Ctrl Pts',(3.76709635207613,-34.7249566347993,11.5808449099813));
#37771=CARTESIAN_POINT('Ctrl Pts',(3.48197968126964,-34.7366269416685,11.6659447859668));
#37772=CARTESIAN_POINT('Ctrl Pts',(3.19686301046314,-34.7482972485377,11.7510446619523));
#37773=CARTESIAN_POINT('Ctrl Pts',(2.9086568133186,-34.759967555407,11.8256776570603));
#37774=CARTESIAN_POINT('Ctrl Pts',(2.61815035720158,-34.7716378622762,11.8896483950151));
#37775=CARTESIAN_POINT('Ctrl Pts',(2.34066284388209,-34.7827851685224,11.950752307257));
#37776=CARTESIAN_POINT('Ctrl Pts',(2.06099383559946,-34.7939324747685,12.0021468563789));
#37777=CARTESIAN_POINT('Ctrl Pts',(1.77983883484186,-34.8050797810147,12.043696441375));
#37778=CARTESIAN_POINT('Ctrl Pts',(1.49873158822519,-34.8162251938923,12.0852389691794));
#37779=CARTESIAN_POINT('Ctrl Pts',(1.21613911682261,-34.8273706067699,12.1169398323548));
#37780=CARTESIAN_POINT('Ctrl Pts',(0.932765073298876,-34.8385160196475,
12.1387149059542));
#37781=CARTESIAN_POINT('Ctrl Pts',(0.649422488696312,-34.8496601952111,
12.160487562182));
#37782=CARTESIAN_POINT('Ctrl Pts',(0.365298771126767,-34.8608043707748,
12.1723366087547));
#37783=CARTESIAN_POINT('Ctrl Pts',(0.0811018770416422,-34.8719485463384,
12.174229862112));
#37784=CARTESIAN_POINT('Ctrl Pts',(-0.212044954636546,-34.883443674632,
12.1761827378641));
#37785=CARTESIAN_POINT('Ctrl Pts',(-0.505269349828249,-34.8949388029255,
12.1675425913307));
#37786=CARTESIAN_POINT('Ctrl Pts',(-0.797793774022385,-34.9064339312191,
12.1483322042217));
#37787=CARTESIAN_POINT('Ctrl Pts',(-1.08140241902979,-34.9175787023558,
12.1297073257247));
#37788=CARTESIAN_POINT('Ctrl Pts',(-1.36435285121784,-34.9287234734924,
12.1011470191103));
#37789=CARTESIAN_POINT('Ctrl Pts',(-1.64594008431267,-34.9398682446291,
12.0627248782708));
#37790=CARTESIAN_POINT('Ctrl Pts',(-1.94080566577381,-34.9515385515011,
12.022490927409));
#37791=CARTESIAN_POINT('Ctrl Pts',(-2.23417607541674,-34.9632088583732,
11.9714427292178));
#37792=CARTESIAN_POINT('Ctrl Pts',(-2.52525076469805,-34.9748791652452,
11.9097253883283));
#37793=CARTESIAN_POINT('Ctrl Pts',(-2.81632545397939,-34.9865494721172,
11.8480080474388));
#37794=CARTESIAN_POINT('Ctrl Pts',(-3.10510409651557,-34.9982197789893,
11.7756216420282));
#37795=CARTESIAN_POINT('Ctrl Pts',(-3.39080016893301,-35.0098900858613,
11.6927723173063));
#37796=CARTESIAN_POINT('Ctrl Pts',(-3.66369287414124,-35.0210373921087,
11.6136358554125));
#37797=CARTESIAN_POINT('Ctrl Pts',(-3.93385472728386,-35.0321846983561,
11.5249300100742));
#37798=CARTESIAN_POINT('Ctrl Pts',(-4.2006101415968,-35.0433320046035,11.4268685425323));
#37799=CARTESIAN_POINT('Ctrl Pts',(-4.46732024753662,-35.0544774174824,
11.3288237307182));
#37800=CARTESIAN_POINT('Ctrl Pts',(-4.73062481951651,-35.0656228303613,
11.2214265612428));
#37801=CARTESIAN_POINT('Ctrl Pts',(-4.98986574788565,-35.0767682432401,
11.1049398948431));
#37802=CARTESIAN_POINT('Ctrl Pts',(-5.24907789648447,-35.087912418805,10.988466160273));
#37803=CARTESIAN_POINT('Ctrl Pts',(-5.50422705905216,-35.0990565943699,
10.8629050530432));
#37804=CARTESIAN_POINT('Ctrl Pts',(-5.75467620310833,-35.1102007699348,
10.7285671013131));
#37805=CARTESIAN_POINT('Ctrl Pts',(-6.01301249949392,-35.1216958982274,
10.5899985745779));
#37806=CARTESIAN_POINT('Ctrl Pts',(-6.26634768811444,-35.1331910265201,
10.4420915758947));
#37807=CARTESIAN_POINT('Ctrl Pts',(-6.51400994570973,-35.1446861548127,
10.2852381925357));
#37808=CARTESIAN_POINT('Ctrl Pts',(-6.75412376698444,-35.1558309259506,
10.1331655044164));
#37809=CARTESIAN_POINT('Ctrl Pts',(-6.98890510846621,-35.1669756970884,
9.97268385469132));
#37810=CARTESIAN_POINT('Ctrl Pts',(-7.21777016470931,-35.1781204682263,
9.80419522956536));
#37811=CARTESIAN_POINT('Ctrl Pts',(-7.45742743583133,-35.1897907750963,
9.62776146210592));
#37812=CARTESIAN_POINT('Ctrl Pts',(-7.6905967708411,-35.2014610819663,9.44254759390732));
#37813=CARTESIAN_POINT('Ctrl Pts',(-7.91664467542025,-35.2131313888364,
9.24906413282664));
#37814=CARTESIAN_POINT('Ctrl Pts',(-8.14269257999939,-35.2248016957064,
9.05558067174598));
#37815=CARTESIAN_POINT('Ctrl Pts',(-8.36161880497333,-35.2364720025764,
8.85382784261634));
#37816=CARTESIAN_POINT('Ctrl Pts',(-8.57283138154773,-35.2481423094464,
8.64436303920366));
#37817=CARTESIAN_POINT('Ctrl Pts',(-8.7745785421954,-35.2592896156963,8.44428532588983));
#37818=CARTESIAN_POINT('Ctrl Pts',(-8.96934848056512,-35.2704369219463,
8.23711190810849));
#37819=CARTESIAN_POINT('Ctrl Pts',(-9.15665028193266,-35.2815842281962,
8.02335377908656));
#37820=CARTESIAN_POINT('Ctrl Pts',(-9.34392027011314,-35.2927296410776,
7.80963195685556));
#37821=CARTESIAN_POINT('Ctrl Pts',(-9.52372447804811,-35.303875053959,7.58932785684307));
#37822=CARTESIAN_POINT('Ctrl Pts',(-9.69561083324766,-35.3150204668404,
7.36298722124455));
#37823=CARTESIAN_POINT('Ctrl Pts',(-9.8674781063922,-35.3261646424078,7.13667171297192));
#37824=CARTESIAN_POINT('Ctrl Pts',(-10.0314291207498,-35.3373088179753,
6.90432121967417));
#37825=CARTESIAN_POINT('Ctrl Pts',(-10.1870531218382,-35.3484529935428,
6.66651325228162));
#37826=CARTESIAN_POINT('Ctrl Pts',(-10.3475780388049,-35.3599481218335,
6.42121622899009));
#37827=CARTESIAN_POINT('Ctrl Pts',(-10.4992428040734,-35.3714432501243,
6.17011267067247));
#37828=CARTESIAN_POINT('Ctrl Pts',(-10.6416451441391,-35.382938378415,5.91386835127568));
#37829=CARTESIAN_POINT('Ctrl Pts',(-10.7797072387721,-35.3940831495554,
5.6654340386276));
#37830=CARTESIAN_POINT('Ctrl Pts',(-10.9090630261503,-35.4052279206958,
5.41216793644504));
#37831=CARTESIAN_POINT('Ctrl Pts',(-11.0293922551297,-35.4163726918363,
5.15470239029231));
#37832=CARTESIAN_POINT('Ctrl Pts',(-11.1553956525465,-35.4280429987021,
4.8850959629249));
#37833=CARTESIAN_POINT('Ctrl Pts',(-11.2715005718733,-35.439713305568,4.61088479720244));
#37834=CARTESIAN_POINT('Ctrl Pts',(-11.3773950641872,-35.4513836124339,
4.33282030592177));
#37835=CARTESIAN_POINT('Ctrl Pts',(-11.4832895565011,-35.4630539192998,
4.05475581464107));
#37836=CARTESIAN_POINT('Ctrl Pts',(-11.578973510603,-35.4747242261657,3.77283831446075));
#37837=CARTESIAN_POINT('Ctrl Pts',(-11.6641938765588,-35.4863945330316,
3.48784051528297));
#37838=CARTESIAN_POINT('Ctrl Pts',(-11.7486157263752,-35.4979554889427,
3.20551314986525));
#37839=CARTESIAN_POINT('Ctrl Pts',(-11.8227942500949,-35.5095164448538,
2.92007971671269));
#37840=CARTESIAN_POINT('Ctrl Pts',(-11.8865239621894,-35.521077400765,2.63229906095355));
#37841=CARTESIAN_POINT('Ctrl Pts',(-11.9482806334632,-35.5322804351166,
2.35342795401509));
#37842=CARTESIAN_POINT('Ctrl Pts',(-12.0002256656454,-35.5434834694682,
2.07235304358251));
#37843=CARTESIAN_POINT('Ctrl Pts',(-12.042223537602,-35.5546865038198,1.78977722647935));
#37844=CARTESIAN_POINT('Ctrl Pts',(-12.0862340710423,-35.5664264205107,
1.49365954554348));
#37845=CARTESIAN_POINT('Ctrl Pts',(-12.119320691996,-35.5781663372016,1.19589388457444));
#37846=CARTESIAN_POINT('Ctrl Pts',(-12.1413881016093,-35.5899062538925,
0.897298844366037));
#37847=CARTESIAN_POINT('Ctrl Pts',(-12.1634555112226,-35.6016461705834,
0.598703804157665));
#37848=CARTESIAN_POINT('Ctrl Pts',(-12.1745036811867,-35.6133860872742,
0.299279713519359));
#37849=CARTESIAN_POINT('Ctrl Pts',(-12.1744999990795,-35.6251260039651,
-0.00014971078451594));
#37850=CARTESIAN_POINT('Origin',(0.,-13.3748739960349,0.));
#37851=CARTESIAN_POINT('',(7.41272179941102,-30.6876856710377,-9.65763976210216));
#37852=CARTESIAN_POINT('',(7.41333450932786,-30.9374378643274,-9.65843860956001));
#37853=CARTESIAN_POINT('',(7.41272179941101,-13.3748739960349,-9.65763976210217));
#37854=CARTESIAN_POINT('',(-12.1744999985554,-32.8748739960349,0.000187550598588881));
#37855=CARTESIAN_POINT('Ctrl Pts',(7.41333450932841,-30.9374378643275,-9.65843860955958));
#37856=CARTESIAN_POINT('Ctrl Pts',(7.47386574430169,-30.9404304108071,-9.61201282177837));
#37857=CARTESIAN_POINT('Ctrl Pts',(9.12856187469929,-31.0228403651483,-8.31759967269045));
#37858=CARTESIAN_POINT('Ctrl Pts',(11.6976034309138,-31.1846677273513,-4.92316720896363));
#37859=CARTESIAN_POINT('Ctrl Pts',(12.6271934885173,-31.4229199509364,1.27494548820119));
#37860=CARTESIAN_POINT('Ctrl Pts',(10.4773717109103,-31.6611721745215,7.16213539565936));
#37861=CARTESIAN_POINT('Ctrl Pts',(5.77241822665602,-31.8994243981066,11.3026850443117));
#37862=CARTESIAN_POINT('Ctrl Pts',(-0.340263191846742,-32.1376766216917,
12.6868326368173));
#37863=CARTESIAN_POINT('Ctrl Pts',(-6.36996413642198,-32.3759288452768,
10.9770241092494));
#37864=CARTESIAN_POINT('Ctrl Pts',(-10.8462127664019,-32.6141810688619,
6.59023292610109));
#37865=CARTESIAN_POINT('Ctrl Pts',(-12.1244826930503,-32.7804961191146,
2.40607098746999));
#37866=CARTESIAN_POINT('Ctrl Pts',(-12.1754508005637,-32.8673937615056,
0.190879886591904));
#37867=CARTESIAN_POINT('Ctrl Pts',(-12.175309711376,-32.8748739960349,0.000187563072374733));
#37868=CARTESIAN_POINT('Ctrl Pts',(-12.1744999985554,-32.8748739960349,
0.000187550598588881));
#37869=CARTESIAN_POINT('Ctrl Pts',(-12.1745043615588,-32.8859843814439,
-0.283028740965722));
#37870=CARTESIAN_POINT('Ctrl Pts',(-12.1646216592697,-32.8970947668528,
-0.566289459754149));
#37871=CARTESIAN_POINT('Ctrl Pts',(-12.1448686657604,-32.9082051522618,
-0.848890653400877));
#37872=CARTESIAN_POINT('Ctrl Pts',(-12.125118898305,-32.9193137231254,-1.13144569269124));
#37873=CARTESIAN_POINT('Ctrl Pts',(-12.0955020767017,-32.930422293989,-1.4133411523803));
#37874=CARTESIAN_POINT('Ctrl Pts',(-12.0560869992745,-32.9415308648526,
-1.69387618081272));
#37875=CARTESIAN_POINT('Ctrl Pts',(-12.0166757019596,-32.9526383703461,
-1.97438430446705));
#37876=CARTESIAN_POINT('Ctrl Pts',(-11.9674680629165,-32.9637458758396,
-2.2535319898437));
#37877=CARTESIAN_POINT('Ctrl Pts',(-11.9085845275246,-32.9748533813331,
-2.5306253774118));
#37878=CARTESIAN_POINT('Ctrl Pts',(-11.849696245945,-32.9859617821245,-2.80774109952985));
#37879=CARTESIAN_POINT('Ctrl Pts',(-11.7811305632598,-32.9970701829159,
-3.08280192803896));
#37880=CARTESIAN_POINT('Ctrl Pts',(-11.703058959395,-33.0081785837073,-3.35512462405274));
#37881=CARTESIAN_POINT('Ctrl Pts',(-11.6249866141567,-33.0192870899849,
-3.62744990606199));
#37882=CARTESIAN_POINT('Ctrl Pts',(-11.5374082443903,-33.0303955962625,
-3.89703674452342));
#37883=CARTESIAN_POINT('Ctrl Pts',(-11.4405453455313,-33.0415041025401,
-4.16321659859816));
#37884=CARTESIAN_POINT('Ctrl Pts',(-11.3436617578851,-33.0526149814652,
-4.4294533055898));
#37885=CARTESIAN_POINT('Ctrl Pts',(-11.2374897710976,-33.0637258603903,
-4.6922813200952));
#37886=CARTESIAN_POINT('Ctrl Pts',(-11.1222997533272,-33.0748367393155,
-4.95105023678181));
#37887=CARTESIAN_POINT('Ctrl Pts',(-11.067529982669,-33.0801196648877,-5.07408793132099));
#37888=CARTESIAN_POINT('Ctrl Pts',(-11.0107221639337,-33.0854025904599,
-5.19620826044135));
#37889=CARTESIAN_POINT('Ctrl Pts',(-10.9519091180938,-33.0906855160321,
-5.31734303191104));
#37890=CARTESIAN_POINT('Ctrl Pts',(-10.8278098809659,-33.1018328222794,
-5.5729450418798));
#37891=CARTESIAN_POINT('Ctrl Pts',(-10.6947401199187,-33.1129801285267,
-5.82423887901939));
#37892=CARTESIAN_POINT('Ctrl Pts',(-10.5530246517763,-33.124127434774,-6.07059477720272));
#37893=CARTESIAN_POINT('Ctrl Pts',(-10.4113332539878,-33.1352728476528,
-6.31690883186865));
#37894=CARTESIAN_POINT('Ctrl Pts',(-10.2609992138668,-33.1464182605315,
-6.55828639092668));
#37895=CARTESIAN_POINT('Ctrl Pts',(-10.1023927896335,-33.1575636734103,
-6.7941232086239));
#37896=CARTESIAN_POINT('Ctrl Pts',(-9.94380397317836,-33.168707848975,-7.02993384476881));
#37897=CARTESIAN_POINT('Ctrl Pts',(-9.77694475525955,-33.1798520245398,
-7.26020474653669));
#37898=CARTESIAN_POINT('Ctrl Pts',(-9.60222881583929,-33.1909962001045,
-7.48436049494315));
#37899=CARTESIAN_POINT('Ctrl Pts',(-9.42201071655001,-33.2024913283972,
-7.71557536324092));
#37900=CARTESIAN_POINT('Ctrl Pts',(-9.2334332035449,-33.21398645669,-7.94028343973844));
#37901=CARTESIAN_POINT('Ctrl Pts',(-9.03699622097056,-33.2254815849827,
-8.15788879258377));
#37902=CARTESIAN_POINT('Ctrl Pts',(-8.84654639230963,-33.2366263561204,
-8.36886180602542));
#37903=CARTESIAN_POINT('Ctrl Pts',(-8.64870928031278,-33.2477711272582,
-8.57315844163609));
#37904=CARTESIAN_POINT('Ctrl Pts',(-8.44397971682008,-33.258915898396,-8.77027119261035));
#37905=CARTESIAN_POINT('Ctrl Pts',(-8.22959605637275,-33.2705862052662,
-8.97667886697739));
#37906=CARTESIAN_POINT('Ctrl Pts',(-8.00765450035677,-33.2822565121364,
-9.1752086165817));
#37907=CARTESIAN_POINT('Ctrl Pts',(-7.77876523658056,-33.2939268190066,
-9.36532229259441));
#37908=CARTESIAN_POINT('Ctrl Pts',(-7.54987597280433,-33.3055971258768,
-9.55543596860713));
#37909=CARTESIAN_POINT('Ctrl Pts',(-7.31403926496306,-33.317267432747,-9.73713336341621));
#37910=CARTESIAN_POINT('Ctrl Pts',(-7.07190449795741,-33.3289377396172,
-9.90992517740522));
#37911=CARTESIAN_POINT('Ctrl Pts',(-6.8406209138327,-33.3400850458639,-10.0749733881227));
#37912=CARTESIAN_POINT('Ctrl Pts',(-6.60352227774398,-33.3512323521105,
-10.2319459674008));
#37913=CARTESIAN_POINT('Ctrl Pts',(-6.36119516972689,-33.3623796583572,
-10.3804453788189));
#37914=CARTESIAN_POINT('Ctrl Pts',(-6.1189092209383,-33.3735250712353,-10.5289195676309));
#37915=CARTESIAN_POINT('Ctrl Pts',(-5.87139680057618,-33.3846704841134,
-10.6689233225553));
#37916=CARTESIAN_POINT('Ctrl Pts',(-5.61927217655415,-33.3958158969915,
-10.8001032613491));
#37917=CARTESIAN_POINT('Ctrl Pts',(-5.36717554228243,-33.4069600725556,
-10.9312686371318));
#37918=CARTESIAN_POINT('Ctrl Pts',(-5.11046796335894,-33.4181042481198,
-11.0536120297623));
#37919=CARTESIAN_POINT('Ctrl Pts',(-4.84978803993833,-33.4292484236839,
-11.1668261479111));
#37920=CARTESIAN_POINT('Ctrl Pts',(-4.58089877613062,-33.4407435519771,
-11.2836056086468));
#37921=CARTESIAN_POINT('Ctrl Pts',(-4.30778318746436,-33.4522386802703,
-11.3906713514839));
#37922=CARTESIAN_POINT('Ctrl Pts',(-4.03116543587642,-33.4637338085635,
-11.4877393545726));
#37923=CARTESIAN_POINT('Ctrl Pts',(-3.76297864793515,-33.4748785797007,
-11.5818488461391));
#37924=CARTESIAN_POINT('Ctrl Pts',(-3.49150028225666,-33.4860233508378,
-11.6665609182723));
#37925=CARTESIAN_POINT('Ctrl Pts',(-3.2174076966831,-33.497168121975,-11.7416667455402));
#37926=CARTESIAN_POINT('Ctrl Pts',(-2.9303901756055,-33.5088384288462,-11.8203142153935));
#37927=CARTESIAN_POINT('Ctrl Pts',(-2.64050625979877,-33.5205087357174,
-11.8884275851291));
#37928=CARTESIAN_POINT('Ctrl Pts',(-2.34854926057755,-33.5321790425887,
-11.9458263264054));
#37929=CARTESIAN_POINT('Ctrl Pts',(-2.05659226135631,-33.5438493494599,
-12.0032250676818));
#37930=CARTESIAN_POINT('Ctrl Pts',(-1.7625625096131,-33.5555196563311,-12.0499091243916));
#37931=CARTESIAN_POINT('Ctrl Pts',(-1.46726435779509,-33.5671899632023,
-12.0857596184247));
#37932=CARTESIAN_POINT('Ctrl Pts',(-1.18519988690572,-33.5783372694502,
-12.1200034854055));
#37933=CARTESIAN_POINT('Ctrl Pts',(-0.901893961091638,-33.589484575698,
-12.1443736781867));
#37934=CARTESIAN_POINT('Ctrl Pts',(-0.618051873483406,-33.6006318819459,
-12.1588018378327));
#37935=CARTESIAN_POINT('Ctrl Pts',(-0.33425799641702,-33.6117772948253,
-12.1732275468576));
#37936=CARTESIAN_POINT('Ctrl Pts',(-0.0499284056740375,-33.6229227077046,
-12.177714580606));
#37937=CARTESIAN_POINT('Ctrl Pts',(0.234228423537759,-33.634068120584,-12.1722466001806));
#37938=CARTESIAN_POINT('Ctrl Pts',(0.518353706925605,-33.6452122961493,
-12.1667792267859));
#37939=CARTESIAN_POINT('Ctrl Pts',(0.802306000450644,-33.6563564717146,
-12.1513590511794));
#37940=CARTESIAN_POINT('Ctrl Pts',(1.0853775201037,-33.6675006472799,-12.1260218492651));
#37941=CARTESIAN_POINT('Ctrl Pts',(1.37736353694585,-33.6789957755722,-12.0998867273921));
#37942=CARTESIAN_POINT('Ctrl Pts',(1.66841210986734,-33.6904909038645,-12.0631998598776));
#37943=CARTESIAN_POINT('Ctrl Pts',(1.95775146155432,-33.7019860321568,-12.0160583996909));
#37944=CARTESIAN_POINT('Ctrl Pts',(2.23827211116114,-33.7131308032951,-11.9703537523351));
#37945=CARTESIAN_POINT('Ctrl Pts',(2.51718591111053,-33.7242755744335,-11.9148224061326));
#37946=CARTESIAN_POINT('Ctrl Pts',(2.79379816578905,-33.7354203455718,-11.8496051435832));
#37947=CARTESIAN_POINT('Ctrl Pts',(3.08345417180536,-33.7470906524411,-11.7813125373307));
#37948=CARTESIAN_POINT('Ctrl Pts',(3.37058603990602,-33.7587609593103,-11.7023986217551));
#37949=CARTESIAN_POINT('Ctrl Pts',(3.65441080124198,-33.7704312661796,-11.6130845147087));
#37950=CARTESIAN_POINT('Ctrl Pts',(3.93823556257797,-33.7821015730489,-11.5237704076622));
#37951=CARTESIAN_POINT('Ctrl Pts',(4.2187528997546,-33.7937718799181,-11.4240562182253));
#37952=CARTESIAN_POINT('Ctrl Pts',(4.495199651367,-33.8054421867874,-11.3142224807695));
#37953=CARTESIAN_POINT('Ctrl Pts',(4.75926020200681,-33.8165896053773,-11.2093098456155));
#37954=CARTESIAN_POINT('Ctrl Pts',(5.01968578183422,-33.8277370239671,-11.0951332138277));
#37955=CARTESIAN_POINT('Ctrl Pts',(5.27582436586328,-33.838884442557,-10.971970083379));
#37956=CARTESIAN_POINT('Ctrl Pts',(5.53191609534507,-33.8500298219881,-10.8488294827367));
#37957=CARTESIAN_POINT('Ctrl Pts',(5.78372215460884,-33.8611752014191,-10.7167057814429));
#37958=CARTESIAN_POINT('Ctrl Pts',(6.03061264389333,-33.8723205808502,-10.5759236660121));
#37959=CARTESIAN_POINT('Ctrl Pts',(6.27749257898572,-33.8834654838333,-10.4351475688021));
#37960=CARTESIAN_POINT('Ctrl Pts',(6.51945713068993,-33.8946103868163,-10.2857139263875));
#37961=CARTESIAN_POINT('Ctrl Pts',(6.75590182217983,-33.9057552897994,-10.1279929314286));
#37962=CARTESIAN_POINT('Ctrl Pts',(6.9799620768191,-33.916316448033,-9.9785330045858));
#37963=CARTESIAN_POINT('Ctrl Pts',(7.19906559768597,-33.9268776062666,-9.82163158858564));
#37964=CARTESIAN_POINT('Ctrl Pts',(7.41272179941099,-33.9374387645002,-9.65763976210218));
#37965=CARTESIAN_POINT('',(-12.1744999999831,-32.6251260039388,-2.02629457301205E-5));
#37966=CARTESIAN_POINT('Ctrl Pts',(-12.1744999999831,-32.6251260039651,
-2.02636154117562E-5));
#37967=CARTESIAN_POINT('Ctrl Pts',(-12.1744999682797,-32.6258732859801,
-0.0190678768165046));
#37968=CARTESIAN_POINT('Ctrl Pts',(-12.1744552351083,-32.6266205679952,
-0.0381154725570181));
#37969=CARTESIAN_POINT('Ctrl Pts',(-12.1743658010439,-32.6273678500103,
-0.057162858329975));
#37970=CARTESIAN_POINT('Ctrl Pts',(-12.1730317010868,-32.6385151562574,
-0.341295271704965));
#37971=CARTESIAN_POINT('Ctrl Pts',(-12.1617461874558,-32.6496624625045,
-0.625423396093907));
#37972=CARTESIAN_POINT('Ctrl Pts',(-12.1405297269587,-32.6608097687516,
-0.908838928981096));
#37973=CARTESIAN_POINT('Ctrl Pts',(-12.1193168700748,-32.6719551816302,
-1.19220632377607));
#37974=CARTESIAN_POINT('Ctrl Pts',(-12.0881764538661,-32.6831005945087,
-1.47486110281071));
#37975=CARTESIAN_POINT('Ctrl Pts',(-12.0471809543266,-32.6942460073873,
-1.75609831834951));
#37976=CARTESIAN_POINT('Ctrl Pts',(-12.0061900059243,-32.7053901829519,
-2.03730431218924));
#37977=CARTESIAN_POINT('Ctrl Pts',(-11.9553461973366,-32.7165343585165,
-2.31709279288919));
#37978=CARTESIAN_POINT('Ctrl Pts',(-11.8947736229075,-32.7276785340811,
-2.59476602216561));
#37979=CARTESIAN_POINT('Ctrl Pts',(-11.8322934950546,-32.739173662374,-2.88118374553293));
#37980=CARTESIAN_POINT('Ctrl Pts',(-11.7594619685466,-32.7506687906668,
-3.16535053951657));
#37981=CARTESIAN_POINT('Ctrl Pts',(-11.6764720426416,-32.7621639189597,
-3.44651285902283));
#37982=CARTESIAN_POINT('Ctrl Pts',(-11.5960115460404,-32.7733086900973,
-3.71910570214559));
#37983=CARTESIAN_POINT('Ctrl Pts',(-11.506002790155,-32.7844534612349,-3.98887423638641));
#37984=CARTESIAN_POINT('Ctrl Pts',(-11.4066724115637,-32.7955982323725,
-4.25514685354945));
#37985=CARTESIAN_POINT('Ctrl Pts',(-11.3026580728741,-32.807268539243,-4.53397565273587));
#37986=CARTESIAN_POINT('Ctrl Pts',(-11.1884219401367,-32.8189388461134,
-4.80897060131908));
#37987=CARTESIAN_POINT('Ctrl Pts',(-11.0642814033507,-32.8306091529839,
-5.07938256852815));
#37988=CARTESIAN_POINT('Ctrl Pts',(-10.9401408665647,-32.8422794598544,
-5.34979453573721));
#37989=CARTESIAN_POINT('Ctrl Pts',(-10.8060960736838,-32.8539497667249,
-5.61562322032863));
#37990=CARTESIAN_POINT('Ctrl Pts',(-10.6625208843845,-32.8656200735954,
-5.87614658088653));
#37991=CARTESIAN_POINT('Ctrl Pts',(-10.5253799657805,-32.8767673798425,
-6.12499468033231));
#37992=CARTESIAN_POINT('Ctrl Pts',(-10.3795031187475,-32.8879146860897,
-6.3690768373752));
#37993=CARTESIAN_POINT('Ctrl Pts',(-10.2252472674586,-32.8990619923368,
-6.60778091111761));
#37994=CARTESIAN_POINT('Ctrl Pts',(-10.0710176165062,-32.9102074052154,
-6.84644444100378));
#37995=CARTESIAN_POINT('Ctrl Pts',(-9.9084119473859,-32.921352818094,-7.07973148737207));
#37996=CARTESIAN_POINT('Ctrl Pts',(-9.73783124627379,-32.9324982309726,
-7.30705774365399));
#37997=CARTESIAN_POINT('Ctrl Pts',(-9.56726948226978,-32.9436424065372,
-7.53435876318956));
#37998=CARTESIAN_POINT('Ctrl Pts',(-9.3887346142411,-32.9547865821018,-7.75570010072467));
#37999=CARTESIAN_POINT('Ctrl Pts',(-9.20266950256293,-32.9659307576664,
-7.97052848163773));
#38000=CARTESIAN_POINT('Ctrl Pts',(-9.01074482252143,-32.9774258859592,
-8.19212224469573));
#38001=CARTESIAN_POINT('Ctrl Pts',(-8.81080811489427,-32.9889210142521,
-8.40678596077151));
#38002=CARTESIAN_POINT('Ctrl Pts',(-8.60338944894226,-33.0004161425449,
-8.6139503272209));
#38003=CARTESIAN_POINT('Ctrl Pts',(-8.40229264490357,-33.0115609136825,
-8.81480058248823));
#38004=CARTESIAN_POINT('Ctrl Pts',(-8.19416340784828,-33.0227056848202,
-9.00860166320182));
#38005=CARTESIAN_POINT('Ctrl Pts',(-7.97952213246204,-33.0338504559578,
-9.19487230947491));
#38006=CARTESIAN_POINT('Ctrl Pts',(-7.75475936973759,-33.0455207628282,
-9.38992661576092));
#38007=CARTESIAN_POINT('Ctrl Pts',(-7.52285587600274,-33.0571910696987,
-9.57672298982141));
#38008=CARTESIAN_POINT('Ctrl Pts',(-7.28444883114305,-33.0688613765691,
-9.75475553135283));
#38009=CARTESIAN_POINT('Ctrl Pts',(-7.04604178628334,-33.0805316834396,
-9.93278807288427));
#38010=CARTESIAN_POINT('Ctrl Pts',(-6.80113146436942,-33.09220199031,-10.1020565881776));
#38011=CARTESIAN_POINT('Ctrl Pts',(-6.55039166588011,-33.1038722971805,
-10.2621059862763));
#38012=CARTESIAN_POINT('Ctrl Pts',(-6.31088868167215,-33.1150196034276,
-10.4149828279117));
#38013=CARTESIAN_POINT('Ctrl Pts',(-6.06599569770914,-33.1261669096747,
-10.5594943509551));
#38014=CARTESIAN_POINT('Ctrl Pts',(-5.81631905191834,-33.1373142159218,
-10.695273859808));
#38015=CARTESIAN_POINT('Ctrl Pts',(-5.56668481367376,-33.1484596288003,
-10.8310303065287));
#38016=CARTESIAN_POINT('Ctrl Pts',(-5.31226877001417,-33.1596050416789,
-10.9580575727416));
#38017=CARTESIAN_POINT('Ctrl Pts',(-5.05370262822269,-33.1707504545575,
-11.0760344887281));
#38018=CARTESIAN_POINT('Ctrl Pts',(-4.79516519128955,-33.1818946301221,
-11.1939983074444));
#38019=CARTESIAN_POINT('Ctrl Pts',(-4.53247881883711,-33.1930388056867,
-11.3029136715195));
#38020=CARTESIAN_POINT('Ctrl Pts',(-4.26629713627511,-33.2041829812513,
-11.4025066978718));
#38021=CARTESIAN_POINT('Ctrl Pts',(-3.9917328517731,-33.2156781095442,-11.5052361109501));
#38022=CARTESIAN_POINT('Ctrl Pts',(-3.71344981544439,-33.227173237837,-11.5980463999713));
#38023=CARTESIAN_POINT('Ctrl Pts',(-3.43218589779943,-33.2386683661299,
-11.6806913413953));
#38024=CARTESIAN_POINT('Ctrl Pts',(-3.15949455312228,-33.2498131372675,
-11.7608173682115));
#38025=CARTESIAN_POINT('Ctrl Pts',(-2.8840016112494,-33.2609579084051,-11.8313884471381));
#38026=CARTESIAN_POINT('Ctrl Pts',(-2.60639431557328,-33.2721026795427,
-11.8922310321381));
#38027=CARTESIAN_POINT('Ctrl Pts',(-2.31569634698968,-33.2837729864132,
-11.9559426713433));
#38028=CARTESIAN_POINT('Ctrl Pts',(-2.02268013077371,-33.2954432932836,
-12.0089861705082));
#38029=CARTESIAN_POINT('Ctrl Pts',(-1.7281472467221,-33.3071136001541,-12.0512222344311));
#38030=CARTESIAN_POINT('Ctrl Pts',(-1.43361436267048,-33.3187839070246,
-12.0934582983541));
#38031=CARTESIAN_POINT('Ctrl Pts',(-1.13756514413288,-33.3304542138951,
-12.1248868881006));
#38032=CARTESIAN_POINT('Ctrl Pts',(-0.840809011698687,-33.3421245207656,
-12.1454308468595));
#38033=CARTESIAN_POINT('Ctrl Pts',(-0.557351899073608,-33.3532718270128,
-12.1650541354633));
#38034=CARTESIAN_POINT('Ctrl Pts',(-0.273165182359102,-33.3644191332599,
-12.1747527915611));
#38035=CARTESIAN_POINT('Ctrl Pts',(0.0110432552658722,-33.375566439507,
-12.1744949914365));
#38036=CARTESIAN_POINT('Ctrl Pts',(0.295203420124147,-33.3867118523856,
-12.1742372350993));
#38037=CARTESIAN_POINT('Ctrl Pts',(0.579385031881237,-33.3978572652642,
-12.1640263990678));
#38038=CARTESIAN_POINT('Ctrl Pts',(0.862879717510703,-33.4090026781428,
-12.1438827745951));
#38039=CARTESIAN_POINT('Ctrl Pts',(1.14634293082577,-33.4201468537074,-12.1237413863777));
#38040=CARTESIAN_POINT('Ctrl Pts',(1.42911910428309,-33.431291029272,-12.0936694305245));
#38041=CARTESIAN_POINT('Ctrl Pts',(1.71050324800699,-33.4424352048366,-12.0537392077545));
#38042=CARTESIAN_POINT('Ctrl Pts',(2.00074875005628,-33.4539303331295,-12.0125515011501));
#38043=CARTESIAN_POINT('Ctrl Pts',(2.28951283081739,-33.4654254614223,-11.9608745844622));
#38044=CARTESIAN_POINT('Ctrl Pts',(2.57602976407274,-33.4769205897152,-11.8988453601436));
#38045=CARTESIAN_POINT('Ctrl Pts',(2.85381401900554,-33.4880653608528,-11.83870670912));
#38046=CARTESIAN_POINT('Ctrl Pts',(3.12948580577611,-33.4992101319904,-11.7688375157536));
#38047=CARTESIAN_POINT('Ctrl Pts',(3.40235863131958,-33.510354903128,-11.6894142707787));
#38048=CARTESIAN_POINT('Ctrl Pts',(3.68809887410928,-33.5220252099985,-11.6062457938259));
#38049=CARTESIAN_POINT('Ctrl Pts',(3.97076952676932,-33.5336955168689,-11.5126006236716));
#38050=CARTESIAN_POINT('Ctrl Pts',(4.24960009200961,-33.5453658237394,-11.4087400403371));
#38051=CARTESIAN_POINT('Ctrl Pts',(4.52843065724992,-33.5570361306098,-11.3048794570027));
#38052=CARTESIAN_POINT('Ctrl Pts',(4.80342082373624,-33.5687064374803,-11.1908035858233));
#38053=CARTESIAN_POINT('Ctrl Pts',(5.07382294533181,-33.5803767443507,-11.0668320204756));
#38054=CARTESIAN_POINT('Ctrl Pts',(5.33210550270062,-33.5915239819759,-10.948416925394));
#38055=CARTESIAN_POINT('Ctrl Pts',(5.58627938950382,-33.6026712196011,-10.8209383299319));
#38056=CARTESIAN_POINT('Ctrl Pts',(5.83570782148966,-33.6138184572262,-10.6847070372661));
#38057=CARTESIAN_POINT('Ctrl Pts',(6.08509174313785,-33.6249637056343,-10.5485000549839));
#38058=CARTESIAN_POINT('Ctrl Pts',(6.32973166681211,-33.6361089540423,-10.4035436219664));
#38059=CARTESIAN_POINT('Ctrl Pts',(6.56901533244333,-33.6472542024504,-10.2501945255748));
#38060=CARTESIAN_POINT('Ctrl Pts',(6.80827488209085,-33.6583983275948,-10.0968608843306));
#38061=CARTESIAN_POINT('Ctrl Pts',(7.04217902691351,-33.6695424527393,-9.9351364122925));
#38062=CARTESIAN_POINT('Ctrl Pts',(7.27014334671615,-33.6806865778837,-9.76542195546096));
#38063=CARTESIAN_POINT('Ctrl Pts',(7.31793216376122,-33.6830227529401,-9.72984422498785));
#38064=CARTESIAN_POINT('Ctrl Pts',(7.36546005321909,-33.6853589279964,-9.69391551734931));
#38065=CARTESIAN_POINT('Ctrl Pts',(7.412721799411,-33.6876951030527,-9.65763976210218));
#38066=CARTESIAN_POINT('Ctrl Pts',(7.41272179941101,-30.6876856710377,-9.65763976210217));
#38067=CARTESIAN_POINT('Ctrl Pts',(7.63967546407975,-30.6989071344683,-9.48344146738549));
#38068=CARTESIAN_POINT('Ctrl Pts',(7.86046128966899,-30.7101285978989,-9.30125847901165));
#38069=CARTESIAN_POINT('Ctrl Pts',(8.07452674462437,-30.7213500613295,-9.11155684284227));
#38070=CARTESIAN_POINT('Ctrl Pts',(8.28717754530411,-30.7324973675766,-8.92310885234291));
#38071=CARTESIAN_POINT('Ctrl Pts',(8.49326006179604,-30.7436446738237,-8.72718501437767));
#38072=CARTESIAN_POINT('Ctrl Pts',(8.69225549345207,-30.7547919800708,-8.5242679853787));
#38073=CARTESIAN_POINT('Ctrl Pts',(8.89121712575985,-30.7659373929494,-8.32138542181079));
#38074=CARTESIAN_POINT('Ctrl Pts',(9.08309388980057,-30.777082805828,-8.11151222901466));
#38075=CARTESIAN_POINT('Ctrl Pts',(9.26740381715966,-30.7882282187066,-7.89516793612995));
#38076=CARTESIAN_POINT('Ctrl Pts',(9.45169328325431,-30.7993723942712,-7.67884766082179));
#38077=CARTESIAN_POINT('Ctrl Pts',(9.62841741714516,-30.8105165698359,-7.45605792294065));
#38078=CARTESIAN_POINT('Ctrl Pts',(9.79713372167153,-30.8216607454005,-7.22735228764217));
#38079=CARTESIAN_POINT('Ctrl Pts',(9.97116324537854,-30.8331558736934,-6.99144424726733));
#38080=CARTESIAN_POINT('Ctrl Pts',(10.1366722171911,-30.8446510019862,-6.74924189734947));
#38081=CARTESIAN_POINT('Ctrl Pts',(10.2932216574243,-30.8561461302791,-6.50138740278804));
#38082=CARTESIAN_POINT('Ctrl Pts',(10.4449996662181,-30.8672909014166,-6.26108720370023));
#38083=CARTESIAN_POINT('Ctrl Pts',(10.5883560576907,-30.8784356725542,-6.01547453459209));
#38084=CARTESIAN_POINT('Ctrl Pts',(10.7229356202202,-30.8895804436918,-5.76516278474537));
#38085=CARTESIAN_POINT('Ctrl Pts',(10.8638613309254,-30.9012507505623,-5.50304749337414));
#38086=CARTESIAN_POINT('Ctrl Pts',(10.9951623959193,-30.9129210574327,-5.23577956394708));
#38087=CARTESIAN_POINT('Ctrl Pts',(11.1164852149529,-30.9245913643032,-4.96409173119642));
#38088=CARTESIAN_POINT('Ctrl Pts',(11.2378080339866,-30.9362616711737,-4.69240389844574));
#38089=CARTESIAN_POINT('Ctrl Pts',(11.3491524782766,-30.9479319780441,-4.41629647229513));
#38090=CARTESIAN_POINT('Ctrl Pts',(11.4502225594297,-30.9596022849146,-4.13652675435896));
#38091=CARTESIAN_POINT('Ctrl Pts',(11.5467632210884,-30.9707495911617,-3.86929481614853));
#38092=CARTESIAN_POINT('Ctrl Pts',(11.6339589947617,-30.9818968974088,-3.59864180777725));
#38093=CARTESIAN_POINT('Ctrl Pts',(11.7115853118451,-30.993044203656,-3.32523980088261));
#38094=CARTESIAN_POINT('Ctrl Pts',(11.7891984441082,-31.0041896165345,-3.05188423128495));
#38095=CARTESIAN_POINT('Ctrl Pts',(11.8572452920049,-31.015335029413,-2.77578085187103));
#38096=CARTESIAN_POINT('Ctrl Pts',(11.9155512731645,-31.0264804422916,-2.49761648508908));
#38097=CARTESIAN_POINT('Ctrl Pts',(11.9738507814546,-31.0376246178562,-2.21948299887197));
#38098=CARTESIAN_POINT('Ctrl Pts',(12.022411527657,-31.0487687934208,-1.9392892431739));
#38099=CARTESIAN_POINT('Ctrl Pts',(12.0611098753863,-31.0599129689854,-1.65773303757252));
#38100=CARTESIAN_POINT('Ctrl Pts',(12.1010269127024,-31.0714080972782,-1.36731005506706));
#38101=CARTESIAN_POINT('Ctrl Pts',(12.1304502618443,-31.0829032255711,-1.07543771211255));
#38102=CARTESIAN_POINT('Ctrl Pts',(12.1493017737572,-31.094398353864,-0.782889941294685));
#38103=CARTESIAN_POINT('Ctrl Pts',(12.1675787151288,-31.1055431250016,-0.499258661197821));
#38104=CARTESIAN_POINT('Ctrl Pts',(12.17591869138,-31.1166878961392,-0.214992794448297));
#38105=CARTESIAN_POINT('Ctrl Pts',(12.1743033368384,-31.1278326672768,0.069199079805505));
#38106=CARTESIAN_POINT('Ctrl Pts',(12.1726118096663,-31.1395029741473,0.366792125161997));
#38107=CARTESIAN_POINT('Ctrl Pts',(12.1600034675358,-31.1511732810177,0.664303713974559));
#38108=CARTESIAN_POINT('Ctrl Pts',(12.136518471558,-31.1628435878882,0.960921245228644));
#38109=CARTESIAN_POINT('Ctrl Pts',(12.1130334755802,-31.1745138947587,1.25753877648276));
#38110=CARTESIAN_POINT('Ctrl Pts',(12.0786718609865,-31.1861842016292,1.55326191641704));
#38111=CARTESIAN_POINT('Ctrl Pts',(12.0335361321028,-31.1978545084997,1.84728406244831));
#38112=CARTESIAN_POINT('Ctrl Pts',(11.9904231447464,-31.2090018147468,2.12812971129163));
#38113=CARTESIAN_POINT('Ctrl Pts',(11.9374676168789,-31.2201491209939,2.40750735169076));
#38114=CARTESIAN_POINT('Ctrl Pts',(11.8747939778081,-31.231296427241,2.68471939587967));
#38115=CARTESIAN_POINT('Ctrl Pts',(11.8121309838468,-31.2424418401196,2.96188435563876));
#38116=CARTESIAN_POINT('Ctrl Pts',(11.7397532329452,-31.2535872529982,3.2368841934707));
#38117=CARTESIAN_POINT('Ctrl Pts',(11.6578361044304,-31.2647326658768,3.50903228999679));
#38118=CARTESIAN_POINT('Ctrl Pts',(11.5759280699893,-31.2758768414414,3.7811501738566));
#38119=CARTESIAN_POINT('Ctrl Pts',(11.4844828494922,-31.287021017006,4.0504166932242));
#38120=CARTESIAN_POINT('Ctrl Pts',(11.383725818712,-31.2981651925706,4.31615995236384));
#38121=CARTESIAN_POINT('Ctrl Pts',(11.2797957443419,-31.3096603208635,4.59027200659853));
#38122=CARTESIAN_POINT('Ctrl Pts',(11.1659579563437,-31.3211554491563,4.8606350145712));
#38123=CARTESIAN_POINT('Ctrl Pts',(11.0425141946155,-31.3326505774492,5.12653201606268));
#38124=CARTESIAN_POINT('Ctrl Pts',(10.922832844588,-31.3437953485868,5.38432480900107));
#38125=CARTESIAN_POINT('Ctrl Pts',(10.7941225236154,-31.3549401197244,5.63791954766483));
#38126=CARTESIAN_POINT('Ctrl Pts',(10.6567061908373,-31.366084890862,5.88668526525489));
#38127=CARTESIAN_POINT('Ctrl Pts',(10.5128099409518,-31.3777551977325,6.14718162065625));
#38128=CARTESIAN_POINT('Ctrl Pts',(10.3593670062242,-31.3894255046029,6.40238228983842));
#38129=CARTESIAN_POINT('Ctrl Pts',(10.1968015149776,-31.4010958114734,6.65159297568257));
#38130=CARTESIAN_POINT('Ctrl Pts',(10.0342360237311,-31.4127661183439,6.90080366152668));
#38131=CARTESIAN_POINT('Ctrl Pts',(9.86254816662018,-31.4244364252143,7.14402408782862));
#38132=CARTESIAN_POINT('Ctrl Pts',(9.68221394281234,-31.4361067320848,7.38059505836828));
#38133=CARTESIAN_POINT('Ctrl Pts',(9.50996133266801,-31.4472540383319,7.60656418557765));
#38134=CARTESIAN_POINT('Ctrl Pts',(9.32976884399584,-31.4584013445791,7.82653423106822));
#38135=CARTESIAN_POINT('Ctrl Pts',(9.1420795592616,-31.4695486508262,8.0399522126771));
#38136=CARTESIAN_POINT('Ctrl Pts',(8.95442215352886,-31.4806940637047,8.25333394526852));
#38137=CARTESIAN_POINT('Ctrl Pts',(8.75927067002798,-31.4918394765833,8.4601656355874));
#38138=CARTESIAN_POINT('Ctrl Pts',(8.557107679775,-31.5029848894619,8.65992831417996));
#38139=CARTESIAN_POINT('Ctrl Pts',(8.35496713275467,-31.5141290650264,8.85966881601174));
#38140=CARTESIAN_POINT('Ctrl Pts',(8.14581682298889,-31.525273240591,9.05234168573748));
#38141=CARTESIAN_POINT('Ctrl Pts',(7.93017617569519,-31.5364174161556,9.23746480764265));
#38142=CARTESIAN_POINT('Ctrl Pts',(7.70774456633725,-31.5479125444485,9.42841783274024));
#38143=CARTESIAN_POINT('Ctrl Pts',(7.47840742626827,-31.5594076727413,9.61133769016819));
#38144=CARTESIAN_POINT('Ctrl Pts',(7.24277279859588,-31.5709028010342,9.78573923819349));
#38145=CARTESIAN_POINT('Ctrl Pts',(7.01432002011501,-31.5820475721717,9.95482524482719));
#38146=CARTESIAN_POINT('Ctrl Pts',(6.77994817299307,-31.5931923433093,10.1159043417922));
#38147=CARTESIAN_POINT('Ctrl Pts',(6.54024278067235,-31.6043371144469,10.2685770494194));
#38148=CARTESIAN_POINT('Ctrl Pts',(6.28923399346961,-31.6160074213174,10.4284490940549));
#38149=CARTESIAN_POINT('Ctrl Pts',(6.03237681530273,-31.6276777281879,10.57910268941));
#38150=CARTESIAN_POINT('Ctrl Pts',(5.77037590892259,-31.6393480350584,10.7201311614982));
#38151=CARTESIAN_POINT('Ctrl Pts',(5.50837500254246,-31.6510183419289,10.8611596335865));
#38152=CARTESIAN_POINT('Ctrl Pts',(5.24123066753154,-31.6626886487994,10.9925628311193));
#38153=CARTESIAN_POINT('Ctrl Pts',(4.96967631529748,-31.6743589556699,11.1139897233699));
#38154=CARTESIAN_POINT('Ctrl Pts',(4.71029157411813,-31.685506261917,11.2299749129259));
#38155=CARTESIAN_POINT('Ctrl Pts',(4.44680592598916,-31.6966535681641,11.3368929521746));
#38156=CARTESIAN_POINT('Ctrl Pts',(4.1798730513762,-31.7078008744112,11.4344703211115));
#38157=CARTESIAN_POINT('Ctrl Pts',(3.9129855152784,-31.7189462872898,11.5320311165445));
#38158=CARTESIAN_POINT('Ctrl Pts',(3.64265217210709,-31.7300917001683,11.6202543175883));
#38159=CARTESIAN_POINT('Ctrl Pts',(3.36954509927963,-31.7412371130469,11.6989151665409));
#38160=CARTESIAN_POINT('Ctrl Pts',(3.09646834558192,-31.7523812886114,11.7775672829167));
#38161=CARTESIAN_POINT('Ctrl Pts',(2.82061873337085,-31.7635254641758,11.8466590931784));
#38162=CARTESIAN_POINT('Ctrl Pts',(2.54268306433363,-31.7746696397403,11.9060158358853));
#38163=CARTESIAN_POINT('Ctrl Pts',(2.2559946364402,-31.7861647680332,11.9672418430058));
#38164=CARTESIAN_POINT('Ctrl Pts',(1.96708692245802,-31.7976598963261,12.0181096212011));
#38165=CARTESIAN_POINT('Ctrl Pts',(1.67672598435743,-31.809155024619,12.0584841594365));
#38166=CARTESIAN_POINT('Ctrl Pts',(1.39521488504789,-31.8202997957566,12.0976281321661));
#38167=CARTESIAN_POINT('Ctrl Pts',(1.11233811118305,-31.8314445668942,12.1269089964084));
#38168=CARTESIAN_POINT('Ctrl Pts',(0.828800958063812,-31.8425893380319,
12.1462561813059));
#38169=CARTESIAN_POINT('Ctrl Pts',(0.531893507454375,-31.8542596449024,
12.1665156897378));
#38170=CARTESIAN_POINT('Ctrl Pts',(0.234262215273674,-31.8659299517729,
12.1758821023111));
#38171=CARTESIAN_POINT('Ctrl Pts',(-0.0632795684179096,-31.8776002586434,
12.1743355443417));
#38172=CARTESIAN_POINT('Ctrl Pts',(-0.360821352109494,-31.889270565514,
12.1727889863723));
#38173=CARTESIAN_POINT('Ctrl Pts',(-0.658273291861257,-31.9009408723845,
12.1603294683821));
#38174=CARTESIAN_POINT('Ctrl Pts',(-0.95482342212009,-31.912611179255,12.1369997315058));
#38175=CARTESIAN_POINT('Ctrl Pts',(-1.23808376448244,-31.9237584855021,
12.1147155084335));
#38176=CARTESIAN_POINT('Ctrl Pts',(-1.52060594814087,-31.9349057917492,
12.0825072854502));
#38177=CARTESIAN_POINT('Ctrl Pts',(-1.80168510862513,-31.9460530979963,
12.0404477084267));
#38178=CARTESIAN_POINT('Ctrl Pts',(-2.08271652784845,-31.9571985108749,
11.9983952752173));
#38179=CARTESIAN_POINT('Ctrl Pts',(-2.36230514952426,-31.9683439237534,
11.9464948680739));
#38180=CARTESIAN_POINT('Ctrl Pts',(-2.63975329032011,-31.9794893366319,
11.8848707530307));
#38181=CARTESIAN_POINT('Ctrl Pts',(-2.9171706300654,-31.9906335121966,11.8232534792208));
#38182=CARTESIAN_POINT('Ctrl Pts',(-3.19244770309873,-32.0017776877613,
11.751914710889));
#38183=CARTESIAN_POINT('Ctrl Pts',(-3.46489782257824,-32.0129218633259,
11.6710296601925));
#38184=CARTESIAN_POINT('Ctrl Pts',(-3.74592794980863,-32.0244169916188,
11.5875973749297));
#38185=CARTESIAN_POINT('Ctrl Pts',(-4.02394989801542,-32.0359121199116,
11.4940078756704));
#38186=CARTESIAN_POINT('Ctrl Pts',(-4.29822640699997,-32.0474072482045,
11.3905092074133));
#38187=CARTESIAN_POINT('Ctrl Pts',(-4.56414331050772,-32.0585520193421,
11.2901650493154));
#38188=CARTESIAN_POINT('Ctrl Pts',(-4.82653944546716,-32.0696967904797,
11.1805069143627));
#38189=CARTESIAN_POINT('Ctrl Pts',(-5.08476174609812,-32.0808415616173,
11.0618103507255));
#38190=CARTESIAN_POINT('Ctrl Pts',(-5.35516061314951,-32.0925118684878,
10.9375166074974));
#38191=CARTESIAN_POINT('Ctrl Pts',(-5.62098224809431,-32.1041821753582,
10.8033116367849));
#38192=CARTESIAN_POINT('Ctrl Pts',(-5.88150296641168,-32.1158524822287,
10.6595672100743));
#38193=CARTESIAN_POINT('Ctrl Pts',(-6.14202368472907,-32.1275227890992,
10.5158227833637));
#38194=CARTESIAN_POINT('Ctrl Pts',(-6.39724319690685,-32.1391930959696,
10.3625390704213));
#38195=CARTESIAN_POINT('Ctrl Pts',(-6.64646899845364,-32.1508634028401,
10.2001421609012));
#38196=CARTESIAN_POINT('Ctrl Pts',(-6.88452583494995,-32.1620107090872,
10.0450230107282));
#38197=CARTESIAN_POINT('Ctrl Pts',(-7.11718546291348,-32.1731580153343,
9.88154319117064));
#38198=CARTESIAN_POINT('Ctrl Pts',(-7.3438637301814,-32.1843053215814,9.71010379772154));
#38199=CARTESIAN_POINT('Ctrl Pts',(-7.57050349617527,-32.19545073446,9.53869352323099));
#38200=CARTESIAN_POINT('Ctrl Pts',(-7.79116371711331,-32.2065961473386,
9.3593265348274));
#38201=CARTESIAN_POINT('Ctrl Pts',(-8.00529124878566,-32.2177415602172,
9.17244581734423));
#38202=CARTESIAN_POINT('Ctrl Pts',(-8.2193950089754,-32.2288857357819,8.98558584652402));
#38203=CARTESIAN_POINT('Ctrl Pts',(-8.42696732714878,-32.2400299113465,
8.79121398762406));
#38204=CARTESIAN_POINT('Ctrl Pts',(-8.627489094617,-32.2511740869111,8.58981269715847));
#38205=CARTESIAN_POINT('Ctrl Pts',(-8.83432569990824,-32.2626692152039,
8.3820688709039));
#38206=CARTESIAN_POINT('Ctrl Pts',(-9.03366027000809,-32.2741643434968,
8.16684589996586));
#38207=CARTESIAN_POINT('Ctrl Pts',(-9.22496414319454,-32.2856594717896,
7.94471439428599));
#38208=CARTESIAN_POINT('Ctrl Pts',(-9.41043731322679,-32.2968042429273,
7.72935317950114));
#38209=CARTESIAN_POINT('Ctrl Pts',(-9.58836188649626,-32.3079490140649,
7.50749853242398));
#38210=CARTESIAN_POINT('Ctrl Pts',(-9.75829629083444,-32.3190937852025,
7.27970492192416));
#38211=CARTESIAN_POINT('Ctrl Pts',(-9.93624401376104,-32.3307640920729,
7.04116962094411));
#38212=CARTESIAN_POINT('Ctrl Pts',(-10.1054296870796,-32.3424343989434,
6.79612202615387));
#38213=CARTESIAN_POINT('Ctrl Pts',(-10.2653957777935,-32.3541047058139,
6.54523489076284));
#38214=CARTESIAN_POINT('Ctrl Pts',(-10.4253618685074,-32.3657750126843,
6.2943477553718));
#38215=CARTESIAN_POINT('Ctrl Pts',(-10.576108203647,-32.3774453195548,6.03762136698964));
#38216=CARTESIAN_POINT('Ctrl Pts',(-10.7172306218485,-32.3891156264253,
5.77576125269328));
#38217=CARTESIAN_POINT('Ctrl Pts',(-10.8519688998768,-32.4002579882968,
5.52574724829742));
#38218=CARTESIAN_POINT('Ctrl Pts',(-10.9779752599429,-32.4114003501683,
5.27097837052066));
#38219=CARTESIAN_POINT('Ctrl Pts',(-11.0949288753281,-32.4225427120399,
5.0120857436213));
#38220=CARTESIAN_POINT('Ctrl Pts',(-11.2118624589273,-32.4336831654505,
4.75323745978609));
#38221=CARTESIAN_POINT('Ctrl Pts',(-11.3197462835136,-32.4448236188611,
4.49026708040664));
#38222=CARTESIAN_POINT('Ctrl Pts',(-11.418306790496,-32.4559640722717,4.22382768210448));
#38223=CARTESIAN_POINT('Ctrl Pts',(-11.5168563332357,-32.4671032863762,
3.9574179235265));
#38224=CARTESIAN_POINT('Ctrl Pts',(-11.6060845367131,-32.4782425004807,
3.68754016717926));
#38225=CARTESIAN_POINT('Ctrl Pts',(-11.6857666143717,-32.4893817145852,
3.41486586624351));
#38226=CARTESIAN_POINT('Ctrl Pts',(-11.7666848528916,-32.500693738698,3.13796138822696));
#38227=CARTESIAN_POINT('Ctrl Pts',(-11.8377582625043,-32.5120057628108,
2.85817315383455));
#38228=CARTESIAN_POINT('Ctrl Pts',(-11.8988041826084,-32.5233177869236,
2.57621995837733));
#38229=CARTESIAN_POINT('Ctrl Pts',(-11.9589208024357,-32.5344576084204,
2.29855892826241));
#38230=CARTESIAN_POINT('Ctrl Pts',(-12.009312981119,-32.5455974299172,2.01879864552249));
#38231=CARTESIAN_POINT('Ctrl Pts',(-12.0498576548315,-32.556737251414,1.73763654090826));
#38232=CARTESIAN_POINT('Ctrl Pts',(-12.0913424556654,-32.5681353768348,
1.44995500733155));
#38233=CARTESIAN_POINT('Ctrl Pts',(-12.1225175320442,-32.5795335022556,
1.16080614795246));
#38234=CARTESIAN_POINT('Ctrl Pts',(-12.1433070423736,-32.5909316276764,
0.870944501468714));
#38235=CARTESIAN_POINT('Ctrl Pts',(-12.1640965527031,-32.6023297530972,
0.581082854984967));
#38236=CARTESIAN_POINT('Ctrl Pts',(-12.1745004835326,-32.613727878518,0.290508720558424));
#38237=CARTESIAN_POINT('Ctrl Pts',(-12.1744999999831,-32.6251260039388,
-2.02629457920173E-5));
#38238=CARTESIAN_POINT('Origin',(0.,-13.3748739960349,0.));
#38239=CARTESIAN_POINT('',(7.412721799411,-27.6877007372717,-9.65763976210218));
#38240=CARTESIAN_POINT('',(7.41272179941101,-27.9374461219842,-9.65763976210217));
#38241=CARTESIAN_POINT('',(7.41272179941101,-13.3748739960349,-9.65763976210217));
#38242=CARTESIAN_POINT('',(-12.174396721221,-29.8748739960031,-4.71261348963091E-6));
#38243=CARTESIAN_POINT('Ctrl Pts',(7.41272179941101,-27.9374461219842,-9.65763976210217));
#38244=CARTESIAN_POINT('Ctrl Pts',(7.63815696377125,-27.9485898492208,-9.48460699236017));
#38245=CARTESIAN_POINT('Ctrl Pts',(7.8575395359938,-27.9597335764574,-9.303670767682));
#38246=CARTESIAN_POINT('Ctrl Pts',(8.0703221215742,-27.970877303694,-9.11528118622954));
#38247=CARTESIAN_POINT('Ctrl Pts',(8.28312509826385,-27.982022098842,-8.92687355126708));
#38248=CARTESIAN_POINT('Ctrl Pts',(8.48932662312901,-27.9931668939901,-8.73101130733214));
#38249=CARTESIAN_POINT('Ctrl Pts',(8.68841372480532,-28.0043116891381,-8.52818369857348));
#38250=CARTESIAN_POINT('Ctrl Pts',(8.88750330607416,-28.0154566230925,-8.32535356363499));
#38251=CARTESIAN_POINT('Ctrl Pts',(9.0794781021168,-28.0266015570469,-8.11555808277237));
#38252=CARTESIAN_POINT('Ctrl Pts',(9.26386259015722,-28.0377464910013,-7.89932276595188));
#38253=CARTESIAN_POINT('Ctrl Pts',(9.44828472996781,-28.0488937007788,-7.68304329334291));
#38254=CARTESIAN_POINT('Ctrl Pts',(9.62511329145496,-28.0600409105564,-7.46032156006608));
#38255=CARTESIAN_POINT('Ctrl Pts',(9.79391260850612,-28.0711881203339,-7.23171667496349));
#38256=CARTESIAN_POINT('Ctrl Pts',(9.87568694844433,-28.0765883538043,-7.12096970090879));
#38257=CARTESIAN_POINT('Ctrl Pts',(9.95557752999588,-28.0819885872747,-7.00884249464973));
#38258=CARTESIAN_POINT('Ctrl Pts',(10.0335383821488,-28.087388820745,-6.89540120543738));
#38259=CARTESIAN_POINT('Ctrl Pts',(10.194467256614,-28.0985361269921,-6.66123266460331));
#38260=CARTESIAN_POINT('Ctrl Pts',(10.3472188441184,-28.1096834332392,-6.42139291309911));
#38261=CARTESIAN_POINT('Ctrl Pts',(10.4914060523786,-28.1208307394863,-6.1764754750677));
#38262=CARTESIAN_POINT('Ctrl Pts',(10.6355687704599,-28.1319761523649,-5.93159963623197));
#38263=CARTESIAN_POINT('Ctrl Pts',(10.7711698782457,-28.1431215652434,-5.68164806252201));
#38264=CARTESIAN_POINT('Ctrl Pts',(10.8978669207609,-28.154266978122,-5.42724118013789));
#38265=CARTESIAN_POINT('Ctrl Pts',(11.0245498979363,-28.1654111536866,-5.1728625408699));
#38266=CARTESIAN_POINT('Ctrl Pts',(11.1423306648156,-28.1765553292512,-4.91402981929681));
#38267=CARTESIAN_POINT('Ctrl Pts',(11.250913280774,-28.1876995048158,-4.65138695428623));
#38268=CARTESIAN_POINT('Ctrl Pts',(11.3629153838978,-28.1991946331086,-4.38047293188917));
#38269=CARTESIAN_POINT('Ctrl Pts',(11.4651304890387,-28.2106897614015,-4.10550516952863));
#38270=CARTESIAN_POINT('Ctrl Pts',(11.5572874357625,-28.2221848896944,-3.82721274260596));
#38271=CARTESIAN_POINT('Ctrl Pts',(11.6466355538357,-28.2333296608319,-3.55740232132468));
#38272=CARTESIAN_POINT('Ctrl Pts',(11.7265294669145,-28.2444744319695,-3.28446716262288));
#38273=CARTESIAN_POINT('Ctrl Pts',(11.7967723708194,-28.2556192031071,-3.00908821423886));
#38274=CARTESIAN_POINT('Ctrl Pts',(11.8703276043836,-28.2672895099776,-2.72072367147365));
#38275=CARTESIAN_POINT('Ctrl Pts',(11.9332996556248,-28.2789598168481,-2.42967962578353));
#38276=CARTESIAN_POINT('Ctrl Pts',(11.9855220652797,-28.2906301237186,-2.13675245938659));
#38277=CARTESIAN_POINT('Ctrl Pts',(12.0377444749345,-28.3023004305891,-1.84382529298966));
#38278=CARTESIAN_POINT('Ctrl Pts',(12.0792171927608,-28.3139707374596,-1.54901533771966));
#38279=CARTESIAN_POINT('Ctrl Pts',(12.1098355954862,-28.3256410443301,-1.25312892405157));
#38280=CARTESIAN_POINT('Ctrl Pts',(12.1390818454577,-28.3367883505772,-0.970502554057997));
#38281=CARTESIAN_POINT('Ctrl Pts',(12.1584339953508,-28.3479356568243,-0.686809677550053));
#38282=CARTESIAN_POINT('Ctrl Pts',(12.1678361799058,-28.3590829630714,-0.40275668706502));
#38283=CARTESIAN_POINT('Ctrl Pts',(12.177236767501,-28.37022837595,-0.118751942944197));
#38284=CARTESIAN_POINT('Ctrl Pts',(12.1766907550221,-28.3813737888286,0.165612526537045));
#38285=CARTESIAN_POINT('Ctrl Pts',(12.1661943454187,-28.3925192017072,0.449628067964166));
#38286=CARTESIAN_POINT('Ctrl Pts',(12.1556991010799,-28.4036633772718,0.733612079254089));
#38287=CARTESIAN_POINT('Ctrl Pts',(12.1352556752733,-28.4148075528364,1.0172469733435));
#38288=CARTESIAN_POINT('Ctrl Pts',(12.104912365353,-28.425951728401,1.29982571028703));
#38289=CARTESIAN_POINT('Ctrl Pts',(12.07361348296,-28.4374468566938,1.59130342572396));
#38290=CARTESIAN_POINT('Ctrl Pts',(12.0317810995415,-28.4489419849867,1.88165708895882));
#38291=CARTESIAN_POINT('Ctrl Pts',(11.9795260125188,-28.4604371132795,2.1701167630765));
#38292=CARTESIAN_POINT('Ctrl Pts',(11.9288635952924,-28.4715818844171,2.44978454655556));
#38293=CARTESIAN_POINT('Ctrl Pts',(11.8684044580646,-28.4827266555547,2.727671809539));
#38294=CARTESIAN_POINT('Ctrl Pts',(11.7983016566862,-28.4938714266923,3.00308645693653));
#38295=CARTESIAN_POINT('Ctrl Pts',(11.7248931322342,-28.5055417335628,3.29148838211453));
#38296=CARTESIAN_POINT('Ctrl Pts',(11.6409096368336,-28.5172120404333,3.57717857842725));
#38297=CARTESIAN_POINT('Ctrl Pts',(11.5465861114499,-28.5288823473038,3.85937811322915));
#38298=CARTESIAN_POINT('Ctrl Pts',(11.4522625860663,-28.5405526541742,4.14157764803105));
#38299=CARTESIAN_POINT('Ctrl Pts',(11.3475991453805,-28.5522229610447,4.42028620590779));
#38300=CARTESIAN_POINT('Ctrl Pts',(11.2328897869991,-28.5638932679152,4.6947457101671));
#38301=CARTESIAN_POINT('Ctrl Pts',(11.1233210874371,-28.5750405741623,4.95690541002459));
#38302=CARTESIAN_POINT('Ctrl Pts',(11.0045543630941,-28.5861878804094,5.21526682176328));
#38303=CARTESIAN_POINT('Ctrl Pts',(10.8768785996751,-28.5973351866565,5.46918295341547));
#38304=CARTESIAN_POINT('Ctrl Pts',(10.7492245219682,-28.6084805995351,5.72305595744509));
#38305=CARTESIAN_POINT('Ctrl Pts',(10.6126645460732,-28.6196260124137,5.97248495058034));
#38306=CARTESIAN_POINT('Ctrl Pts',(10.467534458856,-28.6307714252922,6.21684587251955));
#38307=CARTESIAN_POINT('Ctrl Pts',(10.3224204833328,-28.6419156008568,6.46117966660059));
#38308=CARTESIAN_POINT('Ctrl Pts',(10.1687384324912,-28.6530597764214,6.70044628368926));
#38309=CARTESIAN_POINT('Ctrl Pts',(10.0068690633192,-28.664203951986,6.93404800961067));
#38310=CARTESIAN_POINT('Ctrl Pts',(9.83990209886954,-28.6756990802789,7.17500632845005));
#38311=CARTESIAN_POINT('Ctrl Pts',(9.66422395039496,-28.6871942085718,7.40993692714886));
#38312=CARTESIAN_POINT('Ctrl Pts',(9.48030035284617,-28.6986893368646,7.63821677290091));
#38313=CARTESIAN_POINT('Ctrl Pts',(9.30198251686694,-28.7098341080022,7.85953893403023));
#38314=CARTESIAN_POINT('Ctrl Pts',(9.11591458607458,-28.7209788791398,8.0746095348416));
#38315=CARTESIAN_POINT('Ctrl Pts',(8.92256215039984,-28.7321236502774,8.28289411511775));
#38316=CARTESIAN_POINT('Ctrl Pts',(8.72009211035867,-28.7437939571479,8.50100043046518));
#38317=CARTESIAN_POINT('Ctrl Pts',(8.50963424411612,-28.7554642640184,8.71166509837527));
#38318=CARTESIAN_POINT('Ctrl Pts',(8.29176759747592,-28.7671345708889,8.91431659519946));
#38319=CARTESIAN_POINT('Ctrl Pts',(8.07390095083574,-28.7788048777594,9.11696809202363));
#38320=CARTESIAN_POINT('Ctrl Pts',(7.84862577543433,-28.7904751846298,9.31160619568754));
#38321=CARTESIAN_POINT('Ctrl Pts',(7.61656299213793,-28.8021454915003,9.49770595653471));
#38322=CARTESIAN_POINT('Ctrl Pts',(7.39490001937541,-28.8132927977474,9.67546572324013));
#38323=CARTESIAN_POINT('Ctrl Pts',(7.16697823266025,-28.8244401039945,9.84548870117944));
#38324=CARTESIAN_POINT('Ctrl Pts',(6.93336099330269,-28.8355874102417,10.0073450818161));
#38325=CARTESIAN_POINT('Ctrl Pts',(6.69978343380329,-28.8467328231202,10.1691739711672));
#38326=CARTESIAN_POINT('Ctrl Pts',(6.46051257220027,-28.8578782359988,10.322838880697));
#38327=CARTESIAN_POINT('Ctrl Pts',(6.21614189045026,-28.8690236488774,10.4679525336997));
#38328=CARTESIAN_POINT('Ctrl Pts',(5.97179833764223,-28.880167824442,10.6130500768326));
#38329=CARTESIAN_POINT('Ctrl Pts',(5.72235632451466,-28.8913120000066,10.7495981229215));
#38330=CARTESIAN_POINT('Ctrl Pts',(5.46843621193528,-28.9024561755712,10.8772540489774));
#38331=CARTESIAN_POINT('Ctrl Pts',(5.20651963916458,-28.913951303864,11.0089301194816));
#38332=CARTESIAN_POINT('Ctrl Pts',(4.93983860834533,-28.9254464321569,11.1311447906859));
#38333=CARTESIAN_POINT('Ctrl Pts',(4.66910021250522,-28.9369415604497,11.2435738737994));
#38334=CARTESIAN_POINT('Ctrl Pts',(4.40661358487193,-28.9480863315874,11.3525762588611));
#38335=CARTESIAN_POINT('Ctrl Pts',(4.14031351438129,-28.959231102725,11.4523806207877));
#38336=CARTESIAN_POINT('Ctrl Pts',(3.87086458095801,-28.9703758738626,11.5427404738166));
#38337=CARTESIAN_POINT('Ctrl Pts',(3.58870968516497,-28.9820461807331,11.6373612785507));
#38338=CARTESIAN_POINT('Ctrl Pts',(3.30310211058093,-28.9937164876035,11.7216253225378));
#38339=CARTESIAN_POINT('Ctrl Pts',(3.01482379511475,-29.005386794474,11.7953078694204));
#38340=CARTESIAN_POINT('Ctrl Pts',(2.72654547964853,-29.0170571013445,11.868990416303));
#38341=CARTESIAN_POINT('Ctrl Pts',(2.43559675052517,-29.0287274082149,11.9320913915042));
#38342=CARTESIAN_POINT('Ctrl Pts',(2.14277402700613,-29.0403977150854,11.9844469926312));
#38343=CARTESIAN_POINT('Ctrl Pts',(1.86307404898437,-29.0515450213325,12.0344562962418));
#38344=CARTESIAN_POINT('Ctrl Pts',(1.58158081379775,-29.0626923275796,12.0746770922416));
#38345=CARTESIAN_POINT('Ctrl Pts',(1.29899467062888,-29.0738396338267,12.1050015735512));
#38346=CARTESIAN_POINT('Ctrl Pts',(1.01645652468036,-29.0849850467053,12.1353209042516));
#38347=CARTESIAN_POINT('Ctrl Pts',(0.732826106484331,-29.0961304595838,
12.1557472477031));
#38348=CARTESIAN_POINT('Ctrl Pts',(0.448809859789771,-29.1072758724624,
12.1662245565235));
#38349=CARTESIAN_POINT('Ctrl Pts',(0.164825143310763,-29.118420048027,12.1767007021999));
#38350=CARTESIAN_POINT('Ctrl Pts',(-0.119545049638622,-29.1295642235916,
12.1772300089198));
#38351=CARTESIAN_POINT('Ctrl Pts',(-0.403592042607901,-29.1407083991562,
12.1678085008412));
#38352=CARTESIAN_POINT('Ctrl Pts',(-0.696584252436126,-29.152203527449,
12.1580902903332));
#38353=CARTESIAN_POINT('Ctrl Pts',(-0.989232279100445,-29.1636986557419,
12.1377843664195));
#38354=CARTESIAN_POINT('Ctrl Pts',(-1.28076011128974,-29.1751937840348,
12.1069444447114));
#38355=CARTESIAN_POINT('Ctrl Pts',(-1.56340253921341,-29.1863385551724,
12.0770444853042));
#38356=CARTESIAN_POINT('Ctrl Pts',(-1.84499176824494,-29.19748332631,12.0372431750742));
#38357=CARTESIAN_POINT('Ctrl Pts',(-2.12482630052757,-29.2086280974475,
11.9876421135512));
#38358=CARTESIAN_POINT('Ctrl Pts',(-2.41785653186929,-29.220298404318,11.9357020959475));
#38359=CARTESIAN_POINT('Ctrl Pts',(-2.70896228484959,-29.2319687111885,
11.8730159224245));
#38360=CARTESIAN_POINT('Ctrl Pts',(-2.99734942177683,-29.243639018059,11.7997604506945));
#38361=CARTESIAN_POINT('Ctrl Pts',(-3.28573655870407,-29.2553093249295,
11.7265049789645));
#38362=CARTESIAN_POINT('Ctrl Pts',(-3.57140475656548,-29.2669796318,11.6426803001354));
#38363=CARTESIAN_POINT('Ctrl Pts',(-3.85357632161499,-29.2786499386705,
11.5485237058028));
#38364=CARTESIAN_POINT('Ctrl Pts',(-4.12310246901941,-29.2897972449176,
11.4585867055287));
#38365=CARTESIAN_POINT('Ctrl Pts',(-4.38951899259722,-29.3009445511647,
11.3591966162271));
#38366=CARTESIAN_POINT('Ctrl Pts',(-4.65215935045579,-29.3120918574118,
11.2505939233432));
#38367=CARTESIAN_POINT('Ctrl Pts',(-4.91475509888341,-29.3232372702904,
11.1420096766126));
#38368=CARTESIAN_POINT('Ctrl Pts',(-5.17357571569862,-29.334382683169,11.0242160522334));
#38369=CARTESIAN_POINT('Ctrl Pts',(-5.42797407681309,-29.3455280960475,
10.897501900502));
#38370=CARTESIAN_POINT('Ctrl Pts',(-5.68234419575679,-29.3566722716121,
10.7708018160103));
#38371=CARTESIAN_POINT('Ctrl Pts',(-5.93229280062053,-29.3678164471767,
10.6351833005706));
#38372=CARTESIAN_POINT('Ctrl Pts',(-6.17719572531623,-29.3789606227413,
10.490981995082));
#38373=CARTESIAN_POINT('Ctrl Pts',(-6.42981114063899,-29.3904557510341,
10.3422394975339));
#38374=CARTESIAN_POINT('Ctrl Pts',(-6.67705766802854,-29.401950879327,10.1843650133689));
#38375=CARTESIAN_POINT('Ctrl Pts',(-6.91827962488474,-29.4134460076198,
10.017777062897));
#38376=CARTESIAN_POINT('Ctrl Pts',(-7.15214943773357,-29.4245907787574,
9.85626650512062));
#38377=CARTESIAN_POINT('Ctrl Pts',(-7.38035625506918,-29.435735549895,9.68656592549823));
#38378=CARTESIAN_POINT('Ctrl Pts',(-7.60233273639396,-29.4468803210326,
9.50910023162826));
#38379=CARTESIAN_POINT('Ctrl Pts',(-7.83477659935983,-29.4585506279031,
9.32326607847446));
#38380=CARTESIAN_POINT('Ctrl Pts',(-8.06038815211743,-29.4702209347736,
9.12891705472717));
#38381=CARTESIAN_POINT('Ctrl Pts',(-8.27855472469325,-29.4818912416441,
8.92658848162383));
#38382=CARTESIAN_POINT('Ctrl Pts',(-8.49672129726908,-29.4935615485146,
8.72425990852047));
#38383=CARTESIAN_POINT('Ctrl Pts',(-8.70744264963618,-29.5052318553851,
8.51395202063506));
#38384=CARTESIAN_POINT('Ctrl Pts',(-8.91014947085614,-29.5169021622556,
8.29624533490916));
#38385=CARTESIAN_POINT('Ctrl Pts',(-9.10377205847044,-29.5280494685027,
8.08829509634546));
#38386=CARTESIAN_POINT('Ctrl Pts',(-9.29014048970121,-29.5391967747498,
7.87353252575311));
#38387=CARTESIAN_POINT('Ctrl Pts',(-9.46878458047568,-29.550344080997,7.65248775357047));
#38388=CARTESIAN_POINT('Ctrl Pts',(-9.64739832857408,-29.5614894938755,
7.43148052581425));
#38389=CARTESIAN_POINT('Ctrl Pts',(-9.81829018797549,-29.5726349067541,
7.2041934341806));
#38390=CARTESIAN_POINT('Ctrl Pts',(-9.98103016933431,-29.5837803196327,
6.97118978430787));
#38391=CARTESIAN_POINT('Ctrl Pts',(-10.143752084027,-29.5949244951972,6.73821200146009));
#38392=CARTESIAN_POINT('Ctrl Pts',(-10.2983237750866,-29.6060686707618,
6.49951914625352));
#38393=CARTESIAN_POINT('Ctrl Pts',(-10.4443578030689,-29.6172128463264,
6.2557046230999));
#38394=CARTESIAN_POINT('Ctrl Pts',(-10.594990739265,-29.6287079746193,6.00421188529549));
#38395=CARTESIAN_POINT('Ctrl Pts',(-10.7365394011799,-29.6402031029121,
5.74726991837197));
#38396=CARTESIAN_POINT('Ctrl Pts',(-10.868628337183,-29.651698231205,5.48555998218799));
#38397=CARTESIAN_POINT('Ctrl Pts',(-10.9966913673694,-29.6628430023426,
5.23182663803549));
#38398=CARTESIAN_POINT('Ctrl Pts',(-11.1158626482813,-29.6739877734802,
4.97361191341933));
#38399=CARTESIAN_POINT('Ctrl Pts',(-11.2258473549232,-29.6851325446178,
4.71156040117959));
#38400=CARTESIAN_POINT('Ctrl Pts',(-11.341018430374,-29.6968028514883,4.43715175465375));
#38401=CARTESIAN_POINT('Ctrl Pts',(-11.4461155690856,-29.7084731583587,
4.15853605659713));
#38402=CARTESIAN_POINT('Ctrl Pts',(-11.5408569815104,-29.7201434652292,
3.8764765422123));
#38403=CARTESIAN_POINT('Ctrl Pts',(-11.6355983939352,-29.7318137720997,
3.59441702782744));
#38404=CARTESIAN_POINT('Ctrl Pts',(-11.7199839815676,-29.7434840789702,
3.30891401794856));
#38405=CARTESIAN_POINT('Ctrl Pts',(-11.7937916549543,-29.7551543858407,
3.02074968336178));
#38406=CARTESIAN_POINT('Ctrl Pts',(-11.8651552549867,-29.7664382412116,
2.74212764620159));
#38407=CARTESIAN_POINT('Ctrl Pts',(-11.9266493212993,-29.7777220965825,
2.46094394049381));
#38408=CARTESIAN_POINT('Ctrl Pts',(-11.9781123416308,-29.7890059519535,
2.17790610019643));
#38409=CARTESIAN_POINT('Ctrl Pts',(-12.0295653763274,-29.8002876178598,
1.89492317918895));
#38410=CARTESIAN_POINT('Ctrl Pts',(-12.0709912069458,-29.8115692837662,
1.61008709067454));
#38411=CARTESIAN_POINT('Ctrl Pts',(-12.1022795090425,-29.8228509496725,
1.32411515171836));
#38412=CARTESIAN_POINT('Ctrl Pts',(-12.1335625490621,-29.8341307182245,
1.03819130761862));
#38413=CARTESIAN_POINT('Ctrl Pts',(-12.1547114378685,-29.8454104867765,
0.751132245746415));
#38414=CARTESIAN_POINT('Ctrl Pts',(-12.1656676092229,-29.8566902553285,
0.463661376334469));
#38415=CARTESIAN_POINT('Ctrl Pts',(-12.1715549693444,-29.8627515022189,
0.309187292468078));
#38416=CARTESIAN_POINT('Ctrl Pts',(-12.1745000598421,-29.8688127491093,
0.154594386717212));
#38417=CARTESIAN_POINT('Ctrl Pts',(-12.1744999999991,-29.8748739959996,
-4.71256420053583E-6));
#38418=CARTESIAN_POINT('Ctrl Pts',(-12.1734593809614,-29.8748739960349,
-4.71306082890088E-6));
#38419=CARTESIAN_POINT('Ctrl Pts',(-12.1734729483294,-29.9143848671652,
-1.00768895467666));
#38420=CARTESIAN_POINT('Ctrl Pts',(-11.8010964029253,-30.0333131461572,
-4.04082287428804));
#38421=CARTESIAN_POINT('Ctrl Pts',(-9.30992091872449,-30.2316588330109,
-8.62536224638919));
#38422=CARTESIAN_POINT('Ctrl Pts',(-4.04710485413492,-30.469911056596,-12.0288172192438));
#38423=CARTESIAN_POINT('Ctrl Pts',(2.1241845520127,-30.7051707337015,-12.4928842203625));
#38424=CARTESIAN_POINT('Ctrl Pts',(5.86746336791747,-30.8610130029453,-10.8440791401043));
#38425=CARTESIAN_POINT('Ctrl Pts',(7.41333450932841,-30.9374378643275,-9.65843860955958));
#38426=CARTESIAN_POINT('',(-12.1744999986658,-29.6251260039304,0.000180241411394071));
#38427=CARTESIAN_POINT('Ctrl Pts',(-12.1744999986658,-29.6251260039651,
0.00018024052605028));
#38428=CARTESIAN_POINT('Ctrl Pts',(-12.1745042222142,-29.6363114795878,
-0.285102936417017));
#38429=CARTESIAN_POINT('Ctrl Pts',(-12.1644766085762,-29.6474969552104,
-0.570385273907491));
#38430=CARTESIAN_POINT('Ctrl Pts',(-12.1444433863984,-29.6586824308331,
-0.854953264549404));
#38431=CARTESIAN_POINT('Ctrl Pts',(-12.1244071877467,-29.6698695683589,
-1.13956353541974));
#38432=CARTESIAN_POINT('Ctrl Pts',(-12.0943624266308,-29.6810567058848,
-1.42345898533909));
#38433=CARTESIAN_POINT('Ctrl Pts',(-12.0543873318725,-29.6922438434107,
-1.70592974743708));
#38434=CARTESIAN_POINT('Ctrl Pts',(-12.0144104223308,-29.7034314888086,
-1.98841333310159));
#38435=CARTESIAN_POINT('Ctrl Pts',(-11.9645023183561,-29.7146191342066,
-2.2694718422521));
#38436=CARTESIAN_POINT('Ctrl Pts',(-11.9047927944751,-29.7258067796045,
-2.54840318054546));
#38437=CARTESIAN_POINT('Ctrl Pts',(-11.8450710809749,-29.7369967089452,
-2.8273914622972));
#38438=CARTESIAN_POINT('Ctrl Pts',(-11.7755440050082,-29.7481866382859,
-3.10425144891475));
#38439=CARTESIAN_POINT('Ctrl Pts',(-11.6963922226106,-29.7593765676266,
-3.37829235337227));
#38440=CARTESIAN_POINT('Ctrl Pts',(-11.6752552402276,-29.7623647674141,
-3.4514732419674));
#38441=CARTESIAN_POINT('Ctrl Pts',(-11.6534321750649,-29.7653529672017,
-3.52445317187036));
#38442=CARTESIAN_POINT('Ctrl Pts',(-11.6309270707671,-29.7683411669892,
-3.59721916547995));
#38443=CARTESIAN_POINT('Ctrl Pts',(-11.5469730825569,-29.7794884732363,
-3.86866849043174));
#38444=CARTESIAN_POINT('Ctrl Pts',(-11.4534995431357,-29.7906357794834,
-4.13721802276228));
#38445=CARTESIAN_POINT('Ctrl Pts',(-11.3507321374569,-29.8017830857305,
-4.40219606488654));
#38446=CARTESIAN_POINT('Ctrl Pts',(-11.247982186809,-29.8129284986091,-4.66712910052394));
#38447=CARTESIAN_POINT('Ctrl Pts',(-11.1359416179192,-29.8240739114877,
-4.92849160846213));
#38448=CARTESIAN_POINT('Ctrl Pts',(-11.0148848982189,-29.8352193243662,
-5.18563023450271));
#38449=CARTESIAN_POINT('Ctrl Pts',(-10.8938416176952,-29.8463634999308,
-5.44274031416114));
#38450=CARTESIAN_POINT('Ctrl Pts',(-10.7637842986543,-29.8575076754954,
-5.69562720699591));
#38451=CARTESIAN_POINT('Ctrl Pts',(-10.6250346954393,-29.86865185106,-5.94365947634216));
#38452=CARTESIAN_POINT('Ctrl Pts',(-10.4819155853449,-29.8801469793528,
-6.19950278573525));
#38453=CARTESIAN_POINT('Ctrl Pts',(-10.329547980573,-29.8916421076457,-6.45018048931594));
#38454=CARTESIAN_POINT('Ctrl Pts',(-10.1683357975651,-29.9031372359385,
-6.69502780860221));
#38455=CARTESIAN_POINT('Ctrl Pts',(-10.0120371605734,-29.9142820070761,
-6.93241248736197));
#38456=CARTESIAN_POINT('Ctrl Pts',(-9.84742525859584,-29.9254267782137,
-7.16431669157156));
#38457=CARTESIAN_POINT('Ctrl Pts',(-9.67491234763068,-29.9365715493513,
-7.39016382197738));
#38458=CARTESIAN_POINT('Ctrl Pts',(-9.49426452765975,-29.9482418562218,
-7.62666085588776));
#38459=CARTESIAN_POINT('Ctrl Pts',(-9.30495281210028,-29.9599121630923,
-7.85651557113396));
#38460=CARTESIAN_POINT('Ctrl Pts',(-9.10749884104637,-29.9715824699628,
-8.07910360809534));
#38461=CARTESIAN_POINT('Ctrl Pts',(-8.91004486999248,-29.9832527768333,
-8.30169164505669));
#38462=CARTESIAN_POINT('Ctrl Pts',(-8.70444887265217,-29.9949230837037,
-8.51701275857697));
#38463=CARTESIAN_POINT('Ctrl Pts',(-8.49127863272491,-30.0065933905742,
-8.7244849378877));
#38464=CARTESIAN_POINT('Ctrl Pts',(-8.28766154076552,-30.0177406968213,
-8.92265932577667));
#38465=CARTESIAN_POINT('Ctrl Pts',(-8.07707334551595,-30.0288880030684,
-9.11373199757563));
#38466=CARTESIAN_POINT('Ctrl Pts',(-7.86003364885051,-30.0400353093155,
-9.29722115951523));
#38467=CARTESIAN_POINT('Ctrl Pts',(-7.64303081634977,-30.0511807221941,
-9.48067915584417));
#38468=CARTESIAN_POINT('Ctrl Pts',(-7.41957887379889,-30.0623261350727,
-9.656556041771));
#38469=CARTESIAN_POINT('Ctrl Pts',(-7.19023147912979,-30.0734715479513,
-9.82440947469776));
#38470=CARTESIAN_POINT('Ctrl Pts',(-6.96090954558389,-30.0846157235159,
-9.99224427328623));
#38471=CARTESIAN_POINT('Ctrl Pts',(-6.72569368202658,-30.0957598990805,
-10.1520572400168));
#38472=CARTESIAN_POINT('Ctrl Pts',(-6.48516857886181,-30.1069040746452,
-10.3034479061013));
#38473=CARTESIAN_POINT('Ctrl Pts',(-6.2370688515653,-30.118399202938,-10.4596061718149));
#38474=CARTESIAN_POINT('Ctrl Pts',(-5.98332031440759,-30.1298943312309,
-10.6068029039343));
#38475=CARTESIAN_POINT('Ctrl Pts',(-5.72459575688008,-30.1413894595237,
-10.7446476754853));
#38476=CARTESIAN_POINT('Ctrl Pts',(-5.47375680077022,-30.1525342306613,
-10.8782911105402));
#38477=CARTESIAN_POINT('Ctrl Pts',(-5.21824090472264,-30.1636790017989,
-11.0031440843534));
#38478=CARTESIAN_POINT('Ctrl Pts',(-4.95868598336946,-30.1748237729366,
-11.1188975878158));
#38479=CARTESIAN_POINT('Ctrl Pts',(-4.68689165538149,-30.186494079807,-11.240109489797));
#38480=CARTESIAN_POINT('Ctrl Pts',(-4.4106685032706,-30.1981643866775,-11.3513429650037));
#38481=CARTESIAN_POINT('Ctrl Pts',(-4.13077334331136,-30.2098346935479,
-11.4522994126153));
#38482=CARTESIAN_POINT('Ctrl Pts',(-3.85087818335214,-30.2215050004184,
-11.5532558602268));
#38483=CARTESIAN_POINT('Ctrl Pts',(-3.56731133412171,-30.2331753072889,
-11.643935174666));
#38484=CARTESIAN_POINT('Ctrl Pts',(-3.28084986321212,-30.2448456141593,
-11.7240980218122));
#38485=CARTESIAN_POINT('Ctrl Pts',(-3.0072260605414,-30.2559929204064,-11.8006683996693));
#38486=CARTESIAN_POINT('Ctrl Pts',(-2.73087965548585,-30.2671402266535,
-11.8676670436835));
#38487=CARTESIAN_POINT('Ctrl Pts',(-2.45249745078426,-30.2782875329007,
-11.9249195596405));
#38488=CARTESIAN_POINT('Ctrl Pts',(-2.17416252926519,-30.2894329457792,
-11.9821623512649));
#38489=CARTESIAN_POINT('Ctrl Pts',(-1.89379275963015,-30.3005783586578,
-12.0296622660804));
#38490=CARTESIAN_POINT('Ctrl Pts',(-1.61208596895547,-30.3117237715363,
-12.0672958478152));
#38491=CARTESIAN_POINT('Ctrl Pts',(-1.3304104521108,-30.3228679471009,-12.1049252516377));
#38492=CARTESIAN_POINT('Ctrl Pts',(-1.04739847494835,-30.3340121226655,
-12.1326904742396));
#38493=CARTESIAN_POINT('Ctrl Pts',(-0.763755074643579,-30.3451562982301,
-12.1505196776087));
#38494=CARTESIAN_POINT('Ctrl Pts',(-0.471179167432488,-30.3566514265229,
-12.1689103588125));
#38495=CARTESIAN_POINT('Ctrl Pts',(-0.177931718560926,-30.3681465548158,
-12.1767290407253));
#38496=CARTESIAN_POINT('Ctrl Pts',(0.115209683570617,-30.3796416831087,
-12.1739548618685));
#38497=CARTESIAN_POINT('Ctrl Pts',(0.399416501839786,-30.3907864542462,
-12.1712652365189));
#38498=CARTESIAN_POINT('Ctrl Pts',(0.683523362929896,-30.4019312253839,
-12.1586189056608));
#38499=CARTESIAN_POINT('Ctrl Pts',(0.96682226273384,-30.4130759965214,-12.136049808825));
#38500=CARTESIAN_POINT('Ctrl Pts',(1.26348022510615,-30.4247463033919,-12.1124164580266));
#38501=CARTESIAN_POINT('Ctrl Pts',(1.55925187642787,-30.4364166102624,-12.0779020256309));
#38502=CARTESIAN_POINT('Ctrl Pts',(1.85332979011717,-30.4480869171329,-12.0326064898286));
#38503=CARTESIAN_POINT('Ctrl Pts',(2.14740770380649,-30.4597572240034,-11.9873109540262));
#38504=CARTESIAN_POINT('Ctrl Pts',(2.43979154960903,-30.4714275308739,-11.9312343745664));
#38505=CARTESIAN_POINT('Ctrl Pts',(2.72968448063129,-30.4830978377444,-11.8645384607325));
#38506=CARTESIAN_POINT('Ctrl Pts',(3.00658378215355,-30.494245056166,-11.8008320023174));
#38507=CARTESIAN_POINT('Ctrl Pts',(3.28129325471924,-30.5053922745877,-11.7274182178329));
#38508=CARTESIAN_POINT('Ctrl Pts',(3.55312640247246,-30.5165394930093,-11.6444726380396));
#38509=CARTESIAN_POINT('Ctrl Pts',(3.82491258716696,-30.5276847855897,-11.5615413882799));
#38510=CARTESIAN_POINT('Ctrl Pts',(4.09382318417072,-30.5388300781702,-11.4690817088839));
#38511=CARTESIAN_POINT('Ctrl Pts',(4.35918639889116,-30.5499753707506,-11.3673191294044));
#38512=CARTESIAN_POINT('Ctrl Pts',(4.63242020081986,-30.5614512291078,-11.2625383046975));
#38513=CARTESIAN_POINT('Ctrl Pts',(4.90189269707538,-30.5729270874651,-11.147894395897));
#38514=CARTESIAN_POINT('Ctrl Pts',(5.16689067451331,-30.5844029458224,-11.0236877227009));
#38515=CARTESIAN_POINT('Ctrl Pts',(5.42422969768999,-30.5955471296698,-10.9030708626731));
#38516=CARTESIAN_POINT('Ctrl Pts',(5.67734896602108,-30.6066913135173,-10.7734363698508));
#38517=CARTESIAN_POINT('Ctrl Pts',(5.92561758210199,-30.6178354973647,-10.6351072641833));
#38518=CARTESIAN_POINT('Ctrl Pts',(6.18496969779133,-30.6294771929769,-10.4906027078578));
#38519=CARTESIAN_POINT('Ctrl Pts',(6.43902791382879,-30.6411188885891,-10.3366096758748));
#38520=CARTESIAN_POINT('Ctrl Pts',(6.68710279673228,-30.6527605842012,-10.1735493529021));
#38521=CARTESIAN_POINT('Ctrl Pts',(6.93517767963574,-30.6644022798134,-10.0104890299294));
#38522=CARTESIAN_POINT('Ctrl Pts',(7.17726895509336,-30.6760439754256,-9.8383616025104));
#38523=CARTESIAN_POINT('Ctrl Pts',(7.41272179941101,-30.6876856710377,-9.65763976210217));
#38524=CARTESIAN_POINT('Ctrl Pts',(7.412721799411,-27.6877007372717,-9.65763976210218));
#38525=CARTESIAN_POINT('Ctrl Pts',(7.63814987596554,-27.6988450042982,-9.48461243260574));
#38526=CARTESIAN_POINT('Ctrl Pts',(7.85753273411191,-27.7099892713247,-9.303676776569));
#38527=CARTESIAN_POINT('Ctrl Pts',(8.07032180364135,-27.7211335383512,-9.11528146771514));
#38528=CARTESIAN_POINT('Ctrl Pts',(8.28309854906444,-27.7322771599351,-8.926897070154));
#38529=CARTESIAN_POINT('Ctrl Pts',(8.48928206907873,-27.743420781519,-8.73105405962382));
#38530=CARTESIAN_POINT('Ctrl Pts',(8.68835826132702,-27.7545644031029,-8.5282402037484));
#38531=CARTESIAN_POINT('Ctrl Pts',(8.88745493347408,-27.7657091710832,-8.32540548346328));
#38532=CARTESIAN_POINT('Ctrl Pts',(9.07944262860806,-27.7768539390636,-8.11559867393501));
#38533=CARTESIAN_POINT('Ctrl Pts',(9.26384437461779,-27.7879987070439,-7.89934412801863));
#38534=CARTESIAN_POINT('Ctrl Pts',(9.44825126409226,-27.7991437858821,-7.68308355017654));
#38535=CARTESIAN_POINT('Ctrl Pts',(9.62507161081348,-27.8102888647202,-7.46037508148394));
#38536=CARTESIAN_POINT('Ctrl Pts',(9.79386837211311,-27.8214339435584,-7.23177658391923));
#38537=CARTESIAN_POINT('Ctrl Pts',(9.96269728861601,-27.8325811454958,-7.00313453912589));
#38538=CARTESIAN_POINT('Ctrl Pts',(10.1234994079084,-27.8437283474331,-6.76860043865689));
#38539=CARTESIAN_POINT('Ctrl Pts',(10.2758798621779,-27.8548755493705,-6.52876277008793));
#38540=CARTESIAN_POINT('Ctrl Pts',(10.309816736,-27.8573581590165,-6.47534817216571));
#38541=CARTESIAN_POINT('Ctrl Pts',(10.3433360636503,-27.8598407686624,-6.42167062675943));
#38542=CARTESIAN_POINT('Ctrl Pts',(10.3764337811701,-27.8623233783083,-6.36773682205794));
#38543=CARTESIAN_POINT('Ctrl Pts',(10.5250477180731,-27.8734706845554,-6.12556558943234));
#38544=CARTESIAN_POINT('Ctrl Pts',(10.6652022492297,-27.8846179908025,-5.87815325893287));
#38545=CARTESIAN_POINT('Ctrl Pts',(10.7965414680425,-27.8957652970496,-5.6261125636481));
#38546=CARTESIAN_POINT('Ctrl Pts',(10.9278583789056,-27.9069107099282,-5.37411467744341));
#38547=CARTESIAN_POINT('Ctrl Pts',(11.0503628435202,-27.9180561228068,-5.11749023242213));
#38548=CARTESIAN_POINT('Ctrl Pts',(11.1637449230493,-27.9292015356854,-4.85687652129331));
#38549=CARTESIAN_POINT('Ctrl Pts',(11.2771144154064,-27.94034571125,-4.59629174233473));
#38550=CARTESIAN_POINT('Ctrl Pts',(11.3813634385435,-27.9514898868146,-4.33171882614915));
#38551=CARTESIAN_POINT('Ctrl Pts',(11.4762297207818,-27.9626340623792,-4.06381614321381));
#38552=CARTESIAN_POINT('Ctrl Pts',(11.5740835349713,-27.9741291906721,-3.78747666054088));
#38553=CARTESIAN_POINT('Ctrl Pts',(11.6619539607177,-27.9856243189649,-3.50759456690943));
#38554=CARTESIAN_POINT('Ctrl Pts',(11.7396078726037,-27.9971194472578,-3.22491197515566));
#38555=CARTESIAN_POINT('Ctrl Pts',(11.8148949902296,-28.0082642183954,-2.95084519578442));
#38556=CARTESIAN_POINT('Ctrl Pts',(11.8805790712359,-28.019408989533,-2.67414637087701));
#38557=CARTESIAN_POINT('Ctrl Pts',(11.9364987602759,-28.0305537606706,-2.39550570776428));
#38558=CARTESIAN_POINT('Ctrl Pts',(11.9950553625732,-28.0422240675411,-2.10372564292783));
#38559=CARTESIAN_POINT('Ctrl Pts',(12.0429044652634,-28.0538943744115,-1.80981650877131));
#38560=CARTESIAN_POINT('Ctrl Pts',(12.0799209821079,-28.065564681282,-1.51458222491543));
#38561=CARTESIAN_POINT('Ctrl Pts',(12.1169374989523,-28.0772349881525,-1.21934794105955));
#38562=CARTESIAN_POINT('Ctrl Pts',(12.1431213969226,-28.0889052950229,-0.922788841490869));
#38563=CARTESIAN_POINT('Ctrl Pts',(12.158409857211,-28.1005756018934,-0.625715585608539));
#38564=CARTESIAN_POINT('Ctrl Pts',(12.1730131706264,-28.1117229081405,-0.34195556130913));
#38565=CARTESIAN_POINT('Ctrl Pts',(12.1776804928749,-28.1228702143876,-0.0576417030646985));
#38566=CARTESIAN_POINT('Ctrl Pts',(12.1723925340344,-28.1340175206348,0.226517653580774));
#38567=CARTESIAN_POINT('Ctrl Pts',(12.167105473353,-28.1451629335133,0.510628745795714));
#38568=CARTESIAN_POINT('Ctrl Pts',(12.1518665124317,-28.1563083463919,0.794585122204064));
#38569=CARTESIAN_POINT('Ctrl Pts',(12.126708476824,-28.1674537592705,1.07767887987282));
#38570=CARTESIAN_POINT('Ctrl Pts',(12.1015532341492,-28.1785979348351,1.36074120973675));
#38571=CARTESIAN_POINT('Ctrl Pts',(12.0664811392585,-28.1897421103997,1.64294084645477));
#38572=CARTESIAN_POINT('Ctrl Pts',(12.0215769591466,-28.2008862859643,1.92357419022913));
#38573=CARTESIAN_POINT('Ctrl Pts',(11.9752586551788,-28.2123814142571,2.21304524811395));
#38574=CARTESIAN_POINT('Ctrl Pts',(11.9184790037928,-28.22387654255,2.50084946845287));
#38575=CARTESIAN_POINT('Ctrl Pts',(11.8513884385692,-28.2353716708428,2.78622366800464));
#38576=CARTESIAN_POINT('Ctrl Pts',(11.7863427099908,-28.2465164419804,3.06290001832938));
#38577=CARTESIAN_POINT('Ctrl Pts',(11.711605351783,-28.257661213118,3.33729201072506));
#38578=CARTESIAN_POINT('Ctrl Pts',(11.6273649772611,-28.2688059842556,3.60871638336431));
#38579=CARTESIAN_POINT('Ctrl Pts',(11.5391522172666,-28.2804762911261,3.89293987092784));
#38580=CARTESIAN_POINT('Ctrl Pts',(11.4405187337417,-28.2921465979966,4.1739088224095));
#38581=CARTESIAN_POINT('Ctrl Pts',(11.3317394027964,-28.3038169048671,4.4508574855988));
#38582=CARTESIAN_POINT('Ctrl Pts',(11.2229600718511,-28.3154872117375,4.72780614878812));
#38583=CARTESIAN_POINT('Ctrl Pts',(11.1040350243111,-28.327157518608,5.00073421461789));
#38584=CARTESIAN_POINT('Ctrl Pts',(10.9752970363654,-28.3388278254785,5.26889981054376));
#38585=CARTESIAN_POINT('Ctrl Pts',(10.8523283952496,-28.3499751317256,5.52504766131596));
#38586=CARTESIAN_POINT('Ctrl Pts',(10.7203702820013,-28.3611224379727,5.77692701782369));
#38587=CARTESIAN_POINT('Ctrl Pts',(10.5797447276347,-28.3722697442198,6.02390668487535));
#38588=CARTESIAN_POINT('Ctrl Pts',(10.4391430585006,-28.3834151570984,6.27084440246207));
#38589=CARTESIAN_POINT('Ctrl Pts',(10.2898770193584,-28.394560569977,6.51288386038527));
#38590=CARTESIAN_POINT('Ctrl Pts',(10.1323141949373,-28.4057059828556,6.7494191827943));
#38591=CARTESIAN_POINT('Ctrl Pts',(9.97476886243749,-28.4168501584202,6.985928246108));
#38592=CARTESIAN_POINT('Ctrl Pts',(9.80892873173729,-28.4279943339848,7.21693417212102));
#38593=CARTESIAN_POINT('Ctrl Pts',(9.63520493625599,-28.4391385095494,7.44185971960963));
#38594=CARTESIAN_POINT('Ctrl Pts',(9.45601022552987,-28.4506336378422,7.67386862953165));
#38595=CARTESIAN_POINT('Ctrl Pts',(9.26842743224974,-28.4621287661351,7.89940774747275));
#38596=CARTESIAN_POINT('Ctrl Pts',(9.07295386254041,-28.4736238944279,8.1178789383812));
#38597=CARTESIAN_POINT('Ctrl Pts',(8.88343808312846,-28.4847686655655,8.32969140021755));
#38598=CARTESIAN_POINT('Ctrl Pts',(8.68650559273255,-28.4959134367031,8.53486019031293));
#38599=CARTESIAN_POINT('Ctrl Pts',(8.48264897592937,-28.5070582078407,8.73287562038785));
#38600=CARTESIAN_POINT('Ctrl Pts',(8.26917942628165,-28.5187285147112,8.94022854002452));
#38601=CARTESIAN_POINT('Ctrl Pts',(8.04811724601362,-28.5303988215817,9.13973700657199));
#38602=CARTESIAN_POINT('Ctrl Pts',(7.8200702391517,-28.5420691284522,9.33086018032282));
#38603=CARTESIAN_POINT('Ctrl Pts',(7.59202323228978,-28.5537394353226,9.52198335407365));
#38604=CARTESIAN_POINT('Ctrl Pts',(7.35699166160922,-28.5654097421931,9.70472102625269));
#38605=CARTESIAN_POINT('Ctrl Pts',(7.1156227436877,-28.5770800490636,9.87858103269464));
#38606=CARTESIAN_POINT('Ctrl Pts',(6.88507068739089,-28.5882273553107,10.0446495652055));
#38607=CARTESIAN_POINT('Ctrl Pts',(6.64866795349273,-28.5993746615578,10.2026682390773));
#38608=CARTESIAN_POINT('Ctrl Pts',(6.40699935977714,-28.6105219678049,10.3522369299497));
#38609=CARTESIAN_POINT('Ctrl Pts',(6.16537181344141,-28.6216673806835,10.5017802165991));
#38610=CARTESIAN_POINT('Ctrl Pts',(5.91848041970368,-28.632812793562,10.6428762453564));
#38611=CARTESIAN_POINT('Ctrl Pts',(5.66693787905207,-28.6439582064406,10.7751689232682));
#38612=CARTESIAN_POINT('Ctrl Pts',(5.41542326353004,-28.6551023820052,10.9074469146377));
#38613=CARTESIAN_POINT('Ctrl Pts',(5.15925876818901,-28.6662465575698,11.0309233825593));
#38614=CARTESIAN_POINT('Ctrl Pts',(4.89908162917456,-28.6773907331344,11.1452882170307));
#38615=CARTESIAN_POINT('Ctrl Pts',(4.63071098349467,-28.6888858614272,11.2632546324753));
#38616=CARTESIAN_POINT('Ctrl Pts',(4.35807113388033,-28.7003809897201,11.3715260989786));
#38617=CARTESIAN_POINT('Ctrl Pts',(4.0818849802408,-28.711876118013,11.4698153977335));
#38618=CARTESIAN_POINT('Ctrl Pts',(3.81411663566336,-28.7230208891506,11.5651089614059));
#38619=CARTESIAN_POINT('Ctrl Pts',(3.54301522272101,-28.7341656602882,11.6510197413072));
#38620=CARTESIAN_POINT('Ctrl Pts',(3.26925716994285,-28.7453104314257,11.7273359211194));
#38621=CARTESIAN_POINT('Ctrl Pts',(2.98258995670472,-28.7569807382962,11.8072508181233));
#38622=CARTESIAN_POINT('Ctrl Pts',(2.69300983150469,-28.7686510451667,11.8766443830866));
#38623=CARTESIAN_POINT('Ctrl Pts',(2.40130930024363,-28.7803213520372,11.9353325841622));
#38624=CARTESIAN_POINT('Ctrl Pts',(2.10960876898257,-28.7919916589077,11.9940207852378));
#38625=CARTESIAN_POINT('Ctrl Pts',(1.81578816230186,-28.8036619657782,12.0420035648568));
#38626=CARTESIAN_POINT('Ctrl Pts',(1.52065129953035,-28.8153322726487,12.0791584920158));
#38627=CARTESIAN_POINT('Ctrl Pts',(1.2387408895783,-28.8264795788958,12.114648334419));
#38628=CARTESIAN_POINT('Ctrl Pts',(0.955545409716465,-28.8376268851429,
12.1402700844111));
#38629=CARTESIAN_POINT('Ctrl Pts',(0.671769844144579,-28.84877419139,12.1559522673667));
#38630=CARTESIAN_POINT('Ctrl Pts',(0.388042477816734,-28.8599196042686,
12.1716317867055));
#38631=CARTESIAN_POINT('Ctrl Pts',(0.103735488728791,-28.8710650171472,
12.1773750948538));
#38632=CARTESIAN_POINT('Ctrl Pts',(-0.180442727021349,-28.8822104300257,
12.1731627226561));
#38633=CARTESIAN_POINT('Ctrl Pts',(-0.464589394575229,-28.8933546055903,
12.1689508180973));
#38634=CARTESIAN_POINT('Ctrl Pts',(-0.748607050688303,-28.9044987811549,
12.154785444124));
#38635=CARTESIAN_POINT('Ctrl Pts',(-1.03178776018388,-28.9156429567195,
12.1306992489277));
#38636=CARTESIAN_POINT('Ctrl Pts',(-1.32388640551171,-28.9271380850124,
12.1058545305128));
#38637=CARTESIAN_POINT('Ctrl Pts',(-1.61509423925137,-28.9386332133052,
12.0704540273367));
#38638=CARTESIAN_POINT('Ctrl Pts',(-1.90463906234965,-28.9501283415981,
12.0245914813008));
#38639=CARTESIAN_POINT('Ctrl Pts',(-2.1853589208235,-28.9612731127357,11.9801267683949));
#38640=CARTESIAN_POINT('Ctrl Pts',(-2.46451536486775,-28.9724178838733,
11.9258283526593));
#38641=CARTESIAN_POINT('Ctrl Pts',(-2.74141308359914,-28.9835626550109,
11.8618339456878));
#38642=CARTESIAN_POINT('Ctrl Pts',(-3.03136801487868,-28.9952329618814,
11.7948218592007));
#38643=CARTESIAN_POINT('Ctrl Pts',(-3.31884576343249,-29.0069032687519,
11.7171774140972));
#38644=CARTESIAN_POINT('Ctrl Pts',(-3.60306239103901,-29.0185735756223,
11.6291182665016));
#38645=CARTESIAN_POINT('Ctrl Pts',(-3.88727901864551,-29.0302438824928,
11.5410591189059));
#38646=CARTESIAN_POINT('Ctrl Pts',(-4.16823420743118,-29.0419141893633,
11.4425853764951));
#38647=CARTESIAN_POINT('Ctrl Pts',(-4.44516356389173,-29.0535844962338,
11.3339741988523));
#38648=CARTESIAN_POINT('Ctrl Pts',(-4.70968243040855,-29.0647318024809,
11.2302303922428));
#38649=CARTESIAN_POINT('Ctrl Pts',(-4.97060736729662,-29.075879108728,11.117206805338));
#38650=CARTESIAN_POINT('Ctrl Pts',(-5.22728514945102,-29.0870264149751,
10.9951780438667));
#38651=CARTESIAN_POINT('Ctrl Pts',(-5.48391933491689,-29.0981718278537,
10.873170008965));
#38652=CARTESIAN_POINT('Ctrl Pts',(-5.73630756506488,-29.1093172407323,
10.7421599676865));
#38653=CARTESIAN_POINT('Ctrl Pts',(-5.98381850576247,-29.1204626536109,
10.6024698226448));
#38654=CARTESIAN_POINT('Ctrl Pts',(-6.2313019689003,-29.1316068291754,10.4627951853795));
#38655=CARTESIAN_POINT('Ctrl Pts',(-6.47390899154312,-29.14275100474,10.3144424996335));
#38656=CARTESIAN_POINT('Ctrl Pts',(-6.71103358465277,-29.1538951803046,
10.1577792098304));
#38657=CARTESIAN_POINT('Ctrl Pts',(-6.95562571292541,-29.1653903085975,
9.99618227476502));
#38658=CARTESIAN_POINT('Ctrl Pts',(-7.19438425759036,-29.1768854368903,
9.82574297352866));
#38659=CARTESIAN_POINT('Ctrl Pts',(-7.42667603774404,-29.1883805651832,
9.64691314775864));
#38660=CARTESIAN_POINT('Ctrl Pts',(-7.65188785452438,-29.1995253363208,
9.47353383175558));
#38661=CARTESIAN_POINT('Ctrl Pts',(-7.87102104620591,-29.2106701074584,
9.29226805311522));
#38662=CARTESIAN_POINT('Ctrl Pts',(-8.08353098601621,-29.221814878596,9.10356946741858));
#38663=CARTESIAN_POINT('Ctrl Pts',(-8.30606190926227,-29.2334851854665,
8.90597273134222));
#38664=CARTESIAN_POINT('Ctrl Pts',(-8.52132966920872,-29.245155492337,8.70022553865971));
#38665=CARTESIAN_POINT('Ctrl Pts',(-8.7287500754548,-29.2568257992075,8.4868941533548));
#38666=CARTESIAN_POINT('Ctrl Pts',(-8.93617048170086,-29.2684961060779,
8.27356276804991));
#38667=CARTESIAN_POINT('Ctrl Pts',(-9.13574330666112,-29.2801664129484,
8.05264743678594));
#38668=CARTESIAN_POINT('Ctrl Pts',(-9.32692999639901,-29.2918367198189,
7.82475731842672));
#38669=CARTESIAN_POINT('Ctrl Pts',(-9.50954872309849,-29.302984026066,7.6070800141164));
#38670=CARTESIAN_POINT('Ctrl Pts',(-9.68457097741769,-29.3141313323131,
7.38297431499236));
#38671=CARTESIAN_POINT('Ctrl Pts',(-9.85155459629223,-29.3252786385603,
7.1529939386437));
#38672=CARTESIAN_POINT('Ctrl Pts',(-10.0185098530204,-29.3364240514388,
6.9230526244327));
#38673=CARTESIAN_POINT('Ctrl Pts',(-10.1774290435821,-29.3475694643174,
6.68723884089972));
#38674=CARTESIAN_POINT('Ctrl Pts',(-10.3279118601732,-29.358714877196,6.44613735957391));
#38675=CARTESIAN_POINT('Ctrl Pts',(-10.4783779708334,-29.3698590527605,
6.20506264425865));
#38676=CARTESIAN_POINT('Ctrl Pts',(-10.6204094365009,-29.3810032283251,
5.95870162955929));
#38677=CARTESIAN_POINT('Ctrl Pts',(-10.753649997694,-29.3921474038897,5.70766694693163));
#38678=CARTESIAN_POINT('Ctrl Pts',(-10.8910865748418,-29.4036425321825,
5.44872667216268));
#38679=CARTESIAN_POINT('Ctrl Pts',(-11.019169440786,-29.4151376604754,5.18481385036724));
#38680=CARTESIAN_POINT('Ctrl Pts',(-11.1375588475103,-29.4266327887682,
4.91662823164873));
#38681=CARTESIAN_POINT('Ctrl Pts',(-11.2523398929623,-29.4377775599059,
4.6566165756786));
#38682=CARTESIAN_POINT('Ctrl Pts',(-11.3580095056908,-29.4489223310435,
4.39258898024842));
#38683=CARTESIAN_POINT('Ctrl Pts',(-11.4543065619484,-29.4600671021811,
4.12520441128752));
#38684=CARTESIAN_POINT('Ctrl Pts',(-11.5551445408871,-29.4717374090516,
3.84521122581278));
#38685=CARTESIAN_POINT('Ctrl Pts',(-11.6457046540313,-29.483407715922,3.56153714931589));
#38686=CARTESIAN_POINT('Ctrl Pts',(-11.7257449261543,-29.4950780227925,
3.274958958028));
#38687=CARTESIAN_POINT('Ctrl Pts',(-11.8057851982772,-29.506748329663,2.98838076674009));
#38688=CARTESIAN_POINT('Ctrl Pts',(-11.8753055475832,-29.5184186365335,
2.69889878615673));
#38689=CARTESIAN_POINT('Ctrl Pts',(-11.9341245976263,-29.530088943404,2.4073056179742));
#38690=CARTESIAN_POINT('Ctrl Pts',(-11.9917048891097,-29.5415134677853,
2.12185354749385));
#38691=CARTESIAN_POINT('Ctrl Pts',(-12.0390440781821,-29.5529379921666,
1.83431123741328));
#38692=CARTESIAN_POINT('Ctrl Pts',(-12.0760155945832,-29.5643625165479,
1.54541179281881));
#38693=CARTESIAN_POINT('Ctrl Pts',(-12.1129779697708,-29.5757842162137,
1.25658377865915));
#38694=CARTESIAN_POINT('Ctrl Pts',(-12.1395777632545,-29.5872059158794,
0.966399535564798));
#38695=CARTESIAN_POINT('Ctrl Pts',(-12.1557400447632,-29.5986276155452,
0.675599151968931));
#38696=CARTESIAN_POINT('Ctrl Pts',(-12.168238897098,-29.6074604116736,0.450713138721019));
#38697=CARTESIAN_POINT('Ctrl Pts',(-12.1744966634544,-29.616293207802,0.225458828196562));
#38698=CARTESIAN_POINT('Ctrl Pts',(-12.1744999986658,-29.6251260039304,
0.000180241411402181));
#38699=CARTESIAN_POINT('Origin',(0.,-13.3748739960349,0.));
#38700=CARTESIAN_POINT('',(7.41272179941104,-24.687686530294,-9.65763976210214));
#38701=CARTESIAN_POINT('',(7.41272179941101,-24.9374329008951,-9.65763976210217));
#38702=CARTESIAN_POINT('',(7.41272179941101,-13.3748739960349,-9.65763976210217));
#38703=CARTESIAN_POINT('',(-12.1744999986836,-26.8748739959973,-0.000179033899940194));
#38704=CARTESIAN_POINT('Ctrl Pts',(7.41272179941101,-24.9374329008951,-9.65763976210217));
#38705=CARTESIAN_POINT('Ctrl Pts',(7.63819850586434,-24.9485801303023,-9.4845751067249));
#38706=CARTESIAN_POINT('Ctrl Pts',(7.85759282138039,-24.9597273597096,-9.30362524607513));
#38707=CARTESIAN_POINT('Ctrl Pts',(8.07036187721715,-24.9708745891168,-9.1152459879457));
#38708=CARTESIAN_POINT('Ctrl Pts',(8.19274451282144,-24.9772863641241,-9.00689212035723));
#38709=CARTESIAN_POINT('Ctrl Pts',(8.3129358372104,-24.9836981391314,-8.89608102723486));
#38710=CARTESIAN_POINT('Ctrl Pts',(8.43083778298808,-24.9901099141387,-8.78290524410578));
#38711=CARTESIAN_POINT('Ctrl Pts',(8.63581832193552,-25.0012572203849,-8.58614145985624));
#38712=CARTESIAN_POINT('Ctrl Pts',(8.83393818577717,-25.0124045266311,-8.38216922295967));
#38713=CARTESIAN_POINT('Ctrl Pts',(9.02469819859376,-25.0235518328773,-8.17149145959895));
#38714=CARTESIAN_POINT('Ctrl Pts',(9.21542581084571,-25.0346972457549,-7.96084947983034));
#38715=CARTESIAN_POINT('Ctrl Pts',(9.39879588886446,-25.0458426586325,-7.74350444513577));
#38716=CARTESIAN_POINT('Ctrl Pts',(9.57434752759173,-25.0569880715101,-7.5199946589674));
#38717=CARTESIAN_POINT('Ctrl Pts',(9.74987967736235,-25.0681322470739,-7.2965096858544));
#38718=CARTESIAN_POINT('Ctrl Pts',(9.91759495631258,-25.0792764226377,-7.06686153759513));
#38719=CARTESIAN_POINT('Ctrl Pts',(10.0770732542511,-25.0904205982015,-6.83162095541444));
#38720=CARTESIAN_POINT('Ctrl Pts',(10.2415738477981,-25.101915726495,-6.58897216937083));
#38721=CARTESIAN_POINT('Ctrl Pts',(10.3973100804441,-25.1134108547885,-6.34037324759497));
#38722=CARTESIAN_POINT('Ctrl Pts',(10.5438688836484,-25.1249059830821,-6.0864833208045));
#38723=CARTESIAN_POINT('Ctrl Pts',(10.6859607575327,-25.1360507542187,-5.8403316419611));
#38724=CARTESIAN_POINT('Ctrl Pts',(10.8194262115694,-25.1471955253553,-5.58920695028854));
#38725=CARTESIAN_POINT('Ctrl Pts',(10.9439347333876,-25.1583402964919,-5.3337362890709));
#38726=CARTESIAN_POINT('Ctrl Pts',(11.0743144998255,-25.1700106033639,-5.06621881593028));
#38727=CARTESIAN_POINT('Ctrl Pts',(11.1948721341598,-25.1816809102359,-4.79393592517866));
#38728=CARTESIAN_POINT('Ctrl Pts',(11.3052834849987,-25.1933512171079,-4.51763384680706));
#38729=CARTESIAN_POINT('Ctrl Pts',(11.4156948358375,-25.2050215239798,-4.24133176843546));
#38730=CARTESIAN_POINT('Ctrl Pts',(11.5159597868368,-25.2166918308518,-3.9610108172485));
#38731=CARTESIAN_POINT('Ctrl Pts',(11.6058127307487,-25.2283621377238,-3.67743947724378));
#38732=CARTESIAN_POINT('Ctrl Pts',(11.6916389471497,-25.2395094439717,-3.4065762853131));
#38733=CARTESIAN_POINT('Ctrl Pts',(11.7679914973803,-25.2506567502196,-3.13266673460072));
#38734=CARTESIAN_POINT('Ctrl Pts',(11.834672744551,-25.2618040564674,-2.85639130361768));
#38735=CARTESIAN_POINT('Ctrl Pts',(11.9013426659205,-25.2729494693468,-2.58016279798063));
#38736=CARTESIAN_POINT('Ctrl Pts',(11.9583445012586,-25.2840948822262,-2.30156947355845));
#38737=CARTESIAN_POINT('Ctrl Pts',(12.0055311474859,-25.2952402951056,-2.02130455813741));
#38738=CARTESIAN_POINT('Ctrl Pts',(12.0527125552623,-25.3063844706709,-1.7410707564762));
#38739=CARTESIAN_POINT('Ctrl Pts',(12.0900809054865,-25.3175286462363,-1.45916599735268));
#38740=CARTESIAN_POINT('Ctrl Pts',(12.1175404384541,-25.3286728218017,-1.17629246891674));
#38741=CARTESIAN_POINT('Ctrl Pts',(12.1458647278962,-25.340167950094,-0.884510678439701));
#38742=CARTESIAN_POINT('Ctrl Pts',(12.163645951052,-25.3516630783862,-0.591698407265157));
#38743=CARTESIAN_POINT('Ctrl Pts',(12.1708368293856,-25.3631582066785,-0.29863208546831));
#38744=CARTESIAN_POINT('Ctrl Pts',(12.1778085387284,-25.3743029778168,-0.0144980591447471));
#38745=CARTESIAN_POINT('Ctrl Pts',(12.1748258979266,-25.3854477489552,0.269874481842067));
#38746=CARTESIAN_POINT('Ctrl Pts',(12.1618987628609,-25.3965925200936,0.553776788898335));
#38747=CARTESIAN_POINT('Ctrl Pts',(12.148362044046,-25.4082628269628,0.851066612358317));
#38748=CARTESIAN_POINT('Ctrl Pts',(12.1239204060494,-25.419933133832,1.14784046916088));
#38749=CARTESIAN_POINT('Ctrl Pts',(12.088646326029,-25.4316034407012,1.44328800112304));
#38750=CARTESIAN_POINT('Ctrl Pts',(12.0533722460086,-25.4432737475704,1.73873553308519));
#38751=CARTESIAN_POINT('Ctrl Pts',(12.0072657724544,-25.4549440544397,2.03285640811261));
#38752=CARTESIAN_POINT('Ctrl Pts',(11.9504614375384,-25.4666143613089,2.32484874344699));
#38753=CARTESIAN_POINT('Ctrl Pts',(11.8962027685468,-25.4777616675556,2.60375554685274));
#38754=CARTESIAN_POINT('Ctrl Pts',(11.832167798918,-25.4889089738023,2.88080369527671));
#38755=CARTESIAN_POINT('Ctrl Pts',(11.7585086287844,-25.5000562800489,3.15530110715318));
#38756=CARTESIAN_POINT('Ctrl Pts',(11.6848619696517,-25.5112016929271,3.4297518956788));
#38757=CARTESIAN_POINT('Ctrl Pts',(11.6015944427383,-25.5223471058052,3.70165255508999));
#38758=CARTESIAN_POINT('Ctrl Pts',(11.5089086211831,-25.5334925186833,3.97032399172388));
#38759=CARTESIAN_POINT('Ctrl Pts',(11.4162330891935,-25.5446366942475,4.23896560165561));
#38760=CARTESIAN_POINT('Ctrl Pts',(11.3141414373819,-25.5557808698117,4.5043784525661));
#38761=CARTESIAN_POINT('Ctrl Pts',(11.2028856095872,-25.5669250453759,4.76590015301466));
#38762=CARTESIAN_POINT('Ctrl Pts',(11.0881261097483,-25.5784201736691,5.03565770311674));
#38763=CARTESIAN_POINT('Ctrl Pts',(10.9636159909716,-25.5899153019623,5.30127477407346));
#38764=CARTESIAN_POINT('Ctrl Pts',(10.8296852946106,-25.6014104302554,5.56204698557055));
#38765=CARTESIAN_POINT('Ctrl Pts',(10.6998366386309,-25.6125552013926,5.81487118569636));
#38766=CARTESIAN_POINT('Ctrl Pts',(10.5611332838991,-25.6236999725298,6.06314123540553));
#38767=CARTESIAN_POINT('Ctrl Pts',(10.4139230509799,-25.6348447436669,6.30623952433371));
#38768=CARTESIAN_POINT('Ctrl Pts',(10.2597710660175,-25.6465150505381,6.56080120144097));
#38769=CARTESIAN_POINT('Ctrl Pts',(10.0962907731105,-25.6581853574093,6.80969135715406));
#38770=CARTESIAN_POINT('Ctrl Pts',(9.92393360285792,-25.6698556642805,7.05223312831244));
#38771=CARTESIAN_POINT('Ctrl Pts',(9.75157643260539,-25.6815259711516,7.29477489947081));
#38772=CARTESIAN_POINT('Ctrl Pts',(9.57034258650591,-25.6931962780228,7.53096801767879));
#38773=CARTESIAN_POINT('Ctrl Pts',(9.38073392759741,-25.704866584894,7.76017275771763));
#38774=CARTESIAN_POINT('Ctrl Pts',(9.19962251284825,-25.7160138911413,7.97910576939872));
#38775=CARTESIAN_POINT('Ctrl Pts',(9.01081632348776,-25.7271611973886,8.19172838519732));
#38776=CARTESIAN_POINT('Ctrl Pts',(8.81478010379253,-25.738308503636,8.39750569941952));
#38777=CARTESIAN_POINT('Ctrl Pts',(8.61877718082411,-25.7494539165147,8.60324806239126));
#38778=CARTESIAN_POINT('Ctrl Pts',(8.41554686318432,-25.7605993293935,8.80214725200268));
#38779=CARTESIAN_POINT('Ctrl Pts',(8.20559199842757,-25.7717447422723,8.9937039202623));
#38780=CARTESIAN_POINT('Ctrl Pts',(7.99566044192338,-25.7828889178371,9.18523932275507));
#38781=CARTESIAN_POINT('Ctrl Pts',(7.77900602600685,-25.7940330934018,9.36943365184795));
#38782=CARTESIAN_POINT('Ctrl Pts',(7.55616695615428,-25.8051772689666,9.54582585116249));
#38783=CARTESIAN_POINT('Ctrl Pts',(7.3263102312941,-25.8166723972593,9.72777299917451));
#38784=CARTESIAN_POINT('Ctrl Pts',(7.08987323230984,-25.828167525552,9.90141845280191));
#38785=CARTESIAN_POINT('Ctrl Pts',(6.84748283278449,-25.8396626538447,10.0663016597319));
#38786=CARTESIAN_POINT('Ctrl Pts',(6.61248018993246,-25.8508074249825,10.2261594324257));
#38787=CARTESIAN_POINT('Ctrl Pts',(6.37188190783707,-25.8619521961203,10.3777810168332));
#38788=CARTESIAN_POINT('Ctrl Pts',(6.1262889482455,-25.8730969672581,10.5207905583471));
#38789=CARTESIAN_POINT('Ctrl Pts',(5.8691149634102,-25.8847672741282,10.6705437667524));
#38790=CARTESIAN_POINT('Ctrl Pts',(5.60646418974573,-25.8964375809984,10.8108530211069));
#38791=CARTESIAN_POINT('Ctrl Pts',(5.33905692026268,-25.9081078878686,10.9413400208656));
#38792=CARTESIAN_POINT('Ctrl Pts',(5.07164965077963,-25.9197781947387,11.0718270206242));
#38793=CARTESIAN_POINT('Ctrl Pts',(4.79948619084543,-25.9314485016089,11.192491626544));
#38794=CARTESIAN_POINT('Ctrl Pts',(4.52331334430271,-25.943118808479,11.3030122816554));
#38795=CARTESIAN_POINT('Ctrl Pts',(4.25951708497672,-25.9542661147261,11.4085799931869));
#38796=CARTESIAN_POINT('Ctrl Pts',(3.99198411281679,-25.9654134209732,11.5049244932549));
#38797=CARTESIAN_POINT('Ctrl Pts',(3.72137847838849,-25.9765607272202,11.5917985002581));
#38798=CARTESIAN_POINT('Ctrl Pts',(3.45081880629348,-25.9877061400987,11.6786577517222));
#38799=CARTESIAN_POINT('Ctrl Pts',(3.1771877677697,-25.9988515529772,11.7560496401096));
#38800=CARTESIAN_POINT('Ctrl Pts',(2.90116585463097,-26.0099969658557,11.8237763398131));
#38801=CARTESIAN_POINT('Ctrl Pts',(2.62517458421184,-26.0211411414202,11.891495520801));
#38802=CARTESIAN_POINT('Ctrl Pts',(2.34679322818403,-26.0322853169848,11.9495515921384));
#38803=CARTESIAN_POINT('Ctrl Pts',(2.06671500071761,-26.0434294925493,11.9977972709914));
#38804=CARTESIAN_POINT('Ctrl Pts',(1.7778165408784,-26.0549246208422,12.0475623042844));
#38805=CARTESIAN_POINT('Ctrl Pts',(1.48711289264152,-26.0664197491351,12.0868889741013));
#38806=CARTESIAN_POINT('Ctrl Pts',(1.19537488525744,-26.0779148774281,12.1156728716855));
#38807=CARTESIAN_POINT('Ctrl Pts',(0.912528688019575,-26.0890596485656,
12.1435794720163));
#38808=CARTESIAN_POINT('Ctrl Pts',(0.628710527637285,-26.1002044197031,
12.1615764172742));
#38809=CARTESIAN_POINT('Ctrl Pts',(0.344627949634741,-26.1113491908406,
12.1696212688124));
#38810=CARTESIAN_POINT('Ctrl Pts',(0.0471493544286068,-26.1230194977112,
12.1780454782484));
#38811=CARTESIAN_POINT('Ctrl Pts',(-0.250618878125068,-26.1346898045818,
12.1755564116312));
#38812=CARTESIAN_POINT('Ctrl Pts',(-0.547863251496386,-26.1463601114524,
12.1621665877285));
#38813=CARTESIAN_POINT('Ctrl Pts',(-0.845107624867718,-26.158030418323,
12.1487767638259));
#38814=CARTESIAN_POINT('Ctrl Pts',(-1.1418278042907,-26.1697007251936,12.124486206505));
#38815=CARTESIAN_POINT('Ctrl Pts',(-1.43721416924489,-26.1813710320642,
12.089369945606));
#38816=CARTESIAN_POINT('Ctrl Pts',(-1.71936290002593,-26.1925183383113,
12.0558274073648));
#38817=CARTESIAN_POINT('Ctrl Pts',(-2.00037900433124,-26.2036656445584,
12.0123981199221));
#38818=CARTESIAN_POINT('Ctrl Pts',(-2.27956106827263,-26.2148129508055,
11.9591827306892));
#38819=CARTESIAN_POINT('Ctrl Pts',(-2.55869571317629,-26.2259583636841,
11.9059763800834));
#38820=CARTESIAN_POINT('Ctrl Pts',(-2.83599667771849,-26.2371037765627,
11.8429872961325));
#38821=CARTESIAN_POINT('Ctrl Pts',(-3.11077177834321,-26.2482491894412,
11.770367419629));
#38822=CARTESIAN_POINT('Ctrl Pts',(-3.38551637466598,-26.2593933650059,
11.6977556050591));
#38823=CARTESIAN_POINT('Ctrl Pts',(-3.65773540917929,-26.2705375405707,
11.6155152010347));
#38824=CARTESIAN_POINT('Ctrl Pts',(-3.92674971415585,-26.2816817161354,
11.5238486163424));
#38825=CARTESIAN_POINT('Ctrl Pts',(-4.20423582610319,-26.2931768444282,
11.429295264676));
#38826=CARTESIAN_POINT('Ctrl Pts',(-4.47831180683099,-26.304671972721,11.3247124991547));
#38827=CARTESIAN_POINT('Ctrl Pts',(-4.74825085465912,-26.3161671010139,
11.2103775168916));
#38828=CARTESIAN_POINT('Ctrl Pts',(-5.00996249740978,-26.3273118721515,
11.0995273221062));
#38829=CARTESIAN_POINT('Ctrl Pts',(-5.26778539315621,-26.3384566432891,
10.9795106872944));
#38830=CARTESIAN_POINT('Ctrl Pts',(-5.52107796274188,-26.3496014144267,
10.8506289393438));
#38831=CARTESIAN_POINT('Ctrl Pts',(-5.78631463548927,-26.3612717212971,
10.7156697257349));
#38832=CARTESIAN_POINT('Ctrl Pts',(-6.04658315982579,-26.3729420281675,
10.5709893503964));
#38833=CARTESIAN_POINT('Ctrl Pts',(-6.30117522427095,-26.384612335038,10.4169880984397));
#38834=CARTESIAN_POINT('Ctrl Pts',(-6.55576728871611,-26.3962826419084,
10.262986846483));
#38835=CARTESIAN_POINT('Ctrl Pts',(-6.8046826107453,-26.4079529487789,10.0996648990647));
#38836=CARTESIAN_POINT('Ctrl Pts',(-7.04724619648092,-26.4196232556493,
9.92747557519963));
#38837=CARTESIAN_POINT('Ctrl Pts',(-7.27893938198356,-26.4307705618965,
9.76300285422281));
#38838=CARTESIAN_POINT('Ctrl Pts',(-7.50490681694821,-26.4419178681436,
9.59039094205251));
#38839=CARTESIAN_POINT('Ctrl Pts',(-7.72458077897762,-26.4530651743908,
9.41006387008343));
#38840=CARTESIAN_POINT('Ctrl Pts',(-7.9442174294129,-26.4642105872694,9.22976742664427));
#38841=CARTESIAN_POINT('Ctrl Pts',(-8.15756253496308,-26.4753560001481,
9.04175860884122));
#38842=CARTESIAN_POINT('Ctrl Pts',(-8.36408102412932,-26.4865014130267,
8.84650206984658));
#38843=CARTESIAN_POINT('Ctrl Pts',(-8.57057658653295,-26.4976455885913,
8.65126720736302));
#38844=CARTESIAN_POINT('Ctrl Pts',(-8.77024685209962,-26.5087897641558,
8.44878641357831));
#38845=CARTESIAN_POINT('Ctrl Pts',(-8.96259232915518,-26.5199339397204,
8.23956242717833));
#38846=CARTESIAN_POINT('Ctrl Pts',(-9.16099515603928,-26.5314290680132,
8.0237495524013));
#38847=CARTESIAN_POINT('Ctrl Pts',(-9.35160416569127,-26.542924196306,7.80076210097047));
#38848=CARTESIAN_POINT('Ctrl Pts',(-9.53391383017232,-26.5544193245989,
7.5711912754103));
#38849=CARTESIAN_POINT('Ctrl Pts',(-9.71066692374877,-26.5655640957365,
7.34861748192455));
#38850=CARTESIAN_POINT('Ctrl Pts',(-9.87961891449672,-26.5767088668741,
7.11985589637044));
#38851=CARTESIAN_POINT('Ctrl Pts',(-10.0403506524587,-26.5878536380117,
6.88547812614872));
#38852=CARTESIAN_POINT('Ctrl Pts',(-10.2086617539316,-26.5995239448822,
6.64004818700301));
#38853=CARTESIAN_POINT('Ctrl Pts',(-10.3679585107329,-26.6111942517526,
6.38845991414234));
#38854=CARTESIAN_POINT('Ctrl Pts',(-10.5178105333709,-26.622864558623,6.13140374091549));
#38855=CARTESIAN_POINT('Ctrl Pts',(-10.6676625560089,-26.6345348654935,
5.87434756768864));
#38856=CARTESIAN_POINT('Ctrl Pts',(-10.8080696830999,-26.6462051723639,
5.61182378836291));
#38857=CARTESIAN_POINT('Ctrl Pts',(-10.9386561591369,-26.6578754792344,
5.34455345956773));
#38858=CARTESIAN_POINT('Ctrl Pts',(-11.0629966322907,-26.6689875907038,
5.09006677648294));
#38859=CARTESIAN_POINT('Ctrl Pts',(-11.1784731441786,-26.6800997021732,
4.83119636045063));
#38860=CARTESIAN_POINT('Ctrl Pts',(-11.284791078264,-26.6912118136426,4.56858189922576));
#38861=CARTESIAN_POINT('Ctrl Pts',(-11.3910898863404,-26.7023219261046,
4.30601468089191));
#38862=CARTESIAN_POINT('Ctrl Pts',(-11.4882333044429,-26.7134320385665,
4.03970501227435));
#38863=CARTESIAN_POINT('Ctrl Pts',(-11.5759747961597,-26.7245421510285,
3.77031268844835));
#38864=CARTESIAN_POINT('Ctrl Pts',(-11.6637063953042,-26.7356510108608,
3.50095073774466));
#38865=CARTESIAN_POINT('Ctrl Pts',(-11.742038101081,-26.7467598706931,3.22850708261955));
#38866=CARTESIAN_POINT('Ctrl Pts',(-11.8107728310722,-26.7578687305254,
2.95365796645564));
#38867=CARTESIAN_POINT('Ctrl Pts',(-11.8795114701164,-26.7689782221362,
2.67879321918694));
#38868=CARTESIAN_POINT('Ctrl Pts',(-11.938651974578,-26.780087713747,2.40152299895952));
#38869=CARTESIAN_POINT('Ctrl Pts',(-11.9880477658973,-26.7911972053578,
2.12253645729935));
#38870=CARTESIAN_POINT('Ctrl Pts',(-12.0374432737353,-26.8023066332115,
1.84355151673624));
#38871=CARTESIAN_POINT('Ctrl Pts',(-12.0770941352764,-26.8134160610651,
1.56285054084612));
#38872=CARTESIAN_POINT('Ctrl Pts',(-12.1069051509043,-26.8245254889188,
1.28113149871751));
#38873=CARTESIAN_POINT('Ctrl Pts',(-12.136721994767,-26.8356370887331,0.9993573788041));
#38874=CARTESIAN_POINT('Ctrl Pts',(-12.1566951200387,-26.8467486885475,
0.716565063644844));
#38875=CARTESIAN_POINT('Ctrl Pts',(-12.1667811943891,-26.8578602883618,
0.433457746337774));
#38876=CARTESIAN_POINT('Ctrl Pts',(-12.1719290135767,-26.8635315242403,
0.288962947910597));
#38877=CARTESIAN_POINT('Ctrl Pts',(-12.1745021246081,-26.8692027601188,
0.144386144645321));
#38878=CARTESIAN_POINT('Ctrl Pts',(-12.1744999986836,-26.8748739959973,
-0.000179033899942618));
#38879=CARTESIAN_POINT('Ctrl Pts',(-12.1744999986836,-26.8748739960349,
-0.000179034858391824));
#38880=CARTESIAN_POINT('Ctrl Pts',(-12.1744973429416,-26.8819585649631,
-0.180771412597766));
#38881=CARTESIAN_POINT('Ctrl Pts',(-12.170475924864,-26.8890431338913,-0.361351713761423));
#38882=CARTESIAN_POINT('Ctrl Pts',(-12.1624403133837,-26.8961277028195,
-0.541752594251753));
#38883=CARTESIAN_POINT('Ctrl Pts',(-12.1497965769811,-26.9072750090666,
-0.825606683675804));
#38884=CARTESIAN_POINT('Ctrl Pts',(-12.127209485585,-26.9184223153137,-1.109060343361));
#38885=CARTESIAN_POINT('Ctrl Pts',(-12.094727685764,-26.9295696215608,-1.39140664696373));
#38886=CARTESIAN_POINT('Ctrl Pts',(-12.0622514029725,-26.9407150344394,
-1.67370499408291));
#38887=CARTESIAN_POINT('Ctrl Pts',(-12.0198837975782,-26.9518604473179,
-1.95489609573094));
#38888=CARTESIAN_POINT('Ctrl Pts',(-11.9677253505645,-26.9630058601965,
-2.23427844805787));
#38889=CARTESIAN_POINT('Ctrl Pts',(-11.9155726939485,-26.9741500357611,
-2.51362978460458));
#38890=CARTESIAN_POINT('Ctrl Pts',(-11.8536314150918,-26.9852942113258,
-2.79117251064493));
#38891=CARTESIAN_POINT('Ctrl Pts',(-11.7820532854202,-26.9964383868904,
-3.0662143808806));
#38892=CARTESIAN_POINT('Ctrl Pts',(-11.7082210150325,-27.0079335151833,
-3.3499178783647));
#38893=CARTESIAN_POINT('Ctrl Pts',(-11.6241351555881,-27.0194286434761,
-3.63096016396926));
#38894=CARTESIAN_POINT('Ctrl Pts',(-11.530018550358,-27.030923771769,-3.90859597277591));
#38895=CARTESIAN_POINT('Ctrl Pts',(-11.4387705017224,-27.0420685429066,
-4.17776978884194));
#38896=CARTESIAN_POINT('Ctrl Pts',(-11.3380941917879,-27.0532133140442,
-4.44374143924996));
#38897=CARTESIAN_POINT('Ctrl Pts',(-11.2282428127532,-27.0643580851818,
-4.70584887006112));
#38898=CARTESIAN_POINT('Ctrl Pts',(-11.1132113520216,-27.0760283920523,
-4.98031607201867));
#38899=CARTESIAN_POINT('Ctrl Pts',(-10.9881188167639,-27.0876986989227,
-5.25054555485061));
#38900=CARTESIAN_POINT('Ctrl Pts',(-10.8533121666699,-27.0993690057932,
-5.51580141618739));
#38901=CARTESIAN_POINT('Ctrl Pts',(-10.7185055165759,-27.1110393126637,
-5.78105727752418));
#38902=CARTESIAN_POINT('Ctrl Pts',(-10.5739849114736,-27.1227096195341,
-6.04133922225082));
#38903=CARTESIAN_POINT('Ctrl Pts',(-10.4201526576011,-27.1343799264046,
-6.29594066381572));
#38904=CARTESIAN_POINT('Ctrl Pts',(-10.2732143410997,-27.1455272326517,
-6.53913223294777));
#38905=CARTESIAN_POINT('Ctrl Pts',(-10.1177367424751,-27.1566745388988,
-6.77721387905434));
#38906=CARTESIAN_POINT('Ctrl Pts',(-9.95410087098509,-27.167821845146,-7.00958815482435));
#38907=CARTESIAN_POINT('Ctrl Pts',(-9.79049279302736,-27.1789672580245,
-7.24192296185269));
#38908=CARTESIAN_POINT('Ctrl Pts',(-9.61872936224129,-27.190112670903,-7.46855211592874));
#38909=CARTESIAN_POINT('Ctrl Pts',(-9.43923450693786,-27.2012580837816,
-7.68890773602035));
#38910=CARTESIAN_POINT('Ctrl Pts',(-9.2597595783524,-27.2124022593461,-7.9092388932142));
#38911=CARTESIAN_POINT('Ctrl Pts',(-9.07255510757798,-27.2235464349107,
-8.12329770037941));
#38912=CARTESIAN_POINT('Ctrl Pts',(-8.87808562861877,-27.2346906104752,
-8.33054895075426));
#38913=CARTESIAN_POINT('Ctrl Pts',(-8.67749191069513,-27.2461857387681,
-8.54432696404207));
#38914=CARTESIAN_POINT('Ctrl Pts',(-8.46916838599521,-27.257680867061,-8.75086148201259));
#38915=CARTESIAN_POINT('Ctrl Pts',(-8.25366736632376,-27.2691759953538,
-8.94960475418229));
#38916=CARTESIAN_POINT('Ctrl Pts',(-8.04473454861487,-27.2803207664914,
-9.14229057960626));
#38917=CARTESIAN_POINT('Ctrl Pts',(-7.82905548443714,-27.291465537629,-9.32765287209847));
#38918=CARTESIAN_POINT('Ctrl Pts',(-7.60716931389788,-27.3026103087666,
-9.50523146902223));
#38919=CARTESIAN_POINT('Ctrl Pts',(-7.37482002035491,-27.3142806156371,
-9.69118384921479));
#38920=CARTESIAN_POINT('Ctrl Pts',(-7.13566438620726,-27.3259509225076,
-9.86860058581242));
#38921=CARTESIAN_POINT('Ctrl Pts',(-6.89035922507428,-27.3376212293782,
-10.0370015442578));
#38922=CARTESIAN_POINT('Ctrl Pts',(-6.64505406394129,-27.3492915362487,
-10.2054025027032));
#38923=CARTESIAN_POINT('Ctrl Pts',(-6.39359965738751,-27.3609618431192,
-10.3647875003511));
#38924=CARTESIAN_POINT('Ctrl Pts',(-6.13668738798872,-27.3726321499897,
-10.5147286295035));
#38925=CARTESIAN_POINT('Ctrl Pts',(-5.89128854994562,-27.3837794562368,
-10.6579502006452));
#38926=CARTESIAN_POINT('Ctrl Pts',(-5.64083698966155,-27.3949267624839,
-10.7925985197516));
#38927=CARTESIAN_POINT('Ctrl Pts',(-5.38595316180751,-27.4060740687311,
-10.9183313188791));
#38928=CARTESIAN_POINT('Ctrl Pts',(-5.13111262593913,-27.4172194816096,
-11.0440427623067));
#38929=CARTESIAN_POINT('Ctrl Pts',(-4.87184156463934,-27.4283648944882,
-11.1608415910916));
#38930=CARTESIAN_POINT('Ctrl Pts',(-4.60878396953977,-27.4395103073668,
-11.2684320369834));
#38931=CARTESIAN_POINT('Ctrl Pts',(-4.3457555779199,-27.4506544829314,-11.3760105386643));
#38932=CARTESIAN_POINT('Ctrl Pts',(-4.07894173873217,-27.461798658496,-11.4743825978158));
#38933=CARTESIAN_POINT('Ctrl Pts',(-3.80900646198326,-27.4729428340606,
-11.5633005678556));
#38934=CARTESIAN_POINT('Ctrl Pts',(-3.53057037498807,-27.4844379623534,
-11.6550187454114));
#38935=CARTESIAN_POINT('Ctrl Pts',(-3.24881334259174,-27.4959330906463,
-11.7366776258322));
#38936=CARTESIAN_POINT('Ctrl Pts',(-2.96448245205888,-27.5074282189391,
-11.8080605537673));
#38937=CARTESIAN_POINT('Ctrl Pts',(-2.68881761199677,-27.5185729900768,
-11.877267819202));
#38938=CARTESIAN_POINT('Ctrl Pts',(-2.41073375712401,-27.5297177612144,
-11.9368161849391));
#38939=CARTESIAN_POINT('Ctrl Pts',(-2.13092449458315,-27.540862532352,-11.9865596001682));
#38940=CARTESIAN_POINT('Ctrl Pts',(-1.83792072458815,-27.5525328392224,
-12.0386486842186));
#38941=CARTESIAN_POINT('Ctrl Pts',(-1.5430252199813,-27.5642031460929,-12.0799857998834));
#38942=CARTESIAN_POINT('Ctrl Pts',(-1.24704447022982,-27.5758734529634,
-12.1104636715226));
#38943=CARTESIAN_POINT('Ctrl Pts',(-0.951063720478334,-27.5875437598338,
-12.1409415431618));
#38944=CARTESIAN_POINT('Ctrl Pts',(-0.653998060217559,-27.5992140667043,
-12.1605601451418));
#38945=CARTESIAN_POINT('Ctrl Pts',(-0.356659339898103,-27.6108843735748,
-12.1692746030839));
#38946=CARTESIAN_POINT('Ctrl Pts',(-0.0726457478549768,-27.6220316798219,
-12.177598525714));
#38947=CARTESIAN_POINT('Ctrl Pts',(0.211701791907702,-27.633178986069,-12.175976638602));
#38948=CARTESIAN_POINT('Ctrl Pts',(0.495674690478524,-27.6443262923161,
-12.1644053225474));
#38949=CARTESIAN_POINT('Ctrl Pts',(0.779599356289084,-27.6554717051947,
-12.1528359718793));
#38950=CARTESIAN_POINT('Ctrl Pts',(1.06314924152558,-27.6666171180733,-12.1313205770283));
#38951=CARTESIAN_POINT('Ctrl Pts',(1.34561734240108,-27.6777625309519,-12.0999076119543));
#38952=CARTESIAN_POINT('Ctrl Pts',(1.6280540849292,-27.6889067065165,-12.0684981342074));
#38953=CARTESIAN_POINT('Ctrl Pts',(1.90940901786181,-27.7000508820811,-12.02719330981));
#38954=CARTESIAN_POINT('Ctrl Pts',(2.18898058826488,-27.7111950576458,-11.9760934462871));
#38955=CARTESIAN_POINT('Ctrl Pts',(2.4773564353774,-27.7226901859386,-11.923384344251));
#38956=CARTESIAN_POINT('Ctrl Pts',(2.76383448278513,-27.7341853142314,-11.8602533185206));
#38957=CARTESIAN_POINT('Ctrl Pts',(3.04765506100921,-27.7456804425243,-11.7868676449303));
#38958=CARTESIAN_POINT('Ctrl Pts',(3.32282514244449,-27.7568252136619,-11.7157186750269));
#38959=CARTESIAN_POINT('Ctrl Pts',(3.59549707841157,-27.7679699847995,-11.6349309684199));
#38960=CARTESIAN_POINT('Ctrl Pts',(3.86499194570396,-27.7791147559371,-11.5447082037461));
#38961=CARTESIAN_POINT('Ctrl Pts',(4.14719494139433,-27.7907850628076,-11.4502309518185));
#38962=CARTESIAN_POINT('Ctrl Pts',(4.42591372566347,-27.8024553696781,-11.3454075047072));
#38963=CARTESIAN_POINT('Ctrl Pts',(4.70038881294249,-27.8141256765485,-11.2305296071541));
#38964=CARTESIAN_POINT('Ctrl Pts',(4.97486390022151,-27.825795983419,-11.115651709601));
#38965=CARTESIAN_POINT('Ctrl Pts',(5.24509498441225,-27.8374662902895,-10.9907194992353));
#38966=CARTESIAN_POINT('Ctrl Pts',(5.5103477343262,-27.8491365971599,-10.8560820785773));
#38967=CARTESIAN_POINT('Ctrl Pts',(5.76371078034282,-27.8602837935513,-10.7274796530913));
#38968=CARTESIAN_POINT('Ctrl Pts',(6.01260764731629,-27.8714309899427,-10.5899845344328));
#38969=CARTESIAN_POINT('Ctrl Pts',(6.25641443501615,-27.8825781863341,-10.4439326246066));
#38970=CARTESIAN_POINT('Ctrl Pts',(6.50018381863798,-27.8937236725574,-10.2979031216095));
#38971=CARTESIAN_POINT('Ctrl Pts',(6.73886445297898,-27.9048691587806,-10.1433195848208));
#38972=CARTESIAN_POINT('Ctrl Pts',(6.97185872814829,-27.9160146450039,-9.98056291622584));
#38973=CARTESIAN_POINT('Ctrl Pts',(7.12119904837047,-27.923158470664,-9.87624218564734));
#38974=CARTESIAN_POINT('Ctrl Pts',(7.26820376898424,-27.9303022963241,-9.76856458234202));
#38975=CARTESIAN_POINT('Ctrl Pts',(7.41272179941101,-27.9374461219842,-9.65763976210217));
#38976=CARTESIAN_POINT('',(-12.174499996235,-26.6251260039329,-0.000302777009382115));
#38977=CARTESIAN_POINT('Ctrl Pts',(-12.174499996235,-26.6251260039651,-0.000302777830488094));
#38978=CARTESIAN_POINT('Ctrl Pts',(-12.1744924727439,-26.6369913152146,
-0.302817471666667));
#38979=CARTESIAN_POINT('Ctrl Pts',(-12.1632051823574,-26.648856626464,-0.605278801658912));
#38980=CARTESIAN_POINT('Ctrl Pts',(-12.1406760102577,-26.6607219377135,
-0.906882717860236));
#38981=CARTESIAN_POINT('Ctrl Pts',(-12.1341314731588,-26.6641687119366,
-0.994496146796198));
#38982=CARTESIAN_POINT('Ctrl Pts',(-12.1266386202186,-26.6676154861597,
-1.08203724349874));
#38983=CARTESIAN_POINT('Ctrl Pts',(-12.1181992022146,-26.6710622603828,
-1.16948635966588));
#38984=CARTESIAN_POINT('Ctrl Pts',(-12.0909050509449,-26.6822095666301,
-1.45230792437143));
#38985=CARTESIAN_POINT('Ctrl Pts',(-12.0537015189063,-26.6933568728774,
-1.73421580133404));
#38986=CARTESIAN_POINT('Ctrl Pts',(-12.0066737159719,-26.7045041791248,
-2.01450652225056));
#38987=CARTESIAN_POINT('Ctrl Pts',(-11.9596539007038,-26.7156495920035,
-2.29474963582362));
#38988=CARTESIAN_POINT('Ctrl Pts',(-11.9028131901233,-26.7267950048823,
-2.57337587876628));
#38989=CARTESIAN_POINT('Ctrl Pts',(-11.8362881790818,-26.737940417761,-2.84968987641259));
#38990=CARTESIAN_POINT('Ctrl Pts',(-11.7697705533498,-26.7490845933258,
-3.12597319891336));
#38991=CARTESIAN_POINT('Ctrl Pts',(-11.6935708363978,-26.7602287688906,
-3.39994452942677));
#38992=CARTESIAN_POINT('Ctrl Pts',(-11.6078763665936,-26.7713729444554,
-3.67092038974925));
#38993=CARTESIAN_POINT('Ctrl Pts',(-11.5194832038473,-26.7828680727481,
-3.95042983039985));
#38994=CARTESIAN_POINT('Ctrl Pts',(-11.4209876598191,-26.7943632010408,
-4.22675179091095));
#38995=CARTESIAN_POINT('Ctrl Pts',(-11.3126507894069,-26.8058583293335,
-4.49915351671094));
#38996=CARTESIAN_POINT('Ctrl Pts',(-11.2076158915104,-26.8170031004714,
-4.763252778092));
#38997=CARTESIAN_POINT('Ctrl Pts',(-11.0933307897004,-26.8281478716092,
-5.02366697453654));
#38998=CARTESIAN_POINT('Ctrl Pts',(-10.9700825475829,-26.839292642747,-5.27974801948126));
#38999=CARTESIAN_POINT('Ctrl Pts',(-10.8410224898273,-26.8509629496171,
-5.54790465914499));
#39000=CARTESIAN_POINT('Ctrl Pts',(-10.7021337694083,-26.8626332564873,
-5.81130936507168));
#39001=CARTESIAN_POINT('Ctrl Pts',(-10.553800908055,-26.8743035633574,-6.06924514607354));
#39002=CARTESIAN_POINT('Ctrl Pts',(-10.4054680467018,-26.8859738702276,
-6.32718092707538));
#39003=CARTESIAN_POINT('Ctrl Pts',(-10.2476912192782,-26.8976441770977,
-6.57964749669029));
#39004=CARTESIAN_POINT('Ctrl Pts',(-10.0809087053182,-26.9093144839679,
-6.82596000025198));
#39005=CARTESIAN_POINT('Ctrl Pts',(-9.92160048999432,-26.9204617902149,
-7.06123409717429));
#39006=CARTESIAN_POINT('Ctrl Pts',(-9.75402843997352,-26.931609096462,-7.29096385566852));
#39007=CARTESIAN_POINT('Ctrl Pts',(-9.57860392681835,-26.9427564027091,
-7.51457231405355));
#39008=CARTESIAN_POINT('Ctrl Pts',(-9.40320920949447,-26.9539018155876,
-7.73814279257031));
#39009=CARTESIAN_POINT('Ctrl Pts',(-9.2199648564318,-26.9650472284661,-7.95559383695199));
#39010=CARTESIAN_POINT('Ctrl Pts',(-9.02932357316257,-26.9761926413446,
-8.16638023001199));
#39011=CARTESIAN_POINT('Ctrl Pts',(-8.83870345403747,-26.9873368169091,
-8.37714322250773));
#39012=CARTESIAN_POINT('Ctrl Pts',(-8.64068822334226,-26.9984809924736,
-8.58124284331955));
#39013=CARTESIAN_POINT('Ctrl Pts',(-8.43576944971309,-27.0096251680382,
-8.77816860405902));
#39014=CARTESIAN_POINT('Ctrl Pts',(-8.22439736760149,-27.0211202963311,
-8.98129595706688));
#39015=CARTESIAN_POINT('Ctrl Pts',(-8.00568009069493,-27.032615424624,-9.17679007677322));
#39016=CARTESIAN_POINT('Ctrl Pts',(-7.78019749632778,-27.0441105529169,
-9.36413248347838));
#39017=CARTESIAN_POINT('Ctrl Pts',(-7.56158732985657,-27.0552553240544,
-9.54576492757846));
#39018=CARTESIAN_POINT('Ctrl Pts',(-7.3366183506728,-27.066400095192,-9.71973503020182));
#39019=CARTESIAN_POINT('Ctrl Pts',(-7.10585275617098,-27.0775448663295,
-9.88561110188022));
#39020=CARTESIAN_POINT('Ctrl Pts',(-6.86420532619913,-27.0892151732001,
-10.0593091199987));
#39021=CARTESIAN_POINT('Ctrl Pts',(-6.61620170182717,-27.1008854800707,
-10.2241312000397));
#39022=CARTESIAN_POINT('Ctrl Pts',(-6.3625226287518,-27.1125557869413,-10.3796317877187));
#39023=CARTESIAN_POINT('Ctrl Pts',(-6.10884355567643,-27.1242260938118,
-10.5351323753978));
#39024=CARTESIAN_POINT('Ctrl Pts',(-5.84948932452369,-27.1358964006824,
-10.6813113028628));
#39025=CARTESIAN_POINT('Ctrl Pts',(-5.58517250510067,-27.147566707553,-10.8177769591662));
#39026=CARTESIAN_POINT('Ctrl Pts',(-5.33270094929267,-27.1587140138001,
-10.9481269559485));
#39027=CARTESIAN_POINT('Ctrl Pts',(-5.07562641811087,-27.1698613200473,
-11.0696540694031));
#39028=CARTESIAN_POINT('Ctrl Pts',(-4.81458622303291,-27.1810086262944,
-11.1820485489458));
#39029=CARTESIAN_POINT('Ctrl Pts',(-4.55359036559887,-27.192154039173,-11.2944239383005));
#39030=CARTESIAN_POINT('Ctrl Pts',(-4.28863043395543,-27.2032994520515,
-11.397669685218));
#39031=CARTESIAN_POINT('Ctrl Pts',(-4.02036484236643,-27.2144448649301,
-11.4915236928905));
#39032=CARTESIAN_POINT('Ctrl Pts',(-3.75212903242545,-27.2255890404947,
-11.5853672813102));
#39033=CARTESIAN_POINT('Ctrl Pts',(-3.48058854705728,-27.2367332160593,
-11.6698211243842));
#39034=CARTESIAN_POINT('Ctrl Pts',(-3.20641930561617,-27.2478773916239,
-11.7446722170766));
#39035=CARTESIAN_POINT('Ctrl Pts',(-2.92361591777954,-27.2593725199168,
-11.8218805227401));
#39036=CARTESIAN_POINT('Ctrl Pts',(-2.63801580485302,-27.2708676482096,
-11.8888713695227));
#39037=CARTESIAN_POINT('Ctrl Pts',(-2.35037625108813,-27.2823627765025,
-11.9454669949869));
#39038=CARTESIAN_POINT('Ctrl Pts',(-2.07150359171745,-27.2935075476401,
-12.0003376564636));
#39039=CARTESIAN_POINT('Ctrl Pts',(-1.79071424363557,-27.3046523187777,
-12.0454373261581));
#39040=CARTESIAN_POINT('Ctrl Pts',(-1.50870843413845,-27.3157970899153,
-12.0806559884288));
#39041=CARTESIAN_POINT('Ctrl Pts',(-1.21340453821725,-27.3274673967858,
-12.1175353995168));
#39042=CARTESIAN_POINT('Ctrl Pts',(-0.916767010429212,-27.3391377036562,
-12.1435794559706));
#39043=CARTESIAN_POINT('Ctrl Pts',(-0.619606806006443,-27.3508080105267,
-12.1587226983738));
#39044=CARTESIAN_POINT('Ctrl Pts',(-0.322446601583674,-27.3624783173972,
-12.173865940777));
#39045=CARTESIAN_POINT('Ctrl Pts',(-0.0247640560390245,-27.3741486242676,
-12.1781083608214));
#39046=CARTESIAN_POINT('Ctrl Pts',(0.272627745971015,-27.3858189311381,
-12.1714470940035));
#39047=CARTESIAN_POINT('Ctrl Pts',(0.556692040867883,-27.3969662373852,
-12.1650843494728));
#39048=CARTESIAN_POINT('Ctrl Pts',(0.840575917591387,-27.4081135436323,
-12.1487718259602));
#39049=CARTESIAN_POINT('Ctrl Pts',(1.12357154681536,-27.4192608498795,-12.1225425232988));
#39050=CARTESIAN_POINT('Ctrl Pts',(1.40651910926765,-27.430406262758,-12.0963176756811));
#39051=CARTESIAN_POINT('Ctrl Pts',(1.68857845992167,-27.4415516756366,-12.0601794363548));
#39052=CARTESIAN_POINT('Ctrl Pts',(1.96904604421539,-27.4526970885152,-12.0142127468162));
#39053=CARTESIAN_POINT('Ctrl Pts',(2.2494824922499,-27.4638412640798,-11.9682511602942));
#39054=CARTESIAN_POINT('Ctrl Pts',(2.52832726361971,-27.4749854396444,-11.9124633454658));
#39055=CARTESIAN_POINT('Ctrl Pts',(2.80488492567743,-27.4861296152089,-11.8469857264921));
#39056=CARTESIAN_POINT('Ctrl Pts',(3.09015195034886,-27.4976247435018,-11.7794460842771));
#39057=CARTESIAN_POINT('Ctrl Pts',(3.37298518903556,-27.5091198717946,-11.7015965039929));
#39058=CARTESIAN_POINT('Ctrl Pts',(3.65263463056829,-27.5206150000875,-11.6136432916451));
#39059=CARTESIAN_POINT('Ctrl Pts',(3.9237607063493,-27.5317597712251,-11.5283707833737));
#39060=CARTESIAN_POINT('Ctrl Pts',(4.19189392120769,-27.5429045423627,-11.4336014988325));
#39061=CARTESIAN_POINT('Ctrl Pts',(4.45636678338372,-27.5540493135003,-11.3295739258789));
#39062=CARTESIAN_POINT('Ctrl Pts',(4.73331095948211,-27.5657196203708,-11.2206408949202));
#39063=CARTESIAN_POINT('Ctrl Pts',(5.00624097019293,-27.5773899272413,-11.1015555262875));
#39064=CARTESIAN_POINT('Ctrl Pts',(5.27441341956734,-27.5890602341118,-10.9726484191141));
#39065=CARTESIAN_POINT('Ctrl Pts',(5.54258586894173,-27.6007305409822,-10.8437413119408));
#39066=CARTESIAN_POINT('Ctrl Pts',(5.80600045840204,-27.6124008478527,-10.7050126194888));
#39067=CARTESIAN_POINT('Ctrl Pts',(6.06394187656684,-27.6240711547232,-10.5568489222693));
#39068=CARTESIAN_POINT('Ctrl Pts',(6.31032521085729,-27.6352185274073,-10.4153242846153));
#39069=CARTESIAN_POINT('Ctrl Pts',(6.55178867359637,-27.6463659000913,-10.2651493360808));
#39070=CARTESIAN_POINT('Ctrl Pts',(6.78772652621512,-27.6575132727754,-10.1066917859068));
#39071=CARTESIAN_POINT('Ctrl Pts',(7.00070243695533,-27.6675757609408,-9.9636556402125));
#39072=CARTESIAN_POINT('Ctrl Pts',(7.20917612457296,-27.6776382491063,-9.81387125325476));
#39073=CARTESIAN_POINT('Ctrl Pts',(7.412721799411,-27.6877007372717,-9.65763976210218));
#39074=CARTESIAN_POINT('Ctrl Pts',(7.41272179941105,-24.687686530294,-9.65763976210214));
#39075=CARTESIAN_POINT('Ctrl Pts',(7.63817646864223,-24.6988315538967,-9.48459202139565));
#39076=CARTESIAN_POINT('Ctrl Pts',(7.85755693299465,-24.7099765774995,-9.30365524582674));
#39077=CARTESIAN_POINT('Ctrl Pts',(8.07031925845228,-24.7211216011022,-9.11528372112763));
#39078=CARTESIAN_POINT('Ctrl Pts',(8.28312306581052,-24.7322687976309,-8.92687546995992));
#39079=CARTESIAN_POINT('Ctrl Pts',(8.48930595663865,-24.7434159941595,-8.73102975054912));
#39080=CARTESIAN_POINT('Ctrl Pts',(8.68835882844288,-24.7545631906881,-8.52823962598488));
#39081=CARTESIAN_POINT('Ctrl Pts',(8.7507460866994,-24.7580569510261,-8.46468103595607));
#39082=CARTESIAN_POINT('Ctrl Pts',(8.8124332169472,-24.761550711364,-8.40044055336482));
#39083=CARTESIAN_POINT('Ctrl Pts',(8.87340530149632,-24.765044471702,-8.33553409238886));
#39084=CARTESIAN_POINT('Ctrl Pts',(9.0679448319984,-24.7761917778973,-8.12844141156305));
#39085=CARTESIAN_POINT('Ctrl Pts',(9.25526037748929,-24.7873390840926,-7.91450441257048));
#39086=CARTESIAN_POINT('Ctrl Pts',(9.43487941609193,-24.7984863902879,-7.69425114314608));
#39087=CARTESIAN_POINT('Ctrl Pts',(9.61446794641304,-24.8096318031139,-7.47403528372458));
#39088=CARTESIAN_POINT('Ctrl Pts',(9.78636241125291,-24.82077721594,-7.24750550239521));
#39089=CARTESIAN_POINT('Ctrl Pts',(9.95013033648356,-24.8319226287661,-7.01522319937076));
#39090=CARTESIAN_POINT('Ctrl Pts',(10.1138800809248,-24.8430668042778,-6.78296668329837));
#39091=CARTESIAN_POINT('Ctrl Pts',(10.2695049335853,-24.8542109797896,-6.54495913870715));
#39092=CARTESIAN_POINT('Ctrl Pts',(10.4166148368308,-24.8653551553013,-6.30179225229755));
#39093=CARTESIAN_POINT('Ctrl Pts',(10.5683575310261,-24.8768502836335,-6.05096754458694));
#39094=CARTESIAN_POINT('Ctrl Pts',(10.711040117134,-24.8883454119656,-5.79465352177919));
#39095=CARTESIAN_POINT('Ctrl Pts',(10.8442841370161,-24.8998405402978,-5.53352977814894));
#39096=CARTESIAN_POINT('Ctrl Pts',(10.9734670445058,-24.9109853113819,-5.28036476221359));
#39097=CARTESIAN_POINT('Ctrl Pts',(11.0937780907114,-24.922130082466,-5.02267912115243));
#39098=CARTESIAN_POINT('Ctrl Pts',(11.2049196053662,-24.9332748535501,-4.76111613881459));
#39099=CARTESIAN_POINT('Ctrl Pts',(11.321302039945,-24.9449451605063,-4.4872190556702));
#39100=CARTESIAN_POINT('Ctrl Pts',(11.4276292249518,-24.9566154674625,-4.20907045001993));
#39101=CARTESIAN_POINT('Ctrl Pts',(11.5236160012056,-24.9682857744186,-3.92743230454166));
#39102=CARTESIAN_POINT('Ctrl Pts',(11.6196027774595,-24.9799560813748,-3.64579415906338));
#39103=CARTESIAN_POINT('Ctrl Pts',(11.7052490450382,-24.991626388331,-3.36066679415295));
#39104=CARTESIAN_POINT('Ctrl Pts',(11.7803292606082,-25.0032966952871,-3.07283139167434));
#39105=CARTESIAN_POINT('Ctrl Pts',(11.8520447828511,-25.0144440015614,-2.79789523103511));
#39106=CARTESIAN_POINT('Ctrl Pts',(11.9141418832278,-25.0255913078357,-2.52040630438659));
#39107=CARTESIAN_POINT('Ctrl Pts',(11.9664583505487,-25.03673861411,-2.24105439349054));
#39108=CARTESIAN_POINT('Ctrl Pts',(12.0187659319259,-25.047884027016,-1.96174993047246));
#39109=CARTESIAN_POINT('Ctrl Pts',(12.0612961478269,-25.0590294399221,-1.680583377044));
#39110=CARTESIAN_POINT('Ctrl Pts',(12.0939379121453,-25.0701748528282,-1.39825463602789));
#39111=CARTESIAN_POINT('Ctrl Pts',(12.1265760527213,-25.0813190284204,-1.11595723788416));
#39112=CARTESIAN_POINT('Ctrl Pts',(12.1493279031616,-25.0924632040126,-0.832498174701055));
#39113=CARTESIAN_POINT('Ctrl Pts',(12.1621341151456,-25.1036073796049,-0.548583644680526));
#39114=CARTESIAN_POINT('Ctrl Pts',(12.1753436207048,-25.1151025078772,-0.255728070579462));
#39115=CARTESIAN_POINT('Ctrl Pts',(12.1779708973995,-25.1265976361494,0.0376118263910138));
#39116=CARTESIAN_POINT('Ctrl Pts',(12.1700088495403,-25.1380927644217,0.330658210410661));
#39117=CARTESIAN_POINT('Ctrl Pts',(12.1622894749236,-25.1492375355872,0.61477290782209));
#39118=CARTESIAN_POINT('Ctrl Pts',(12.1446167235003,-25.1603823067528,0.898611440186133));
#39119=CARTESIAN_POINT('Ctrl Pts',(12.1170370604352,-25.1715270779183,1.18146651498856));
#39120=CARTESIAN_POINT('Ctrl Pts',(12.0881568685195,-25.1831973847439,1.47765972174982));
#39121=CARTESIAN_POINT('Ctrl Pts',(12.0484129862963,-25.1948676915696,1.77277417226269));
#39122=CARTESIAN_POINT('Ctrl Pts',(11.9979196669199,-25.2065379983952,2.06600433594332));
#39123=CARTESIAN_POINT('Ctrl Pts',(11.9474263475436,-25.2182083052209,2.35923449962396));
#39124=CARTESIAN_POINT('Ctrl Pts',(11.8861836565992,-25.2298786120466,2.65058004732725));
#39125=CARTESIAN_POINT('Ctrl Pts',(11.814367381413,-25.2415489188722,2.93924711907746));
#39126=CARTESIAN_POINT('Ctrl Pts',(11.7457695266862,-25.2526962251084,3.21497768016523));
#39127=CARTESIAN_POINT('Ctrl Pts',(11.6675044717985,-25.2638435313446,3.48834690833357));
#39128=CARTESIAN_POINT('Ctrl Pts',(11.5797598749238,-25.2749908375808,3.75867150587886));
#39129=CARTESIAN_POINT('Ctrl Pts',(11.4920301814584,-25.2861362504483,4.02895018882332));
#39130=CARTESIAN_POINT('Ctrl Pts',(11.3948242428908,-25.2972816633159,4.29618501997487));
#39131=CARTESIAN_POINT('Ctrl Pts',(11.2883794518641,-25.3084270761834,4.55970828022289));
#39132=CARTESIAN_POINT('Ctrl Pts',(11.1819464778628,-25.319571251737,4.82320228529501));
#39133=CARTESIAN_POINT('Ctrl Pts',(11.0662767993538,-25.3307154272905,5.08298529497744));
#39134=CARTESIAN_POINT('Ctrl Pts',(10.9416562506894,-25.3418596028441,5.33840882115168));
#39135=CARTESIAN_POINT('Ctrl Pts',(10.8131111475577,-25.3533547311452,5.60187615351543));
#39136=CARTESIAN_POINT('Ctrl Pts',(10.6750423980179,-25.3648498594463,5.86070470407446));
#39137=CARTESIAN_POINT('Ctrl Pts',(10.5278159992574,-25.3763449877474,6.11420808737982));
#39138=CARTESIAN_POINT('Ctrl Pts',(10.3850768775203,-25.3874897588738,6.35998500371434));
#39139=CARTESIAN_POINT('Ctrl Pts',(10.233730207958,-25.3986345300003,6.60075631358498));
#39140=CARTESIAN_POINT('Ctrl Pts',(10.0741552596408,-25.4097793011267,6.83592320426813));
#39141=CARTESIAN_POINT('Ctrl Pts',(9.90705549622338,-25.4214496080151,7.08217947576419));
#39142=CARTESIAN_POINT('Ctrl Pts',(9.7309329452156,-25.4331199149036,7.322289790146));
#39143=CARTESIAN_POINT('Ctrl Pts',(9.54627340902399,-25.444790221792,7.55560151478104));
#39144=CARTESIAN_POINT('Ctrl Pts',(9.36161387283237,-25.4564605286804,7.7889132394161));
#39145=CARTESIAN_POINT('Ctrl Pts',(9.16841756655482,-25.4681308355689,8.01542611667906));
#39146=CARTESIAN_POINT('Ctrl Pts',(8.96721873867355,-25.4798011424573,8.2345272082119));
#39147=CARTESIAN_POINT('Ctrl Pts',(8.77503656446375,-25.4909484487072,8.44380936251634));
#39148=CARTESIAN_POINT('Ctrl Pts',(8.57549596571777,-25.5020957549571,8.64639194661431));
#39149=CARTESIAN_POINT('Ctrl Pts',(8.36908870550682,-25.513243061207,8.84176478364802));
#39150=CARTESIAN_POINT('Ctrl Pts',(8.16271650354294,-25.5243884740884,9.03710443663004));
#39151=CARTESIAN_POINT('Ctrl Pts',(7.94948016228736,-25.5355338869697,9.22523660411083));
#39152=CARTESIAN_POINT('Ctrl Pts',(7.72990765985017,-25.5466792998511,9.405688588306));
#39153=CARTESIAN_POINT('Ctrl Pts',(7.51035953337008,-25.5578234754185,9.58612053952902));
#39154=CARTESIAN_POINT('Ctrl Pts',(7.28447685633972,-25.568967650986,9.75887384069091));
#39155=CARTESIAN_POINT('Ctrl Pts',(7.05282093895285,-25.5801118265534,9.92351586148116));
#39156=CARTESIAN_POINT('Ctrl Pts',(6.81386970621674,-25.5916069548442,10.0933427939065));
#39157=CARTESIAN_POINT('Ctrl Pts',(6.56877595494297,-25.6031020831349,10.2545391062418));
#39158=CARTESIAN_POINT('Ctrl Pts',(6.31818951893443,-25.6145972114257,10.4066772532268));
#39159=CARTESIAN_POINT('Ctrl Pts',(6.07524064445653,-25.6257419825661,10.5541784195464));
#39160=CARTESIAN_POINT('Ctrl Pts',(5.82712918612301,-25.6368867537066,10.6931652624018));
#39161=CARTESIAN_POINT('Ctrl Pts',(5.57447472401811,-25.648031524847,10.8232934821746));
#39162=CARTESIAN_POINT('Ctrl Pts',(5.30990624911238,-25.6597018317129,10.9595579453496));
#39163=CARTESIAN_POINT('Ctrl Pts',(5.04035628966013,-25.6713721385788,11.086108073986));
#39164=CARTESIAN_POINT('Ctrl Pts',(4.76656372398074,-25.6830424454447,11.2026032918796));
#39165=CARTESIAN_POINT('Ctrl Pts',(4.49277115830137,-25.6947127523106,11.3190985097732));
#39166=CARTESIAN_POINT('Ctrl Pts',(4.21473629854935,-25.7063830591765,11.4255386936459));
#39167=CARTESIAN_POINT('Ctrl Pts',(3.9332215664071,-25.7180533660424,11.5216413049335));
#39168=CARTESIAN_POINT('Ctrl Pts',(3.66432281606581,-25.7292006722898,11.613437112148));
#39169=CARTESIAN_POINT('Ctrl Pts',(3.39216892641119,-25.7403479785372,11.6958289457042));
#39170=CARTESIAN_POINT('Ctrl Pts',(3.11743583844296,-25.7514952847845,11.7686041671556));
#39171=CARTESIAN_POINT('Ctrl Pts',(2.84274941385565,-25.7626406976633,11.8413670277446));
#39172=CARTESIAN_POINT('Ctrl Pts',(2.56548492333052,-25.7737861105421,11.9045164689942));
#39173=CARTESIAN_POINT('Ctrl Pts',(2.28633217166219,-25.7849315234209,11.9578900919361));
#39174=CARTESIAN_POINT('Ctrl Pts',(2.00721041028548,-25.7960756989858,12.0112577895767));
#39175=CARTESIAN_POINT('Ctrl Pts',(1.72620106829005,-25.8072198745506,12.0548517859353));
#39176=CARTESIAN_POINT('Ctrl Pts',(1.44400404418548,-25.8183640501154,12.0885608146866));
#39177=CARTESIAN_POINT('Ctrl Pts',(1.15292006251107,-25.8298591784081,12.1233314092329));
#39178=CARTESIAN_POINT('Ctrl Pts',(0.860572674978458,-25.8413543067008,
12.1475843071283));
#39179=CARTESIAN_POINT('Ctrl Pts',(0.567737076103554,-25.8528494349934,
12.1612550693758));
#39180=CARTESIAN_POINT('Ctrl Pts',(0.283826740576818,-25.8639942061314,
12.1745091638625));
#39181=CARTESIAN_POINT('Ctrl Pts',(-0.000542208066812766,-25.8751389772693,
12.177816618211));
#39182=CARTESIAN_POINT('Ctrl Pts',(-0.284660976616601,-25.8862837484072,
12.1711716107527));
#39183=CARTESIAN_POINT('Ctrl Pts',(-0.58217746892358,-25.8979540552772,
12.1642132555533));
#39184=CARTESIAN_POINT('Ctrl Pts',(-0.879419300969854,-25.9096243621473,
12.1463412370951));
#39185=CARTESIAN_POINT('Ctrl Pts',(-1.1755747098368,-25.9212946690173,12.1176100924065));
#39186=CARTESIAN_POINT('Ctrl Pts',(-1.47173011870375,-25.9329649758874,
12.0888789477179));
#39187=CARTESIAN_POINT('Ctrl Pts',(-1.76679877130586,-25.9446352827574,
12.049288717932));
#39188=CARTESIAN_POINT('Ctrl Pts',(-2.05997600562754,-25.9563055896275,
11.9989561673605));
#39189=CARTESIAN_POINT('Ctrl Pts',(-2.34001460716483,-25.9674528958737,
11.9508792520214));
#39190=CARTESIAN_POINT('Ctrl Pts',(-2.61841122729086,-25.9786002021199,
11.8929873201505));
#39191=CARTESIAN_POINT('Ctrl Pts',(-2.89447058978094,-25.9897475083661,
11.8254171281563));
#39192=CARTESIAN_POINT('Ctrl Pts',(-3.1704830636217,-26.0008929212437,11.7578584129511));
#39193=CARTESIAN_POINT('Ctrl Pts',(-3.44415881340236,-26.0120383341213,
11.6806247829658));
#39194=CARTESIAN_POINT('Ctrl Pts',(-3.71481443133084,-26.0231837469989,
11.5939037425181));
#39195=CARTESIAN_POINT('Ctrl Pts',(-3.98544000228493,-26.0343279225626,
11.5071923294519));
#39196=CARTESIAN_POINT('Ctrl Pts',(-4.2530458569297,-26.0454720981264,11.4109956904676));
#39197=CARTESIAN_POINT('Ctrl Pts',(-4.51696419369567,-26.0566162736902,
11.3055510579039));
#39198=CARTESIAN_POINT('Ctrl Pts',(-4.78919385508069,-26.0681114019837,
11.1967857596322));
#39199=CARTESIAN_POINT('Ctrl Pts',(-5.05749970103818,-26.0796065302773,
11.0781806539576));
#39200=CARTESIAN_POINT('Ctrl Pts',(-5.32117022414081,-26.0911016585708,
10.9500501229774));
#39201=CARTESIAN_POINT('Ctrl Pts',(-5.57680439893524,-26.1022464297075,
10.8258248505894));
#39202=CARTESIAN_POINT('Ctrl Pts',(-5.82808137347083,-26.1133912008442,
10.6926463228217));
#39203=CARTESIAN_POINT('Ctrl Pts',(-6.07437599582975,-26.1245359719809,
10.5508486156938));
#39204=CARTESIAN_POINT('Ctrl Pts',(-6.33228473065996,-26.1362062788529,
10.4023643861279));
#39205=CARTESIAN_POINT('Ctrl Pts',(-6.58472964220962,-26.1478765857248,
10.2444286953403));
#39206=CARTESIAN_POINT('Ctrl Pts',(-6.83102404875189,-26.1595468925968,
10.0774778935691));
#39207=CARTESIAN_POINT('Ctrl Pts',(-7.07731845529416,-26.1712171994687,
9.91052709179783));
#39208=CARTESIAN_POINT('Ctrl Pts',(-7.31746208404252,-26.1828875063407,
9.73456137455619));
#39209=CARTESIAN_POINT('Ctrl Pts',(-7.55080426673173,-26.1945578132126,
9.55006833355165));
#39210=CARTESIAN_POINT('Ctrl Pts',(-7.77368930304789,-26.2057051194604,
9.37384328212515));
#39211=CARTESIAN_POINT('Ctrl Pts',(-7.99043566959423,-26.2168524257083,
9.18978577348594));
#39212=CARTESIAN_POINT('Ctrl Pts',(-8.20049831293366,-26.2279997319561,
8.99834860791536));
#39213=CARTESIAN_POINT('Ctrl Pts',(-8.41052527716152,-26.2391451448355,
8.80694395792146));
#39214=CARTESIAN_POINT('Ctrl Pts',(-8.61387058758587,-26.2502905577149,
8.60816233308373));
#39215=CARTESIAN_POINT('Ctrl Pts',(-8.81002389705792,-26.2614359705943,
8.40249541405816));
#39216=CARTESIAN_POINT('Ctrl Pts',(-9.00615543046492,-26.2725801461596,
8.19685132725613));
#39217=CARTESIAN_POINT('Ctrl Pts',(-9.19509637319099,-26.283724321725,7.98432366558186));
#39218=CARTESIAN_POINT('Ctrl Pts',(-9.37637387833569,-26.2948684972904,
7.76544030584642));
#39219=CARTESIAN_POINT('Ctrl Pts',(-9.56336018036558,-26.3063636255827,
7.53966386447199));
#39220=CARTESIAN_POINT('Ctrl Pts',(-9.74219235219411,-26.3178587538749,
7.30712515292804));
#39221=CARTESIAN_POINT('Ctrl Pts',(-9.91239608982264,-26.3293538821672,
7.06844070559192));
#39222=CARTESIAN_POINT('Ctrl Pts',(-10.0774122300974,-26.3404986533055,
6.83703106211519));
#39223=CARTESIAN_POINT('Ctrl Pts',(-10.2343179534282,-26.3516434244438,
6.59984499127896));
#39224=CARTESIAN_POINT('Ctrl Pts',(-10.3827242058869,-26.3627881955821,
6.35747499519189));
#39225=CARTESIAN_POINT('Ctrl Pts',(-10.5381286090834,-26.3744585024514,
6.10367595390744));
#39226=CARTESIAN_POINT('Ctrl Pts',(-10.6842124964244,-26.3861288093207,
5.84419259488536));
#39227=CARTESIAN_POINT('Ctrl Pts',(-10.8205817294359,-26.3977991161899,
5.57973666821271));
#39228=CARTESIAN_POINT('Ctrl Pts',(-10.9569509624474,-26.4094694230592,
5.31528074154007));
#39229=CARTESIAN_POINT('Ctrl Pts',(-11.0836053951668,-26.4211397299285,
5.04585254943003));
#39230=CARTESIAN_POINT('Ctrl Pts',(-11.2002070324854,-26.4328100367977,
4.77219160129437));
#39231=CARTESIAN_POINT('Ctrl Pts',(-11.311144830923,-26.4439134670834,4.51182353269197));
#39232=CARTESIAN_POINT('Ctrl Pts',(-11.4130186487047,-26.4550168973691,
4.24754059388121));
#39233=CARTESIAN_POINT('Ctrl Pts',(-11.5055675162661,-26.4661203276549,
3.97999577620921));
#39234=CARTESIAN_POINT('Ctrl Pts',(-11.5980993129953,-26.4772217098896,
3.71250030773821));
#39235=CARTESIAN_POINT('Ctrl Pts',(-11.6813095047598,-26.4883230921244,
3.44174441751769));
#39236=CARTESIAN_POINT('Ctrl Pts',(-11.7549861724547,-26.4994244743592,
3.16839870208905));
#39237=CARTESIAN_POINT('Ctrl Pts',(-11.8286604607754,-26.5105254980769,
2.89506181430902));
#39238=CARTESIAN_POINT('Ctrl Pts',(-11.8928017662328,-26.5216265217947,
2.61913552911646));
#39239=CARTESIAN_POINT('Ctrl Pts',(-11.9472483674234,-26.5327275455124,
2.34130448619971));
#39240=CARTESIAN_POINT('Ctrl Pts',(-12.0016914005901,-26.5438278417519,
2.06349165025601));
#39241=CARTESIAN_POINT('Ctrl Pts',(-12.0464409474768,-26.5549281379914,
1.78377457205652));
#39242=CARTESIAN_POINT('Ctrl Pts',(-12.0813864435219,-26.5660284342308,
1.50284791389073));
#39243=CARTESIAN_POINT('Ctrl Pts',(-12.1163370539098,-26.5771303550208,
1.22188014154935));
#39244=CARTESIAN_POINT('Ctrl Pts',(-12.1414807111354,-26.5882322758107,
0.939702704299309));
#39245=CARTESIAN_POINT('Ctrl Pts',(-12.1567585846212,-26.5993341966006,
0.657016716103665));
#39246=CARTESIAN_POINT('Ctrl Pts',(-12.1685896895518,-26.6079314657114,
0.438106172572895));
#39247=CARTESIAN_POINT('Ctrl Pts',(-12.1745054475292,-26.6165287348221,
0.218890818353648));
#39248=CARTESIAN_POINT('Ctrl Pts',(-12.174499996235,-26.6251260039329,-0.000302777009381836));
#39249=CARTESIAN_POINT('Origin',(0.,-13.3748739960349,0.));
#39250=CARTESIAN_POINT('',(7.41324263166141,-21.6876995907947,-9.65831743152016));
#39251=CARTESIAN_POINT('',(7.41272179941102,-21.9374490664136,-9.65763976210216));
#39252=CARTESIAN_POINT('',(7.41272179941101,-13.3748739960349,-9.65763976210217));
#39253=CARTESIAN_POINT('',(-12.1737246773372,-20.6251260039651,-0.000249401258526419));
#39254=CARTESIAN_POINT('Ctrl Pts',(-12.1737246773372,-20.6251260039651,
-0.000249401258526419));
#39255=CARTESIAN_POINT('Ctrl Pts',(-12.1741911104616,-20.6550028928951,
-0.762156362199578));
#39256=CARTESIAN_POINT('Ctrl Pts',(-11.9165818304369,-20.7642971896869,
-3.54900219940989));
#39257=CARTESIAN_POINT('Ctrl Pts',(-9.8146932898574,-20.9530088943404,-8.04643346012397));
#39258=CARTESIAN_POINT('Ctrl Pts',(-4.76736202235426,-21.1912611179255,
-11.7619196070543));
#39259=CARTESIAN_POINT('Ctrl Pts',(1.44252672235886,-21.4295133415106,-12.6091655852676));
#39260=CARTESIAN_POINT('Ctrl Pts',(5.51132592543989,-21.594992832467,-11.0618012110311));
#39261=CARTESIAN_POINT('Ctrl Pts',(7.27894291850697,-21.6810549155617,-9.7615477464203));
#39262=CARTESIAN_POINT('Ctrl Pts',(7.41324263166141,-21.6876995907947,-9.65831743152016));
#39263=CARTESIAN_POINT('',(-3.14788895504393,-20.,11.7604951161383));
#39264=CARTESIAN_POINT('Ctrl Pts',(-3.14788895504386,-20.,11.7604951161383));
#39265=CARTESIAN_POINT('Ctrl Pts',(-5.10402892604601,-20.0794174078617,
11.2369022445433));
#39266=CARTESIAN_POINT('Ctrl Pts',(-8.7479903792511,-20.2382522235851,9.19518133472436));
#39267=CARTESIAN_POINT('Ctrl Pts',(-11.6635919119852,-20.4466275582401,
4.5523794220281));
#39268=CARTESIAN_POINT('Ctrl Pts',(-12.1729512588234,-20.5755854850334,
1.26311059284835));
#39269=CARTESIAN_POINT('Ctrl Pts',(-12.1737246773372,-20.6251260039651,
-0.000249401258526419));
#39270=CARTESIAN_POINT('',(3.14799128255578,-20.,11.7604677260283));
#39271=CARTESIAN_POINT('Origin',(0.,-20.,0.));
#39272=CARTESIAN_POINT('',(-12.1744999960254,-20.8748739960726,-0.000311090449405607));
#39273=CARTESIAN_POINT('Ctrl Pts',(3.14799128255578,-20.,11.7604677260283));
#39274=CARTESIAN_POINT('Ctrl Pts',(2.87408896340417,-20.0111238078539,11.8337847175841));
#39275=CARTESIAN_POINT('Ctrl Pts',(2.59758120573957,-20.0222476157078,11.8975402035724));
#39276=CARTESIAN_POINT('Ctrl Pts',(2.3191538849406,-20.0333714235617,11.9515679100261));
#39277=CARTESIAN_POINT('Ctrl Pts',(2.04077383251934,-20.0444933429358,12.0055864442404));
#39278=CARTESIAN_POINT('Ctrl Pts',(1.76047513153612,-20.05561526231,12.0498804447393));
#39279=CARTESIAN_POINT('Ctrl Pts',(1.47895412675117,-20.0667371816841,12.0843346916976));
#39280=CARTESIAN_POINT('Ctrl Pts',(1.19746278684058,-20.0778579291019,12.1187853080887));
#39281=CARTESIAN_POINT('Ctrl Pts',(0.914749667258382,-20.0889786765196,
12.1433982086866));
#39282=CARTESIAN_POINT('Ctrl Pts',(0.631517738404003,-20.1000994239374,
12.1581098693868));
#39283=CARTESIAN_POINT('Ctrl Pts',(0.348264204419321,-20.1112210196536,
12.1728226523028));
#39284=CARTESIAN_POINT('Ctrl Pts',(0.0644920506102684,-20.1223426153698,
12.1776326690876));
#39285=CARTESIAN_POINT('Ctrl Pts',(-0.219092759740573,-20.1334642110859,
12.1725284395901));
#39286=CARTESIAN_POINT('Ctrl Pts',(-0.502675706866799,-20.1445857337304,
12.1674242436287));
#39287=CARTESIAN_POINT('Ctrl Pts',(-0.786071044024664,-20.1557072563748,
12.1524059386502));
#39288=CARTESIAN_POINT('Ctrl Pts',(-1.06857402377094,-20.1668287790193,
12.1275141643175));
#39289=CARTESIAN_POINT('Ctrl Pts',(-1.3511407675224,-20.1779528119128,12.1026167716397));
#39290=CARTESIAN_POINT('Ctrl Pts',(-1.63281448316961,-20.1890768448062,
12.0678414788482));
#39291=CARTESIAN_POINT('Ctrl Pts',(-1.91289517693805,-20.2002008776997,
12.0232808455948));
#39292=CARTESIAN_POINT('Ctrl Pts',(-2.12157502678727,-20.2084890659454,
11.9900800343165));
#39293=CARTESIAN_POINT('Ctrl Pts',(-2.32937062841864,-20.216777254191,11.9514481621977));
#39294=CARTESIAN_POINT('Ctrl Pts',(-2.53599567615223,-20.2250654424367,
11.90744205027));
#39295=CARTESIAN_POINT('Ctrl Pts',(-2.8138996165917,-20.2362127849193,11.8482552670494));
#39296=CARTESIAN_POINT('Ctrl Pts',(-3.08977208840528,-20.2473601274019,
11.7793265425912));
#39297=CARTESIAN_POINT('Ctrl Pts',(-3.36292380790864,-20.2585074698845,
11.700820215361));
#39298=CARTESIAN_POINT('Ctrl Pts',(-3.63602920899082,-20.2696529221088,
11.6223272004729));
#39299=CARTESIAN_POINT('Ctrl Pts',(-3.90641452259799,-20.2807983743331,
11.5342598989376));
#39300=CARTESIAN_POINT('Ctrl Pts',(-4.17340434525454,-20.2919438265575,
11.4368328841953));
#39301=CARTESIAN_POINT('Ctrl Pts',(-4.44036459984081,-20.3030880444669,
11.3394166591108));
#39302=CARTESIAN_POINT('Ctrl Pts',(-4.70392986384688,-20.3142322623763,
11.2326428820654));
#39303=CARTESIAN_POINT('Ctrl Pts',(-4.96344230817088,-20.3253764802857,
11.1167751935289));
#39304=CARTESIAN_POINT('Ctrl Pts',(-5.23112562291956,-20.3368715790971,
10.997259356743));
#39305=CARTESIAN_POINT('Ctrl Pts',(-5.49449649858205,-20.3483666779084,
10.8680677908846));
#39306=CARTESIAN_POINT('Ctrl Pts',(-5.75285652074203,-20.3598617767197,
10.7295429586612));
#39307=CARTESIAN_POINT('Ctrl Pts',(-6.00334380137697,-20.3710065971057,
10.5952392524068));
#39308=CARTESIAN_POINT('Ctrl Pts',(-6.24912084279396,-20.3821514174916,
10.4521627969437));
#39309=CARTESIAN_POINT('Ctrl Pts',(-6.48957628823896,-20.3932962378776,
10.300672300832));
#39310=CARTESIAN_POINT('Ctrl Pts',(-6.74136789952925,-20.4049664759016,
10.1420398521446));
#39311=CARTESIAN_POINT('Ctrl Pts',(-6.98732380660455,-20.4166367139256,
9.97418109459479));
#39312=CARTESIAN_POINT('Ctrl Pts',(-7.22677526496622,-20.4283069519497,
9.79755936545793));
#39313=CARTESIAN_POINT('Ctrl Pts',(-7.4662267233279,-20.4399771899737,9.62093763632107));
#39314=CARTESIAN_POINT('Ctrl Pts',(-7.69917346821438,-20.4516474279977,
9.43555314181049));
#39315=CARTESIAN_POINT('Ctrl Pts',(-7.9249847794445,-20.4633176660218,9.24191898339155));
#39316=CARTESIAN_POINT('Ctrl Pts',(-8.14066853729478,-20.474464498208,9.05696924500836));
#39317=CARTESIAN_POINT('Ctrl Pts',(-8.34990739550198,-20.4856113303942,
8.86443818228698));
#39318=CARTESIAN_POINT('Ctrl Pts',(-8.55217478046388,-20.4967581625804,
8.66479986926402));
#39319=CARTESIAN_POINT('Ctrl Pts',(-8.75440768931906,-20.5079030948094,
8.46519558422725));
#39320=CARTESIAN_POINT('Ctrl Pts',(-8.9496713075049,-20.5190480270384,8.25848665482182));
#39321=CARTESIAN_POINT('Ctrl Pts',(-9.13747528589881,-20.5301929592674,
8.04518462495352));
#39322=CARTESIAN_POINT('Ctrl Pts',(-9.3252583249383,-20.5413366488833,7.83190637736524));
#39323=CARTESIAN_POINT('Ctrl Pts',(-9.5055832087329,-20.5524803384992,7.61203669738287));
#39324=CARTESIAN_POINT('Ctrl Pts',(-9.67799849801041,-20.5636240281151,
7.38612180528512));
#39325=CARTESIAN_POINT('Ctrl Pts',(-9.85585682286771,-20.5751195165727,
7.15307493086235));
#39326=CARTESIAN_POINT('Ctrl Pts',(-10.0252978522716,-20.5866150050304,
6.91359518794776));
#39327=CARTESIAN_POINT('Ctrl Pts',(-10.1858721211816,-20.598110493488,6.66831758248921));
#39328=CARTESIAN_POINT('Ctrl Pts',(-10.3415405228375,-20.6092547716255,
6.43053370177853));
#39329=CARTESIAN_POINT('Ctrl Pts',(-10.4888757631469,-20.620399049763,6.18730120579808));
#39330=CARTESIAN_POINT('Ctrl Pts',(-10.6275127035771,-20.6315433279005,
5.93922755796635));
#39331=CARTESIAN_POINT('Ctrl Pts',(-10.7727033288179,-20.6432144215182,
5.67942690221995));
#39332=CARTESIAN_POINT('Ctrl Pts',(-10.9083532859157,-20.654885515136,5.41431662760413));
#39333=CARTESIAN_POINT('Ctrl Pts',(-11.0340969861489,-20.6665566087537,
5.14462379093558));
#39334=CARTESIAN_POINT('Ctrl Pts',(-11.159840686382,-20.6782277023714,4.87493095426703));
#39335=CARTESIAN_POINT('Ctrl Pts',(-11.2756779958382,-20.6898987959892,
4.60065586355721));
#39336=CARTESIAN_POINT('Ctrl Pts',(-11.3813005554201,-20.7015698896069,
4.32255108902081));
#39337=CARTESIAN_POINT('Ctrl Pts',(-11.4819409370545,-20.7126904619584,
4.05756441614999));
#39338=CARTESIAN_POINT('Ctrl Pts',(-11.5733394354702,-20.7238110343099,
3.7890178396337));
#39339=CARTESIAN_POINT('Ctrl Pts',(-11.6552609185346,-20.7349316066614,
3.51757632054809));
#39340=CARTESIAN_POINT('Ctrl Pts',(-11.7411699266226,-20.7465934724425,
3.23292239600646));
#39341=CARTESIAN_POINT('Ctrl Pts',(-11.8166563253145,-20.7582553382236,
2.94508500430039));
#39342=CARTESIAN_POINT('Ctrl Pts',(-11.8815075908379,-20.7699172040048,
2.65484982981369));
#39343=CARTESIAN_POINT('Ctrl Pts',(-11.9433326930578,-20.7810348905784,
2.37815793821194));
#39344=CARTESIAN_POINT('Ctrl Pts',(-11.995492397791,-20.792152577152,2.09928720024168));
#39345=CARTESIAN_POINT('Ctrl Pts',(-12.0378545291329,-20.8032702637256,
1.81893061589332));
#39346=CARTESIAN_POINT('Ctrl Pts',(-12.0802138904517,-20.8143872233234,
1.53859236381978));
#39347=CARTESIAN_POINT('Ctrl Pts',(-12.1127769187808,-20.8255041829211,
1.25676872584638));
#39348=CARTESIAN_POINT('Ctrl Pts',(-12.1354629727721,-20.8366211425188,
0.974160503447343));
#39349=CARTESIAN_POINT('Ctrl Pts',(-12.1581504142312,-20.8477387820242,
0.691534996870884));
#39350=CARTESIAN_POINT('Ctrl Pts',(-12.1709596530285,-20.8588564215296,
0.408125078448854));
#39351=CARTESIAN_POINT('Ctrl Pts',(-12.1738620090751,-20.869974061035,0.124635604858819));
#39352=CARTESIAN_POINT('Ctrl Pts',(-12.1742883992265,-20.8716073727016,
0.0829876755153614));
#39353=CARTESIAN_POINT('Ctrl Pts',(-12.1745010602666,-20.8732406843683,
0.0413380318515849));
#39354=CARTESIAN_POINT('Ctrl Pts',(-12.1744999960254,-20.8748739960349,
-0.000311089488517879));
#39355=CARTESIAN_POINT('Ctrl Pts',(-12.1744999960254,-20.8748739960726,
-0.000311090449404772));
#39356=CARTESIAN_POINT('Ctrl Pts',(-12.1744923950652,-20.8865393020214,
-0.297774062673808));
#39357=CARTESIAN_POINT('Ctrl Pts',(-12.1635784601364,-20.8982046079702,
-0.595182841827181));
#39358=CARTESIAN_POINT('Ctrl Pts',(-12.1417960711354,-20.909869913919,-0.891761412577232));
#39359=CARTESIAN_POINT('Ctrl Pts',(-12.1231530265705,-20.9198539803433,
-1.14559617382575));
#39360=CARTESIAN_POINT('Ctrl Pts',(-12.0965494250141,-20.9298380467676,
-1.39882274221339));
#39361=CARTESIAN_POINT('Ctrl Pts',(-12.0620392196327,-20.939822113192,-1.65095733259334));
#39362=CARTESIAN_POINT('Ctrl Pts',(-12.0235090635879,-20.9509691820964,
-1.9324620354562));
#39363=CARTESIAN_POINT('Ctrl Pts',(-11.9751141751885,-20.9621162510008,
-2.2126594358091));
#39364=CARTESIAN_POINT('Ctrl Pts',(-11.9169675814257,-20.9732633199052,
-2.49085003829017));
#39365=CARTESIAN_POINT('Ctrl Pts',(-11.8588308783237,-20.9844084927074,
-2.76899332090735));
#39366=CARTESIAN_POINT('Ctrl Pts',(-11.7909458361135,-20.9955536655097,
-3.04513022613635));
#39367=CARTESIAN_POINT('Ctrl Pts',(-11.7134766039781,-21.006698838312,-3.31857139414821));
#39368=CARTESIAN_POINT('Ctrl Pts',(-11.6360159868468,-21.0178427717099,
-3.591982154));
#39369=CARTESIAN_POINT('Ctrl Pts',(-11.5489733807489,-21.0289867051078,
-3.86269751864585));
#39370=CARTESIAN_POINT('Ctrl Pts',(-11.4525631648402,-21.0401306385056,
-4.1300420343315));
#39371=CARTESIAN_POINT('Ctrl Pts',(-11.3531130779724,-21.0516259466949,
-4.40581608024554));
#39372=CARTESIAN_POINT('Ctrl Pts',(-11.2436951564039,-21.0631212548842,
-4.67800297633621));
#39373=CARTESIAN_POINT('Ctrl Pts',(-11.1245994311076,-21.0746165630735,
-4.94588088689978));
#39374=CARTESIAN_POINT('Ctrl Pts',(-11.0091379329855,-21.0857610898951,
-5.20558445552521));
#39375=CARTESIAN_POINT('Ctrl Pts',(-10.8845806273897,-21.0969056167168,
-5.46123786352323));
#39376=CARTESIAN_POINT('Ctrl Pts',(-10.7512401330826,-21.1080501435385,
-5.71220499026376));
#39377=CARTESIAN_POINT('Ctrl Pts',(-10.6116041681331,-21.1197208424116,
-5.97502115196405));
#39378=CARTESIAN_POINT('Ctrl Pts',(-10.4623358132792,-21.1313915412847,
-6.23269757967499));
#39379=CARTESIAN_POINT('Ctrl Pts',(-10.3038478790065,-21.1430622401578,
-6.48453307002857));
#39380=CARTESIAN_POINT('Ctrl Pts',(-10.1453599447337,-21.1547329390309,
-6.73636856038215));
#39381=CARTESIAN_POINT('Ctrl Pts',(-9.97765261724218,-21.166403637904,-6.98236283400452));
#39382=CARTESIAN_POINT('Ctrl Pts',(-9.80119115426147,-21.1780743367771,
-7.22184894660825));
#39383=CARTESIAN_POINT('Ctrl Pts',(-9.63264179299859,-21.1892217499704,
-7.45059708588386));
#39384=CARTESIAN_POINT('Ctrl Pts',(-9.45605571647231,-21.2003691631638,
-7.67347617436341));
#39385=CARTESIAN_POINT('Ctrl Pts',(-9.27186695090699,-21.2115165763572,
-7.88992607662954));
#39386=CARTESIAN_POINT('Ctrl Pts',(-9.08770945043724,-21.2226620973345,
-8.10633923763807));
#39387=CARTESIAN_POINT('Ctrl Pts',(-8.89595201024563,-21.2338076183118,
-8.31632518819218));
#39388=CARTESIAN_POINT('Ctrl Pts',(-8.69706869375794,-21.2449531392891,
-8.51935715802874));
#39389=CARTESIAN_POINT('Ctrl Pts',(-8.49820744079386,-21.2560974238155,
-8.72236660410243));
#39390=CARTESIAN_POINT('Ctrl Pts',(-8.29222207669095,-21.2672417083419,
-8.91842341943104));
#39391=CARTESIAN_POINT('Ctrl Pts',(-8.07962411441024,-21.2783859928682,
-9.10703708237979));
#39392=CARTESIAN_POINT('Ctrl Pts',(-7.86033469976557,-21.2898810401594,
-9.30158729959874));
#39393=CARTESIAN_POINT('Ctrl Pts',(-7.63400990204134,-21.3013760874505,
-9.48821803027954));
#39394=CARTESIAN_POINT('Ctrl Pts',(-7.40124976128749,-21.3128711347417,
-9.66643430749115));
#39395=CARTESIAN_POINT('Ctrl Pts',(-7.17558004674712,-21.3240160156153,
-9.83922169400216));
#39396=CARTESIAN_POINT('Ctrl Pts',(-6.94386147980823,-21.3351608964889,
-10.0040995187547));
#39397=CARTESIAN_POINT('Ctrl Pts',(-6.70667300845964,-21.3463057773625,
-10.1606588077545));
#39398=CARTESIAN_POINT('Ctrl Pts',(-6.45830602768054,-21.3579759078624,
-10.3245966151054));
#39399=CARTESIAN_POINT('Ctrl Pts',(-6.20394142385836,-21.3696460383624,
-10.4794127629059));
#39400=CARTESIAN_POINT('Ctrl Pts',(-5.94427710028753,-21.3813161688623,
-10.6246891721592));
#39401=CARTESIAN_POINT('Ctrl Pts',(-5.68461277671671,-21.3929862993622,
-10.7699655814125));
#39402=CARTESIAN_POINT('Ctrl Pts',(-5.41964903042489,-21.4046564298622,
-10.9057020959921));
#39403=CARTESIAN_POINT('Ctrl Pts',(-5.15011341352574,-21.4163265603621,
-11.031535798692));
#39404=CARTESIAN_POINT('Ctrl Pts',(-4.89265384818702,-21.4274738319566,
-11.1517317519199));
#39405=CARTESIAN_POINT('Ctrl Pts',(-4.63094619394671,-21.4386211035511,
-11.262928642111));
#39406=CARTESIAN_POINT('Ctrl Pts',(-4.36563958289154,-21.4497683751456,
-11.3648423342469));
#39407=CARTESIAN_POINT('Ctrl Pts',(-4.10037804211338,-21.460913753042,-11.4667387132886));
#39408=CARTESIAN_POINT('Ctrl Pts',(-3.83151901407759,-21.4720591309384,
-11.5593549471958));
#39409=CARTESIAN_POINT('Ctrl Pts',(-3.55973082007956,-21.4832045088348,
-11.6424553569501));
#39410=CARTESIAN_POINT('Ctrl Pts',(-3.28797280464175,-21.4943486491813,
-11.7255465394797));
#39411=CARTESIAN_POINT('Ctrl Pts',(-3.01328652773389,-21.5054927895278,
-11.7991239297607));
#39412=CARTESIAN_POINT('Ctrl Pts',(-2.73635584774457,-21.5166369298742,
-11.8630015984368));
#39413=CARTESIAN_POINT('Ctrl Pts',(-2.45070250392632,-21.5281320843803,
-11.9288912631476));
#39414=CARTESIAN_POINT('Ctrl Pts',(-2.16266136567062,-21.5396272388864,
-11.9844601901464));
#39415=CARTESIAN_POINT('Ctrl Pts',(-1.87299620102137,-21.5511223933925,
-12.0295609014195));
#39416=CARTESIAN_POINT('Ctrl Pts',(-1.59216120034856,-21.5622671291682,
-12.0732867608822));
#39417=CARTESIAN_POINT('Ctrl Pts',(-1.30979999634929,-21.573411864944,-12.1071731361329));
#39418=CARTESIAN_POINT('Ctrl Pts',(-1.02661663648201,-21.5845566007197,
-12.1311379734837));
#39419=CARTESIAN_POINT('Ctrl Pts',(-0.730077273105364,-21.596226964591,
-12.156233083644));
#39420=CARTESIAN_POINT('Ctrl Pts',(-0.432636652240616,-21.6078973284622,
-12.1704482314372));
#39421=CARTESIAN_POINT('Ctrl Pts',(-0.135107706832327,-21.6195676923335,
-12.1737502914079));
#39422=CARTESIAN_POINT('Ctrl Pts',(0.162421238575963,-21.6312380562048,
-12.1770523513786));
#39423=CARTESIAN_POINT('Ctrl Pts',(0.460038172932362,-21.642908420076,-12.1694413285824));
#39424=CARTESIAN_POINT('Ctrl Pts',(0.756930527455535,-21.6545787839473,
-12.1509467296423));
#39425=CARTESIAN_POINT('Ctrl Pts',(1.04051646831786,-21.665726093968,-12.1332810398346));
#39426=CARTESIAN_POINT('Ctrl Pts',(1.3235260540737,-21.6768734039887,-12.1056806331005));
#39427=CARTESIAN_POINT('Ctrl Pts',(1.60525332965216,-21.6880207140093,-12.06820666038));
#39428=CARTESIAN_POINT('Ctrl Pts',(1.88693275396258,-21.6991661306637,-12.0307390525992));
#39429=CARTESIAN_POINT('Ctrl Pts',(2.16733003861535,-21.7103115473181,-11.983401262163));
#39430=CARTESIAN_POINT('Ctrl Pts',(2.44574556760614,-21.7214569639726,-11.9263061703335));
#39431=CARTESIAN_POINT('Ctrl Pts',(2.72413018796538,-21.7326011433053,-11.8692174169836));
#39432=CARTESIAN_POINT('Ctrl Pts',(3.00053323073972,-21.743745322638,-11.8023735788288));
#39433=CARTESIAN_POINT('Ctrl Pts',(3.27426524481699,-21.7548895019707,-11.725938655672));
#39434=CARTESIAN_POINT('Ctrl Pts',(3.55661747114512,-21.7663846274341,-11.6470966875695));
#39435=CARTESIAN_POINT('Ctrl Pts',(3.83612742536457,-21.7778797528976,-11.5580498424949));
#39436=CARTESIAN_POINT('Ctrl Pts',(4.11205390419248,-21.7893748783611,-11.4590341189393));
#39437=CARTESIAN_POINT('Ctrl Pts',(4.37957064322365,-21.8005196532004,-11.3630362154728));
#39438=CARTESIAN_POINT('Ctrl Pts',(4.64371884535657,-21.8116644280397,-11.2576681964017));
#39439=CARTESIAN_POINT('Ctrl Pts',(4.90384104113911,-21.8228092028791,-11.1431949320309));
#39440=CARTESIAN_POINT('Ctrl Pts',(5.17622916085864,-21.8344795036546,-11.0233237416993));
#39441=CARTESIAN_POINT('Ctrl Pts',(5.4442021591021,-21.8461498044302,-10.8934680664644));
#39442=CARTESIAN_POINT('Ctrl Pts',(5.70703039091341,-21.8578201052057,-10.7539878355516));
#39443=CARTESIAN_POINT('Ctrl Pts',(5.96985862272471,-21.8694904059813,-10.6145076046387));
#39444=CARTESIAN_POINT('Ctrl Pts',(6.22754179586539,-21.8811607067569,-10.465402983073));
#39445=CARTESIAN_POINT('Ctrl Pts',(6.47938055605088,-21.8928310075324,-10.3070887189288));
#39446=CARTESIAN_POINT('Ctrl Pts',(6.71993112197717,-21.9039782092341,-10.1558705910837));
#39447=CARTESIAN_POINT('Ctrl Pts',(6.95522152552982,-21.9151254109358,-9.99620511839035));
#39448=CARTESIAN_POINT('Ctrl Pts',(7.18466117342611,-21.9262726126375,-9.82848381354232));
#39449=CARTESIAN_POINT('Ctrl Pts',(7.26134175173749,-21.9299980972295,-9.77243000257806));
#39450=CARTESIAN_POINT('Ctrl Pts',(7.33736906532864,-21.9337235818215,-9.71547675626813));
#39451=CARTESIAN_POINT('Ctrl Pts',(7.41272179941102,-21.9374490664136,-9.65763976210216));
#39452=CARTESIAN_POINT('Origin',(0.,-20.,0.));
#39453=CARTESIAN_POINT('',(10.3559140620128,-38.4202905549692,1.73955308634279));
#39454=CARTESIAN_POINT('',(10.355914065439,-39.2383818084129,1.73955306594595));
#39455=CARTESIAN_POINT('',(10.355914065439,-20.,1.73955306594593));
#39456=CARTESIAN_POINT('',(-1.99079507083261,-40.,10.3105642903746));
#39457=CARTESIAN_POINT('Ctrl Pts',(10.355914065439,-39.2383818084129,1.73955306594595));
#39458=CARTESIAN_POINT('Ctrl Pts',(10.3137968728013,-39.2499421539653,1.99028530066326));
#39459=CARTESIAN_POINT('Ctrl Pts',(10.2625736848822,-39.2615024995176,2.23946228145483));
#39460=CARTESIAN_POINT('Ctrl Pts',(10.2023884912638,-39.27306284507,2.48641711571641));
#39461=CARTESIAN_POINT('Ctrl Pts',(10.1812505764525,-39.2771230064615,2.57315124308255));
#39462=CARTESIAN_POINT('Ctrl Pts',(10.1590076417178,-39.2811831678531,2.65961136916614));
#39463=CARTESIAN_POINT('Ctrl Pts',(10.1356674049065,-39.2852433292447,2.74576897373338));
#39464=CARTESIAN_POINT('Ctrl Pts',(10.0690759979193,-39.296827267396,2.99158293685373));
#39465=CARTESIAN_POINT('Ctrl Pts',(9.99352834835741,-39.3084112055473,3.2350090451317));
#39466=CARTESIAN_POINT('Ctrl Pts',(9.90922078800109,-39.3199951436986,3.47539125490169));
#39467=CARTESIAN_POINT('Ctrl Pts',(9.82492758520526,-39.3315771091076,3.71573252762991));
#39468=CARTESIAN_POINT('Ctrl Pts',(9.73187754086394,-39.3431590745166,3.95303067716415));
#39469=CARTESIAN_POINT('Ctrl Pts',(9.63031632810827,-39.3547410399256,4.18664644083677));
#39470=CARTESIAN_POINT('Ctrl Pts',(9.52876641285088,-39.3663217169763,4.42023621748527));
#39471=CARTESIAN_POINT('Ctrl Pts',(9.41870732932391,-39.3779023940269,4.65014417391184));
#39472=CARTESIAN_POINT('Ctrl Pts',(9.30043265936412,-39.3894830710776,4.87575156756713));
#39473=CARTESIAN_POINT('Ctrl Pts',(9.18214987722267,-39.4010645424197,5.10137443510336));
#39474=CARTESIAN_POINT('Ctrl Pts',(9.05565050760297,-39.4126460137618,5.32269590522329));
#39475=CARTESIAN_POINT('Ctrl Pts',(8.92127444893441,-39.4242274851039,5.53912115834182));
#39476=CARTESIAN_POINT('Ctrl Pts',(8.78690188205367,-39.4358086554992,5.75554078760838));
#39477=CARTESIAN_POINT('Ctrl Pts',(8.64465318193135,-39.4473898258945,5.96706422131404));
#39478=CARTESIAN_POINT('Ctrl Pts',(8.49491242743426,-39.4589709962898,6.17312431838393));
#39479=CARTESIAN_POINT('Ctrl Pts',(8.34514009761779,-39.4705546087668,6.37922786663983));
#39480=CARTESIAN_POINT('Ctrl Pts',(8.18787271707229,-39.4821382212438,6.57986555252027));
#39481=CARTESIAN_POINT('Ctrl Pts',(8.02353650941463,-39.4937218337208,6.77450093232635));
#39482=CARTESIAN_POINT('Ctrl Pts',(7.88273702232455,-39.5036464067571,6.94126005398848));
#39483=CARTESIAN_POINT('Ctrl Pts',(7.73674929148784,-39.5135709797935,7.10361351542306));
#39484=CARTESIAN_POINT('Ctrl Pts',(7.58586439719135,-39.5234955528298,7.26124385676619));
#39485=CARTESIAN_POINT('Ctrl Pts',(7.41051234539617,-39.5350294724659,7.44443518223697));
#39486=CARTESIAN_POINT('Ctrl Pts',(7.22849149706608,-39.5465633921019,7.62130277938994));
#39487=CARTESIAN_POINT('Ctrl Pts',(7.04028338094605,-39.558097311738,7.79136771792828));
#39488=CARTESIAN_POINT('Ctrl Pts',(6.85210898568282,-39.5696291648657,7.96140218628521));
#39489=CARTESIAN_POINT('Ctrl Pts',(6.65774974306552,-39.5811610179933,8.12463624128184));
#39490=CARTESIAN_POINT('Ctrl Pts',(6.45772254452777,-39.592692871121,8.28062923562563));
#39491=CARTESIAN_POINT('Ctrl Pts',(6.2577168989946,-39.6042234816872,8.43660542166661));
#39492=CARTESIAN_POINT('Ctrl Pts',(6.05204473760968,-39.6157540922535,8.58534193270929));
#39493=CARTESIAN_POINT('Ctrl Pts',(5.84125523482977,-39.6272847028197,8.72643903786498));
#39494=CARTESIAN_POINT('Ctrl Pts',(5.63044338606736,-39.6388165357562,8.86755110085016));
#39495=CARTESIAN_POINT('Ctrl Pts',(5.41451334264833,-39.6503483686927,9.00102198096848));
#39496=CARTESIAN_POINT('Ctrl Pts',(5.19404353388615,-39.6618802016292,9.12649509768649));
#39497=CARTESIAN_POINT('Ctrl Pts',(4.97357359805668,-39.6734120412121,9.25196828672065));
#39498=CARTESIAN_POINT('Ctrl Pts',(4.74856413637869,-39.6849438807949,9.36944356696252));
#39499=CARTESIAN_POINT('Ctrl Pts',(4.51961908132821,-39.6964757203778,9.47860983265447));
#39500=CARTESIAN_POINT('Ctrl Pts',(4.2906085924439,-39.7080108558277,9.58780729870271));
#39501=CARTESIAN_POINT('Ctrl Pts',(4.05766051472073,-39.7195459912777,9.68869088273747));
#39502=CARTESIAN_POINT('Ctrl Pts',(3.82140107039531,-39.7310811267276,9.7809966189127));
#39503=CARTESIAN_POINT('Ctrl Pts',(3.61203246650753,-39.74130334329,9.86279619805342));
#39504=CARTESIAN_POINT('Ctrl Pts',(3.40006381849039,-39.7515255598525,9.93786007685317));
#39505=CARTESIAN_POINT('Ctrl Pts',(3.18594275547069,-39.7617477764149,10.0060366658764));
#39506=CARTESIAN_POINT('Ctrl Pts',(2.94219156771723,-39.7733845457893,10.0836475478562));
#39507=CARTESIAN_POINT('Ctrl Pts',(2.69557041193126,-39.7850213151637,10.1523578833729));
#39508=CARTESIAN_POINT('Ctrl Pts',(2.44674288382941,-39.7966580845381,10.2119758254919));
#39509=CARTESIAN_POINT('Ctrl Pts',(2.19796065802866,-39.8082927352867,10.2715829133858));
#39510=CARTESIAN_POINT('Ctrl Pts',(1.94697312436059,-39.8199273860353,10.3221008501457));
#39511=CARTESIAN_POINT('Ctrl Pts',(1.69445649222457,-39.8315620367839,10.3633883549715));
#39512=CARTESIAN_POINT('Ctrl Pts',(1.44197452343055,-39.8431950904262,10.4046701921987));
#39513=CARTESIAN_POINT('Ctrl Pts',(1.18796414163377,-39.8548281440686,10.4367240840553));
#39514=CARTESIAN_POINT('Ctrl Pts',(0.933110299572317,-39.866461197711,10.4594601279814));
#39515=CARTESIAN_POINT('Ctrl Pts',(0.678258384732152,-39.8780941633835,
10.482195999976));
#39516=CARTESIAN_POINT('Ctrl Pts',(0.422563290990595,-39.8897271290559,
10.4956141379029));
#39517=CARTESIAN_POINT('Ctrl Pts',(0.166714969412438,-39.9013600947284,
10.4996765244923));
#39518=CARTESIAN_POINT('Ctrl Pts',(-0.0891139888816756,-39.912992179987,
10.5037386036294));
#39519=CARTESIAN_POINT('Ctrl Pts',(-0.345095881899718,-39.9246242652456,
10.4984463426919));
#39520=CARTESIAN_POINT('Ctrl Pts',(-0.600539942610578,-39.9362563505041,
10.4838138469418));
#39521=CARTESIAN_POINT('Ctrl Pts',(-0.856008621241452,-39.9478895567821,
10.4691799410137));
#39522=CARTESIAN_POINT('Ctrl Pts',(-1.11093909430189,-39.9595227630601,
10.4452040152679));
#39523=CARTESIAN_POINT('Ctrl Pts',(-1.36464347042229,-39.971155969338,10.411952228023));
#39524=CARTESIAN_POINT('Ctrl Pts',(-1.57432647122329,-39.9807706462253,
10.3844701063579));
#39525=CARTESIAN_POINT('Ctrl Pts',(-1.7831719369394,-39.9903853231127,10.3506527957081));
#39526=CARTESIAN_POINT('Ctrl Pts',(-1.99079507083262,-40.,10.3105642903746));
#39527=CARTESIAN_POINT('',(-9.92805791774733,-40.,-3.42120840959077));
#39528=CARTESIAN_POINT('Origin',(0.,-40.,0.));
#39529=CARTESIAN_POINT('Ctrl Pts',(-9.92805791774733,-40.,-3.42120840959077));
#39530=CARTESIAN_POINT('Ctrl Pts',(-10.1111316554273,-39.974275356352,-2.88994388159232));
#39531=CARTESIAN_POINT('Ctrl Pts',(-10.2512699108423,-39.9482650884727,
-2.34483397106979));
#39532=CARTESIAN_POINT('Ctrl Pts',(-10.4258103297589,-39.9013712674295,
-1.33653471943939));
#39533=CARTESIAN_POINT('Ctrl Pts',(-10.4744594655408,-39.8804422906188,
-0.87724558207502));
#39534=CARTESIAN_POINT('Ctrl Pts',(-10.5012056208305,-39.8500482605621,
-0.20301881929045));
#39535=CARTESIAN_POINT('Ctrl Pts',(-10.5031627804929,-39.8404701108489,
0.0104120456919794));
#39536=CARTESIAN_POINT('Ctrl Pts',(-10.4917955435466,-39.8165343692672,
0.543764874022827));
#39537=CARTESIAN_POINT('Ctrl Pts',(-10.4703474461067,-39.8021969428684,
0.863292901457895));
#39538=CARTESIAN_POINT('Ctrl Pts',(-10.3665187504896,-39.7604692508409,
1.78037491566855));
#39539=CARTESIAN_POINT('Ctrl Pts',(-10.2472399091455,-39.7325893674282,
2.37244076548405));
#39540=CARTESIAN_POINT('Ctrl Pts',(-9.92787464628935,-39.6803008606321,
3.46310075736266));
#39541=CARTESIAN_POINT('Ctrl Pts',(-9.73909313925916,-39.6559657510241,
3.96306068770059));
#39542=CARTESIAN_POINT('Ctrl Pts',(-9.24174827762745,-39.6029350754466,
5.02710969464659));
#39543=CARTESIAN_POINT('Ctrl Pts',(-8.91779324410202,-39.5744790473274,
5.58163838000466));
#39544=CARTESIAN_POINT('Ctrl Pts',(-8.32975921606371,-39.5286586219976,
6.4049721887172));
#39545=CARTESIAN_POINT('Ctrl Pts',(-8.09836911571393,-39.5116161086541,
6.69514443400181));
#39546=CARTESIAN_POINT('Ctrl Pts',(-7.54702162497352,-39.473359561036,7.31605142355112));
#39547=CARTESIAN_POINT('Ctrl Pts',(-7.21969293083172,-39.4521939186461,
7.63925312036954));
#39548=CARTESIAN_POINT('Ctrl Pts',(-6.44208798764159,-39.4052526783258,
8.31228952144449));
#39549=CARTESIAN_POINT('Ctrl Pts',(-5.98238039401832,-39.3796778943089,
8.64903454742865));
#39550=CARTESIAN_POINT('Ctrl Pts',(-5.22609734299015,-39.3398554548815,
9.11375315455387));
#39551=CARTESIAN_POINT('Ctrl Pts',(-4.94708413805671,-39.3255793506384,
9.26816836557142));
#39552=CARTESIAN_POINT('Ctrl Pts',(-4.12321987217292,-39.2840130284288,
9.67630563918418));
#39553=CARTESIAN_POINT('Ctrl Pts',(-3.56308446885428,-39.2562352744204,
9.89627289381794));
#39554=CARTESIAN_POINT('Ctrl Pts',(-2.47387356679438,-39.2039578764649,
10.2194768411937));
#39555=CARTESIAN_POINT('Ctrl Pts',(-1.94959154804844,-39.1795354772728,
10.3323217948457));
#39556=CARTESIAN_POINT('Ctrl Pts',(-0.784081167148053,-39.1264227880154,
10.4912734210105));
#39557=CARTESIAN_POINT('Ctrl Pts',(-0.142594206303842,-39.0979698678402,
10.5195650321403));
#39558=CARTESIAN_POINT('Ctrl Pts',(0.875743842932602,-39.0517984256466,
10.4712702322068));
#39559=CARTESIAN_POINT('Ctrl Pts',(1.25277714357594,-39.0343907046705,10.4328788093865));
#39560=CARTESIAN_POINT('Ctrl Pts',(2.07834302600836,-38.9958879636132,10.3034122761422));
#39561=CARTESIAN_POINT('Ctrl Pts',(2.52469037367328,-38.9748444752928,10.2032231797783));
#39562=CARTESIAN_POINT('Ctrl Pts',(3.49511560285828,-38.9286845765588,9.91779724428442));
#39563=CARTESIAN_POINT('Ctrl Pts',(4.01391229306815,-38.9037481075462,9.71941672261518));
#39564=CARTESIAN_POINT('Ctrl Pts',(4.80712973622315,-38.8643327691386,9.34170587069367));
#39565=CARTESIAN_POINT('Ctrl Pts',(5.09303602013273,-38.8498249264354,9.18895778939308));
#39566=CARTESIAN_POINT('Ctrl Pts',(5.67977192444265,-38.8189616826282,8.83968135322782));
#39567=CARTESIAN_POINT('Ctrl Pts',(5.9785021257871,-38.8025202094301,8.64044397520996));
#39568=CARTESIAN_POINT('Ctrl Pts',(6.64744313636834,-38.7641356919823,8.142969347724));
#39569=CARTESIAN_POINT('Ctrl Pts',(7.00879760375971,-38.7422381579637,7.83410596090346));
#39570=CARTESIAN_POINT('Ctrl Pts',(7.81805924234976,-38.6904747292404,7.04143980606615));
#39571=CARTESIAN_POINT('Ctrl Pts',(8.24380081964105,-38.6609603045329,6.53786641116099));
#39572=CARTESIAN_POINT('Ctrl Pts',(8.78267329648197,-38.6186340103273,5.76343210837005));
#39573=CARTESIAN_POINT('Ctrl Pts',(8.93610319106947,-38.605826340659,5.52254980062014));
#39574=CARTESIAN_POINT('Ctrl Pts',(9.25387399812242,-38.5771868840938,4.97566542339877));
#39575=CARTESIAN_POINT('Ctrl Pts',(9.41323590069673,-38.5612587613568,4.66716255801877));
#39576=CARTESIAN_POINT('Ctrl Pts',(9.75105795401619,-38.5237102398987,3.92519125036772));
#39577=CARTESIAN_POINT('Ctrl Pts',(9.91636962789157,-38.5021257350487,3.486528524834));
#39578=CARTESIAN_POINT('Ctrl Pts',(10.1806866381941,-38.460399479918,2.61206653098461));
#39579=CARTESIAN_POINT('Ctrl Pts',(10.2822193710206,-38.4402881546397,2.17827260156447));
#39580=CARTESIAN_POINT('Ctrl Pts',(10.3559140620128,-38.4202905549692,1.73955308634279));
#39581=CARTESIAN_POINT('Origin',(0.,-20.,0.));
#39582=CARTESIAN_POINT('',(10.3559140316505,-35.4203776493892,1.73955326709568));
#39583=CARTESIAN_POINT('',(10.3560200556488,-36.2384037331188,1.73957079674365));
#39584=CARTESIAN_POINT('',(10.355914065439,-20.,1.73955306594593));
#39585=CARTESIAN_POINT('',(-10.5009999970343,-37.6589303301852,0.000249570010058437));
#39586=CARTESIAN_POINT('Ctrl Pts',(10.3560200556488,-36.2384037331188,1.73957079674365));
#39587=CARTESIAN_POINT('Ctrl Pts',(10.1265052529798,-36.301008037487,3.09711120286187));
#39588=CARTESIAN_POINT('Ctrl Pts',(8.99979051820545,-36.443029749717,6.07621426388429));
#39589=CARTESIAN_POINT('Ctrl Pts',(5.36308582307284,-36.6644688698086,9.54309573608895));
#39590=CARTESIAN_POINT('Ctrl Pts',(0.142355108328082,-36.9027210933937,
10.9459171808689));
#39591=CARTESIAN_POINT('Ctrl Pts',(-5.1130915350103,-37.1409733169788,9.67934169719463));
#39592=CARTESIAN_POINT('Ctrl Pts',(-9.12160202863017,-37.3792255405639,
6.05225196529256));
#39593=CARTESIAN_POINT('Ctrl Pts',(-10.414406757941,-37.5518778777297,2.35425632961265));
#39594=CARTESIAN_POINT('Ctrl Pts',(-10.5016202439438,-37.6451128070338,
0.304109569145099));
#39595=CARTESIAN_POINT('Ctrl Pts',(-10.5013147911428,-37.6589303284762,
0.000249615072858407));
#39596=CARTESIAN_POINT('Ctrl Pts',(-10.5009999970343,-37.6589303301852,
0.000249570010058437));
#39597=CARTESIAN_POINT('Ctrl Pts',(-10.501006017267,-37.6704495017968,-0.253059966089447));
#39598=CARTESIAN_POINT('Ctrl Pts',(-10.4918420359383,-37.6819686734084,
-0.506405209212665));
#39599=CARTESIAN_POINT('Ctrl Pts',(-10.473526383441,-37.69348784502,-0.759108750684794));
#39600=CARTESIAN_POINT('Ctrl Pts',(-10.4552132077971,-37.7050054588767,
-1.01177811867446));
#39601=CARTESIAN_POINT('Ctrl Pts',(-10.4277508520089,-37.7165230727333,
-1.26380567781993));
#39602=CARTESIAN_POINT('Ctrl Pts',(-10.3912096537856,-37.7280406865899,
-1.51451739213295));
#39603=CARTESIAN_POINT('Ctrl Pts',(-10.3546663419992,-37.7395589666317,
-1.76524360775025));
#39604=CARTESIAN_POINT('Ctrl Pts',(-10.3090431757426,-37.7510772466734,
-2.01465354761341));
#39605=CARTESIAN_POINT('Ctrl Pts',(-10.2544621246906,-37.7625955267152,
-2.26208035517882));
#39606=CARTESIAN_POINT('Ctrl Pts',(-10.1998819030225,-37.7741136317315,
-2.50950340298135));
#39607=CARTESIAN_POINT('Ctrl Pts',(-10.1363441312941,-37.7856317367478,
-2.75494310446557));
#39608=CARTESIAN_POINT('Ctrl Pts',(-10.0640216334083,-37.797149841764,-2.9977440788516));
#39609=CARTESIAN_POINT('Ctrl Pts',(-9.99168235613647,-37.8086706190709,
-3.24060138496548));
#39610=CARTESIAN_POINT('Ctrl Pts',(-9.91055435963564,-37.8201913963777,
-3.48081847072262));
#39611=CARTESIAN_POINT('Ctrl Pts',(-9.82086037821651,-37.8317121736846,
-3.71775502576181));
#39612=CARTESIAN_POINT('Ctrl Pts',(-9.75853086376023,-37.8397181117011,
-3.88240532000537));
#39613=CARTESIAN_POINT('Ctrl Pts',(-9.69206584041268,-37.8477240497176,
-4.04547175410928));
#39614=CARTESIAN_POINT('Ctrl Pts',(-9.62155384401236,-37.8557299877341,
-4.20674489680217));
#39615=CARTESIAN_POINT('Ctrl Pts',(-9.51967913321632,-37.8672968509874,
-4.43974999678158));
#39616=CARTESIAN_POINT('Ctrl Pts',(-9.40932061872502,-37.8788637142408,
-4.66908884410403));
#39617=CARTESIAN_POINT('Ctrl Pts',(-9.29076776060954,-37.8904305774941,
-4.89414297077828));
#39618=CARTESIAN_POINT('Ctrl Pts',(-9.17223566898868,-37.90199541462,-5.1191576754986));
#39619=CARTESIAN_POINT('Ctrl Pts',(-9.04551222811135,-37.9135602517458,
-5.33988891303472));
#39620=CARTESIAN_POINT('Ctrl Pts',(-8.91093325131977,-37.9251250888717,
-5.5557420377951));
#39621=CARTESIAN_POINT('Ctrl Pts',(-8.77636931441983,-37.9366886335676,
-5.77157103986051));
#39622=CARTESIAN_POINT('Ctrl Pts',(-8.63395174090438,-37.9482521782636,
-5.98252278281262));
#39623=CARTESIAN_POINT('Ctrl Pts',(-8.48406072464804,-37.9598157229595,
-6.18802994663767));
#39624=CARTESIAN_POINT('Ctrl Pts',(-8.33415787571558,-37.9713801805032,
-6.39355333358115));
#39625=CARTESIAN_POINT('Ctrl Pts',(-8.17678056561849,-37.9829446380469,
-6.59363105689501));
#39626=CARTESIAN_POINT('Ctrl Pts',(-8.01235129322131,-37.9945090955906,
-6.78772625803478));
#39627=CARTESIAN_POINT('Ctrl Pts',(-7.84792499971694,-38.0060733436261,
-6.98181794283716));
#39628=CARTESIAN_POINT('Ctrl Pts',(-7.6764471798126,-38.0176375916616,-7.16992711216603));
#39629=CARTESIAN_POINT('Ctrl Pts',(-7.49837995428331,-38.0292018396971,
-7.35155079294173));
#39630=CARTESIAN_POINT('Ctrl Pts',(-7.32027095783739,-38.0407688004679,
-7.53321707890549));
#39631=CARTESIAN_POINT('Ctrl Pts',(-7.13556965973494,-38.0523357612386,
-7.70839463730362));
#39632=CARTESIAN_POINT('Ctrl Pts',(-6.94477534909365,-38.0639027220094,
-7.87661706258602));
#39633=CARTESIAN_POINT('Ctrl Pts',(-6.77939063709508,-38.073929218446,-8.02243596705712));
#39634=CARTESIAN_POINT('Ctrl Pts',(-6.60942841200286,-38.0839557148826,
-8.16302942840194));
#39635=CARTESIAN_POINT('Ctrl Pts',(-6.43523447667231,-38.0939822113192,
-8.2981177522525));
#39636=CARTESIAN_POINT('Ctrl Pts',(-6.23426730180032,-38.1055497590579,
-8.45396886584565));
#39637=CARTESIAN_POINT('Ctrl Pts',(-6.02760467181233,-38.1171173067966,
-8.60254000476339));
#39638=CARTESIAN_POINT('Ctrl Pts',(-5.81579678690838,-38.1286848545354,
-8.74342660136094));
#39639=CARTESIAN_POINT('Ctrl Pts',(-5.6040259696663,-38.1402503778832,-8.88428854195134));
#39640=CARTESIAN_POINT('Ctrl Pts',(-5.38711192540109,-38.151815901231,-9.01746847168526));
#39641=CARTESIAN_POINT('Ctrl Pts',(-5.16563415427181,-38.1633814245789,
-9.14260492333671));
#39642=CARTESIAN_POINT('Ctrl Pts',(-4.94418113678743,-38.1749456552965,
-9.26772738900991));
#39643=CARTESIAN_POINT('Ctrl Pts',(-4.71816565177371,-38.1865098860141,
-9.38480803549227));
#39644=CARTESIAN_POINT('Ctrl Pts',(-4.48819309123835,-38.1980741167318,
-9.49353062752527));
#39645=CARTESIAN_POINT('Ctrl Pts',(-4.25820248152583,-38.209639255057,-9.60226175254725));
#39646=CARTESIAN_POINT('Ctrl Pts',(-4.0242544245351,-38.2212043933823,-9.70263339102094));
#39647=CARTESIAN_POINT('Ctrl Pts',(-3.78697688107134,-38.2327695317075,
-9.79437629980752));
#39648=CARTESIAN_POINT('Ctrl Pts',(-3.54970371597984,-38.2443344566267,
-9.88611751570483));
#39649=CARTESIAN_POINT('Ctrl Pts',(-3.30910144613982,-38.2558993815458,
-9.969230222245));
#39650=CARTESIAN_POINT('Ctrl Pts',(-3.06581660782314,-38.2674643064649,
-10.0434938904345));
#39651=CARTESIAN_POINT('Ctrl Pts',(-2.82247493856302,-38.2790319329318,
-10.1177749064964));
#39652=CARTESIAN_POINT('Ctrl Pts',(-2.57644971301954,-38.2905995593986,
-10.1832026711533));
#39653=CARTESIAN_POINT('Ctrl Pts',(-2.32840260480898,-38.3021671858654,
-10.2396065505428));
#39654=CARTESIAN_POINT('Ctrl Pts',(-2.11348977034709,-38.3121896022117,
-10.2884759676535));
#39655=CARTESIAN_POINT('Ctrl Pts',(-1.8970594779061,-38.322212018558,-10.3305720727984));
#39656=CARTESIAN_POINT('Ctrl Pts',(-1.67954864780435,-38.3322344349043,
-10.3658148420497));
#39657=CARTESIAN_POINT('Ctrl Pts',(-1.42852518973776,-38.3438010387753,
-10.406487583748));
#39658=CARTESIAN_POINT('Ctrl Pts',(-1.17598466307407,-38.3553676426462,
-10.4380439947674));
#39659=CARTESIAN_POINT('Ctrl Pts',(-0.922603674343791,-38.3669342465172,
-10.4603921274533));
#39660=CARTESIAN_POINT('Ctrl Pts',(-0.669267061252899,-38.3784988246819,
-10.4827363462202));
#39661=CARTESIAN_POINT('Ctrl Pts',(-0.415090555598662,-38.3900634028467,
-10.4958754816972));
#39662=CARTESIAN_POINT('Ctrl Pts',(-0.160755867377762,-38.4016279810114,
-10.4997694522834));
#39663=CARTESIAN_POINT('Ctrl Pts',(0.0935504220672181,-38.4131912678861,
-10.5036629880725));
#39664=CARTESIAN_POINT('Ctrl Pts',(0.348014582076939,-38.4247545547607,
-10.4983134159245));
#39665=CARTESIAN_POINT('Ctrl Pts',(0.601953812652019,-38.4363178416354,
-10.4837327611607));
#39666=CARTESIAN_POINT('Ctrl Pts',(0.855913169215033,-38.4478820449599,
-10.4691509508051));
#39667=CARTESIAN_POINT('Ctrl Pts',(1.10934723657866,-38.4594462482844,-10.4453366084573));
#39668=CARTESIAN_POINT('Ctrl Pts',(1.36157588496065,-38.4710104516089,-10.4123538217587));
#39669=CARTESIAN_POINT('Ctrl Pts',(1.61380001522755,-38.4825744477865,-10.3793716258734));
#39670=CARTESIAN_POINT('Ctrl Pts',(1.8648184953714,-38.494138443964,-10.3372213518512));
#39671=CARTESIAN_POINT('Ctrl Pts',(2.11395819808633,-38.5057024401416,-10.2860187505538));
#39672=CARTESIAN_POINT('Ctrl Pts',(2.36315646670326,-38.517269154697,-10.2348041129309));
#39673=CARTESIAN_POINT('Ctrl Pts',(2.61047480368251,-38.5288358692525,-10.1745329500001));
#39674=CARTESIAN_POINT('Ctrl Pts',(2.85525066777235,-38.5404025838079,-10.105372067578));
#39675=CARTESIAN_POINT('Ctrl Pts',(3.06746464147513,-38.5504306087018,-10.0454114757192));
#39676=CARTESIAN_POINT('Ctrl Pts',(3.2777676572117,-38.5604586335956,-9.97876982858072));
#39677=CARTESIAN_POINT('Ctrl Pts',(3.48573704249832,-38.5704866584894,-9.90558621539155));
#39678=CARTESIAN_POINT('Ctrl Pts',(3.7256265304417,-38.5820538310016,-9.82117004293616));
#39679=CARTESIAN_POINT('Ctrl Pts',(3.96248524580083,-38.5936210035138,-9.7280223607574));
#39680=CARTESIAN_POINT('Ctrl Pts',(4.19567502657272,-38.605188176026,-9.62638624154433));
#39681=CARTESIAN_POINT('Ctrl Pts',(4.42882392223932,-38.6167533204687,-9.52476794216635));
#39682=CARTESIAN_POINT('Ctrl Pts',(4.65830491383272,-38.6283184649115,-9.41466428731077));
#39683=CARTESIAN_POINT('Ctrl Pts',(4.88350017832237,-38.6398836093542,-9.29636633359107));
#39684=CARTESIAN_POINT('Ctrl Pts',(5.10867022262449,-38.6514474585872,-9.17808162835856));
#39685=CARTESIAN_POINT('Ctrl Pts',(5.32955525319949,-38.6630113078201,-9.0516045853062));
#39686=CARTESIAN_POINT('Ctrl Pts',(5.54556142486565,-38.6745751570531,-8.91727253609768));
#39687=CARTESIAN_POINT('Ctrl Pts',(5.76158452743253,-38.6861399126786,-8.78292995773359));
#39688=CARTESIAN_POINT('Ctrl Pts',(5.97272777009596,-38.6977046683041,-8.64073128630361));
#39689=CARTESIAN_POINT('Ctrl Pts',(6.17842456612679,-38.7092694239296,-8.4910582897941));
#39690=CARTESIAN_POINT('Ctrl Pts',(6.38411756461389,-38.7208339660483,-8.34138805652523));
#39691=CARTESIAN_POINT('Ctrl Pts',(6.58436409479135,-38.732398508167,-8.18424393853169));
#39692=CARTESIAN_POINT('Ctrl Pts',(6.77862844023465,-38.7439630502857,-8.02004971737968));
#39693=CARTESIAN_POINT('Ctrl Pts',(6.9729382103727,-38.7555302965331,-7.85581710280887));
#39694=CARTESIAN_POINT('Ctrl Pts',(7.16126278800572,-38.7670975427805,-7.68453126845112));
#39695=CARTESIAN_POINT('Ctrl Pts',(7.34310018304362,-38.7786647890279,-7.50665576017609));
#39696=CARTESIAN_POINT('Ctrl Pts',(7.50068867675949,-38.7886894867101,-7.35250081634749));
#39697=CARTESIAN_POINT('Ctrl Pts',(7.65340527614783,-38.7987141843923,-7.19339723453153));
#39698=CARTESIAN_POINT('Ctrl Pts',(7.80094570771884,-38.8087388820745,-7.02966905801567));
#39699=CARTESIAN_POINT('Ctrl Pts',(7.97121434138562,-38.8203078571622,-6.8407190013345));
#39700=CARTESIAN_POINT('Ctrl Pts',(8.13464093951674,-38.8318768322498,-6.64555079086006));
#39701=CARTESIAN_POINT('Ctrl Pts',(8.29078139631834,-38.8434458073375,-6.44468345525688));
#39702=CARTESIAN_POINT('Ctrl Pts',(8.44689466556722,-38.8550127680073,-6.24385109515837));
#39703=CARTESIAN_POINT('Ctrl Pts',(8.5957241564423,-38.8665797286772,-6.03732180924652));
#39704=CARTESIAN_POINT('Ctrl Pts',(8.73686658849581,-38.878146689347,-5.82564702113212));
#39705=CARTESIAN_POINT('Ctrl Pts',(8.87799331885999,-38.8897123632258,-5.61399578122867));
#39706=CARTESIAN_POINT('Ctrl Pts',(9.0114345444902,-38.9012780371045,-5.39720041215733));
#39707=CARTESIAN_POINT('Ctrl Pts',(9.1368301862523,-38.9128437109833,-5.17584149173725));
#39708=CARTESIAN_POINT('Ctrl Pts',(9.26223565280195,-38.9244102910362,-4.95446522777686));
#39709=CARTESIAN_POINT('Ctrl Pts',(9.37959413660443,-38.9359768710891,-4.72852493708071));
#39710=CARTESIAN_POINT('Ctrl Pts',(9.48859075957821,-38.947543451142,-4.49862716806439));
#39711=CARTESIAN_POINT('Ctrl Pts',(9.59758534383839,-38.9591098148492,-4.26873369914191));
#39712=CARTESIAN_POINT('Ctrl Pts',(9.69821826319968,-38.9706761785565,-4.03488315072507));
#39713=CARTESIAN_POINT('Ctrl Pts',(9.79022185148165,-38.9822425422638,-3.79770418789712));
#39714=CARTESIAN_POINT('Ctrl Pts',(9.88224680885504,-38.9938115924172,-3.56047013701188));
#39715=CARTESIAN_POINT('Ctrl Pts',(9.9656383284593,-39.0053806425706,-3.31990638438798));
#39716=CARTESIAN_POINT('Ctrl Pts',(10.040177387235,-39.0169496927239,-3.07666037008559));
#39717=CARTESIAN_POINT('Ctrl Pts',(10.1046960415995,-39.0269634970358,-2.86611430497433));
#39718=CARTESIAN_POINT('Ctrl Pts',(10.1625830940347,-39.0369773013477,-2.65355905600627));
#39719=CARTESIAN_POINT('Ctrl Pts',(10.2137267948667,-39.0469911056596,-2.43942328426641));
#39720=CARTESIAN_POINT('Ctrl Pts',(10.2727684666407,-39.0585513122495,-2.19221915659396));
#39721=CARTESIAN_POINT('Ctrl Pts',(10.3228406406017,-39.0701115188394,-1.94283118836035));
#39722=CARTESIAN_POINT('Ctrl Pts',(10.3638016850672,-39.0816717254294,-1.69192660378597));
#39723=CARTESIAN_POINT('Ctrl Pts',(10.4047552723966,-39.0932298274335,-1.44106769748098));
#39724=CARTESIAN_POINT('Ctrl Pts',(10.4366009969215,-39.1047879294375,-1.18869299974049));
#39725=CARTESIAN_POINT('Ctrl Pts',(10.459248571689,-39.1163460314416,-0.935478655887372));
#39726=CARTESIAN_POINT('Ctrl Pts',(10.4818951135829,-39.1279036063227,-0.682275860220792));
#39727=CARTESIAN_POINT('Ctrl Pts',(10.4953443160468,-39.1394611812037,-0.428233770982764));
#39728=CARTESIAN_POINT('Ctrl Pts',(10.4995577670001,-39.1510187560848,-0.17403361005399));
#39729=CARTESIAN_POINT('Ctrl Pts',(10.5037709145365,-39.1625754986876,0.080148245542318));
#39730=CARTESIAN_POINT('Ctrl Pts',(10.4987496354465,-39.1741322412905,0.334487872675474));
#39731=CARTESIAN_POINT('Ctrl Pts',(10.484507635958,-39.1856889838933,0.588303179948864));
#39732=CARTESIAN_POINT('Ctrl Pts',(10.4702642162973,-39.1972468789021,0.842143796971907));
#39733=CARTESIAN_POINT('Ctrl Pts',(10.4467982537258,-39.2088047739108,1.09545971255835));
#39734=CARTESIAN_POINT('Ctrl Pts',(10.4141754984657,-39.2203626689196,1.34757177439928));
#39735=CARTESIAN_POINT('Ctrl Pts',(10.3972221813537,-39.2263690487507,1.47858878072037));
#39736=CARTESIAN_POINT('Ctrl Pts',(10.3777967899006,-39.2323754285818,1.60928074572872));
#39737=CARTESIAN_POINT('Ctrl Pts',(10.355914065439,-39.2383818084129,1.73955306594595));
#39738=CARTESIAN_POINT('Ctrl Pts',(10.3559140620128,-38.4202905549692,1.73955308634279));
#39739=CARTESIAN_POINT('Ctrl Pts',(10.3901797572621,-38.4109923050301,1.53556241881902));
#39740=CARTESIAN_POINT('Ctrl Pts',(10.4184269277223,-38.4017146247187,1.33050703383214));
#39741=CARTESIAN_POINT('Ctrl Pts',(10.4708508938559,-38.3797544179074,0.843834465812173));
#39742=CARTESIAN_POINT('Ctrl Pts',(10.48975813854,-38.3670808333518,0.561912731734641));
#39743=CARTESIAN_POINT('Ctrl Pts',(10.5071834954046,-38.3374403158734,-0.0923601063283838));
#39744=CARTESIAN_POINT('Ctrl Pts',(10.4973145956709,-38.3203433791977,-0.464548735667981));
#39745=CARTESIAN_POINT('Ctrl Pts',(10.4311838802339,-38.2820461086368,-1.29316339726322));
#39746=CARTESIAN_POINT('Ctrl Pts',(10.3646647484045,-38.2608948484542,-1.74802854183711));
#39747=CARTESIAN_POINT('Ctrl Pts',(10.1494117631921,-38.2139371231176,-2.7540656563222));
#39748=CARTESIAN_POINT('Ctrl Pts',(9.98511715635084,-38.1883329299172,-3.30043803410304));
#39749=CARTESIAN_POINT('Ctrl Pts',(9.66125723547714,-38.1485061445656,-4.12702485845205));
#39750=CARTESIAN_POINT('Ctrl Pts',(9.53179053499893,-38.134255539071,-4.41782651024056));
#39751=CARTESIAN_POINT('Ctrl Pts',(9.22254818339391,-38.1030341661345,-5.03530683296236));
#39752=CARTESIAN_POINT('Ctrl Pts',(9.03818034631058,-38.0859550084952,-5.35919663522209));
#39753=CARTESIAN_POINT('Ctrl Pts',(8.58400673720119,-38.0472321860406,-6.06672692249711));
#39754=CARTESIAN_POINT('Ctrl Pts',(8.30492167449681,-38.0256431348001,-6.44349543122926));
#39755=CARTESIAN_POINT('Ctrl Pts',(7.5791323067497,-37.9744519958695,-7.29749083215433));
#39756=CARTESIAN_POINT('Ctrl Pts',(7.1112360631156,-37.9451973819484,-7.75415782841438));
#39757=CARTESIAN_POINT('Ctrl Pts',(6.38436993163142,-37.9032550207047,-8.3420988044031));
#39758=CARTESIAN_POINT('Ctrl Pts',(6.15767308116984,-37.8905801002946,-8.51080788101325));
#39759=CARTESIAN_POINT('Ctrl Pts',(5.61721526489458,-37.8609360383146,-8.88011059507597));
#39760=CARTESIAN_POINT('Ctrl Pts',(5.29904365851014,-37.8438368511782,-9.07356554315724));
#39761=CARTESIAN_POINT('Ctrl Pts',(4.56681816543273,-37.8055381882346,-9.46710216779307));
#39762=CARTESIAN_POINT('Ctrl Pts',(4.14852033770569,-37.7843878111762,-9.65772442316781));
#39763=CARTESIAN_POINT('Ctrl Pts',(3.18639661109217,-37.7374301037312,-10.0220923706011));
#39764=CARTESIAN_POINT('Ctrl Pts',(2.63816848148224,-37.71182509799,-10.1801544672134));
#39765=CARTESIAN_POINT('Ctrl Pts',(1.76798949562244,-37.6719984312672,-10.355984995539));
#39766=CARTESIAN_POINT('Ctrl Pts',(1.45345538753827,-37.6577487729046,-10.4047910044558));
#39767=CARTESIAN_POINT('Ctrl Pts',(0.539891428658019,-37.6162023955407,
-10.5043097723675));
#39768=CARTESIAN_POINT('Ctrl Pts',(-0.0618767836849815,-37.5884173526605,
-10.5179909215598));
#39769=CARTESIAN_POINT('Ctrl Pts',(-1.19571668625076,-37.5361427183569,
-10.4464254414296));
#39770=CARTESIAN_POINT('Ctrl Pts',(-1.72659960155281,-37.5117296979594,
-10.3719053329147));
#39771=CARTESIAN_POINT('Ctrl Pts',(-2.87514527786277,-37.4586378897675,
-10.1200203023151));
#39772=CARTESIAN_POINT('Ctrl Pts',(-3.48692410041871,-37.4301961809479,
-9.92585572806258));
#39773=CARTESIAN_POINT('Ctrl Pts',(-4.42628879678326,-37.3840315895262,
-9.53008277645777));
#39774=CARTESIAN_POINT('Ctrl Pts',(-4.76716988270606,-37.3666188462688,
-9.36421832320812));
#39775=CARTESIAN_POINT('Ctrl Pts',(-5.49783622126238,-37.3281103637103,
-8.95843881850812));
#39776=CARTESIAN_POINT('Ctrl Pts',(-5.88243714631961,-37.3070662058718,
-8.71072745963657));
#39777=CARTESIAN_POINT('Ctrl Pts',(-6.6956376647593,-37.2608882563748,-8.10847682085518));
#39778=CARTESIAN_POINT('Ctrl Pts',(-7.11471826927713,-37.2359349976971,
-7.74336891273555));
#39779=CARTESIAN_POINT('Ctrl Pts',(-7.72945554692772,-37.1965151316267,
-7.11556738192073));
#39780=CARTESIAN_POINT('Ctrl Pts',(-7.94510908897947,-37.1820197022894,
-6.87393774098279));
#39781=CARTESIAN_POINT('Ctrl Pts',(-8.37604325490965,-37.1511351788362,
-6.34367471658154));
#39782=CARTESIAN_POINT('Ctrl Pts',(-8.5883401321292,-37.1346588352614,-6.05315681473701));
#39783=CARTESIAN_POINT('Ctrl Pts',(-9.04519498908136,-37.0962573772053,
-5.35542040341359));
#39784=CARTESIAN_POINT('Ctrl Pts',(-9.27788650950018,-37.0743783528394,
-4.94134718687087));
#39785=CARTESIAN_POINT('Ctrl Pts',(-9.76438598141428,-37.0226517828781,
-3.91920603860562));
#39786=CARTESIAN_POINT('Ctrl Pts',(-9.99059659457535,-36.9931553545202,
-3.30021415839559));
#39787=CARTESIAN_POINT('Ctrl Pts',(-10.2298337347066,-36.9508509584716,
-2.3880845333065));
#39788=CARTESIAN_POINT('Ctrl Pts',(-10.2909528004217,-36.9380474976631,
-2.1092020007096));
#39789=CARTESIAN_POINT('Ctrl Pts',(-10.4009929830534,-36.9094277615045,
-1.48678774644738));
#39790=CARTESIAN_POINT('Ctrl Pts',(-10.4444045131096,-36.8935155138551,
-1.14262562704172));
#39791=CARTESIAN_POINT('Ctrl Pts',(-10.5062602940058,-36.8559775006701,
-0.329943163467894));
#39792=CARTESIAN_POINT('Ctrl Pts',(-10.5105221300925,-36.834387397892,0.138933740486254));
#39793=CARTESIAN_POINT('Ctrl Pts',(-10.4457864132672,-36.7831944355856,
1.25784986902689));
#39794=CARTESIAN_POINT('Ctrl Pts',(-10.3474877776306,-36.7539390575865,
1.90424782655247));
#39795=CARTESIAN_POINT('Ctrl Pts',(-10.1215866452411,-36.7119955421712,
2.81145531001605));
#39796=CARTESIAN_POINT('Ctrl Pts',(-10.042298693671,-36.6993202048601,3.08269862297014));
#39797=CARTESIAN_POINT('Ctrl Pts',(-9.83344905793512,-36.6696760554708,
3.70307247067268));
#39798=CARTESIAN_POINT('Ctrl Pts',(-9.69606756687218,-36.6525772137359,
4.04916333147445));
#39799=CARTESIAN_POINT('Ctrl Pts',(-9.34876826955589,-36.6142787224382,
4.80441326606464));
#39800=CARTESIAN_POINT('Ctrl Pts',(-9.12976287408725,-36.5931281699535,
5.20857900645486));
#39801=CARTESIAN_POINT('Ctrl Pts',(-8.58141072505961,-36.546171337583,6.07904782579627));
#39802=CARTESIAN_POINT('Ctrl Pts',(-8.23910469668343,-36.5205673396163,
6.53548815025067));
#39803=CARTESIAN_POINT('Ctrl Pts',(-7.65053971510121,-36.4807408661328,
7.20010181020881));
#39804=CARTESIAN_POINT('Ctrl Pts',(-7.42889621411317,-36.4664903803013,
7.42857465298755));
#39805=CARTESIAN_POINT('Ctrl Pts',(-6.75982720062115,-36.4249506467354,
8.05832144825503));
#39806=CARTESIAN_POINT('Ctrl Pts',(-6.28792466078623,-36.3971733939983,
8.43171198698677));
#39807=CARTESIAN_POINT('Ctrl Pts',(-5.33995959978761,-36.3449021903794,
9.05772967191153));
#39808=CARTESIAN_POINT('Ctrl Pts',(-4.87128559642516,-36.3204850678521,
9.3181669606982));
#39809=CARTESIAN_POINT('Ctrl Pts',(-3.80269483284357,-36.2673849985505,
9.80922536149846));
#39810=CARTESIAN_POINT('Ctrl Pts',(-3.19735136539581,-36.2389392339463,
10.0228895411061));
#39811=CARTESIAN_POINT('Ctrl Pts',(-2.20908252818157,-36.1927704963497,
10.2729968211003));
#39812=CARTESIAN_POINT('Ctrl Pts',(-1.83708616009955,-36.1753578108648,
10.345994732251));
#39813=CARTESIAN_POINT('Ctrl Pts',(-1.00944489913079,-36.1368493503702,
10.4623539838356));
#39814=CARTESIAN_POINT('Ctrl Pts',(-0.553240485444117,-36.1158051563287,
10.4963691497786));
#39815=CARTESIAN_POINT('Ctrl Pts',(0.45864787437623,-36.0696271333995,10.505646249391));
#39816=CARTESIAN_POINT('Ctrl Pts',(1.01310200751067,-36.0446738379394,10.4667379536435));
#39817=CARTESIAN_POINT('Ctrl Pts',(1.88198526065261,-36.0052539457356,10.3360492225335));
#39818=CARTESIAN_POINT('Ctrl Pts',(2.19968348208914,-35.9907585271613,10.2731285845492));
#39819=CARTESIAN_POINT('Ctrl Pts',(2.8631048523538,-35.9598738800818,10.1095470843209));
#39820=CARTESIAN_POINT('Ctrl Pts',(3.20758192647379,-35.9433973981256,10.0055841389362));
#39821=CARTESIAN_POINT('Ctrl Pts',(3.99259124586388,-35.9049958727585,9.72395463586053));
#39822=CARTESIAN_POINT('Ctrl Pts',(4.42778265998368,-35.8831169218686,9.53366820008739));
#39823=CARTESIAN_POINT('Ctrl Pts',(5.43189959854408,-35.8313904989882,9.01098630818926));
#39824=CARTESIAN_POINT('Ctrl Pts',(5.98538066855198,-35.8018941428165,8.65324505530073));
#39825=CARTESIAN_POINT('Ctrl Pts',(6.72587203654103,-35.7595898261739,8.06939224653938));
#39826=CARTESIAN_POINT('Ctrl Pts',(6.94267731440192,-35.7467863732648,7.88363331407993));
#39827=CARTESIAN_POINT('Ctrl Pts',(7.40550657974443,-35.7181664382889,7.45316498574046));
#39828=CARTESIAN_POINT('Ctrl Pts',(7.64751271967655,-35.702253978042,7.20463262975789));
#39829=CARTESIAN_POINT('Ctrl Pts',(8.18651819305307,-35.6647158186083,6.59327584552595));
#39830=CARTESIAN_POINT('Ctrl Pts',(8.47241349625441,-35.6431257851068,6.22162247519114));
#39831=CARTESIAN_POINT('Ctrl Pts',(9.09488367700752,-35.5919329236896,5.28958695475419));
#39832=CARTESIAN_POINT('Ctrl Pts',(9.40587874698015,-35.5626775776679,4.71445725990754));
#39833=CARTESIAN_POINT('Ctrl Pts',(9.77216655635944,-35.5207341467763,3.85429075895417));
#39834=CARTESIAN_POINT('Ctrl Pts',(9.87230658321486,-35.5080588653303,3.59003563526119));
#39835=CARTESIAN_POINT('Ctrl Pts',(10.0793929160753,-35.4784142164439,2.96905938871876));
#39836=CARTESIAN_POINT('Ctrl Pts',(10.1782653227449,-35.46131480269,2.61005250471027));
#39837=CARTESIAN_POINT('Ctrl Pts',(10.294712872304,-35.4362376597028,2.07835083893602));
#39838=CARTESIAN_POINT('Ctrl Pts',(10.327401447064,-35.4283013538438,1.90929447616562));
#39839=CARTESIAN_POINT('Ctrl Pts',(10.3559140316505,-35.4203776493892,1.73955326709568));
#39840=CARTESIAN_POINT('Origin',(0.,-20.,0.));
#39841=CARTESIAN_POINT('',(10.3559140635165,-32.4208472785242,1.73955307739134));
#39842=CARTESIAN_POINT('',(10.3559140834541,-33.2387841926166,1.73955295869885));
#39843=CARTESIAN_POINT('',(10.355914065439,-20.,1.73955306594593));
#39844=CARTESIAN_POINT('',(-10.500269380848,-34.6589705026193,-0.000127306663085271));
#39845=CARTESIAN_POINT('Ctrl Pts',(10.3559140834541,-33.2387841926166,1.73955295869885));
#39846=CARTESIAN_POINT('Ctrl Pts',(10.2973924631457,-33.2547151709991,2.08794411799455));
#39847=CARTESIAN_POINT('Ctrl Pts',(10.2213159167763,-33.2705378423875,2.43322854355677));
#39848=CARTESIAN_POINT('Ctrl Pts',(10.0296902369874,-33.3030904856052,3.13283812117875));
#39849=CARTESIAN_POINT('Ctrl Pts',(9.91243744699974,-33.3198119228177,3.48610686019093));
#39850=CARTESIAN_POINT('Ctrl Pts',(9.67358767019652,-33.3497085214299,4.09542518246441));
#39851=CARTESIAN_POINT('Ctrl Pts',(9.55991772275114,-33.3627182664138,4.35416770444813));
#39852=CARTESIAN_POINT('Ctrl Pts',(9.14963705242817,-33.4058031174883,5.19431141293116));
#39853=CARTESIAN_POINT('Ctrl Pts',(8.80928925113612,-33.4357290612841,5.75266827127988));
#39854=CARTESIAN_POINT('Ctrl Pts',(8.13937141192271,-33.4864346431677,6.65139524394489));
#39855=CARTESIAN_POINT('Ctrl Pts',(7.83460309708945,-33.5073853499531,7.00781165521474));
#39856=CARTESIAN_POINT('Ctrl Pts',(7.26791133697995,-33.5437698631007,7.58718900440697));
#39857=CARTESIAN_POINT('Ctrl Pts',(7.01697012116098,-33.559164073229,7.81985289790815));
#39858=CARTESIAN_POINT('Ctrl Pts',(6.54052725549038,-33.5875875969846,8.22016201556931));
#39859=CARTESIAN_POINT('Ctrl Pts',(6.3188026777928,-33.6004940022986,8.39179900171593));
#39860=CARTESIAN_POINT('Ctrl Pts',(5.55946885917057,-33.6434471797072,8.93242487697804));
#39861=CARTESIAN_POINT('Ctrl Pts',(4.99439341476788,-33.6733510363649,9.26023662951819));
#39862=CARTESIAN_POINT('Ctrl Pts',(3.97960705825934,-33.7239224104242,9.72886321093979));
#39863=CARTESIAN_POINT('Ctrl Pts',(3.54411172102808,-33.7447639699962,9.89582378205501));
#39864=CARTESIAN_POINT('Ctrl Pts',(2.7605913941199,-33.7815751124668,10.1378281231161));
#39865=CARTESIAN_POINT('Ctrl Pts',(2.41715301412927,-33.7975121448548,10.2251548548626));
#39866=CARTESIAN_POINT('Ctrl Pts',(1.44212485624575,-33.8429520293784,10.4211987459417));
#39867=CARTESIAN_POINT('Ctrl Pts',(0.804060321109531,-33.872630919863,10.489738223794));
#39868=CARTESIAN_POINT('Ctrl Pts',(-0.374906274071377,-33.9265817583329,
10.5081229569328));
#39869=CARTESIAN_POINT('Ctrl Pts',(-0.9133998943455,-33.9509036209578,10.4750619973005));
#39870=CARTESIAN_POINT('Ctrl Pts',(-2.02696949219551,-34.0013955259621,
10.3201400141025));
#39871=CARTESIAN_POINT('Ctrl Pts',(-2.59917281747731,-34.0274921551402,
10.1910837431792));
#39872=CARTESIAN_POINT('Ctrl Pts',(-3.45010919296377,-34.0682987209603,
9.92279147991276));
#39873=CARTESIAN_POINT('Ctrl Pts',(-3.7383994157272,-34.0824360279519,9.81781093406341));
#39874=CARTESIAN_POINT('Ctrl Pts',(-4.57485464171308,-34.1241623004757,
9.47102458040724));
#39875=CARTESIAN_POINT('Ctrl Pts',(-5.10741188418669,-34.1515996155695,
9.1947798699861));
#39876=CARTESIAN_POINT('Ctrl Pts',(-6.00522751287061,-34.1996724107393,
8.62688039775064));
#39877=CARTESIAN_POINT('Ctrl Pts',(-6.38010065476171,-34.2204111088318,
8.35345098065261));
#39878=CARTESIAN_POINT('Ctrl Pts',(-7.01202317295036,-34.2573823172053,
7.82510558741575));
#39879=CARTESIAN_POINT('Ctrl Pts',(-7.27628399454426,-34.2735856944686,
7.58000225246598));
#39880=CARTESIAN_POINT('Ctrl Pts',(-7.97398417276742,-34.3193013815474,
6.86270757933141));
#39881=CARTESIAN_POINT('Ctrl Pts',(-8.37760370138294,-34.34898349091,6.36372128408552));
#39882=CARTESIAN_POINT('Ctrl Pts',(-9.0317606425054,-34.4028879542649,5.38398572717683));
#39883=CARTESIAN_POINT('Ctrl Pts',(-9.29550818257294,-34.4271617497354,
4.91462619281569));
#39884=CARTESIAN_POINT('Ctrl Pts',(-9.77180125519483,-34.4779006412457,
3.89018436110101));
#39885=CARTESIAN_POINT('Ctrl Pts',(-9.97557337595318,-34.5042885065916,
3.33310095202253));
#39886=CARTESIAN_POINT('Ctrl Pts',(-10.3766738294454,-34.5740556996699,
1.8617215613258));
#39887=CARTESIAN_POINT('Ctrl Pts',(-10.5010096203886,-34.6172210591878,
0.932883464836268));
#39888=CARTESIAN_POINT('Ctrl Pts',(-10.5009999994417,-34.6593914973464,
-0.000108285591527979));
#39889=CARTESIAN_POINT('Ctrl Pts',(-10.5001996603171,-34.6589303284762,
-0.000129121781424066));
#39890=CARTESIAN_POINT('Ctrl Pts',(-10.5005152891847,-34.6921039126934,
-0.729869341253787));
#39891=CARTESIAN_POINT('Ctrl Pts',(-10.2460312877903,-34.8046949047723,
-3.20638726464124));
#39892=CARTESIAN_POINT('Ctrl Pts',(-8.31997857721865,-34.9967033047129,
-7.11416351656478));
#39893=CARTESIAN_POINT('Ctrl Pts',(-3.90104496745925,-35.234955528298,-10.2281579100833));
#39894=CARTESIAN_POINT('Ctrl Pts',(1.46924208544258,-35.4732077518831,-10.847796722189));
#39895=CARTESIAN_POINT('Ctrl Pts',(6.48122296440533,-35.7114599754682,-8.82196775299734));
#39896=CARTESIAN_POINT('Ctrl Pts',(9.91261866563249,-35.9497121990533,-4.64471280984987));
#39897=CARTESIAN_POINT('Ctrl Pts',(10.6601686118332,-36.1253601182702,-0.730017845395118));
#39898=CARTESIAN_POINT('Ctrl Pts',(10.4176588865487,-36.2215906296253,1.37498776088105));
#39899=CARTESIAN_POINT('Ctrl Pts',(10.3560200556488,-36.2384037331188,1.73957079674365));
#39900=CARTESIAN_POINT('Ctrl Pts',(10.3559140316505,-35.4203776493892,1.73955326709568));
#39901=CARTESIAN_POINT('Ctrl Pts',(10.4034304843784,-35.4071727318551,1.45667816988187));
#39902=CARTESIAN_POINT('Ctrl Pts',(10.4393491507733,-35.3940054952443,1.1719009550135));
#39903=CARTESIAN_POINT('Ctrl Pts',(10.5116180404197,-35.3549077588437,0.318352847184844));
#39904=CARTESIAN_POINT('Ctrl Pts',(10.5134139691215,-35.3293026198815,-0.252206546139801));
#39905=CARTESIAN_POINT('Ctrl Pts',(10.4440818854216,-35.2894759087867,-1.13726178195156));
#39906=CARTESIAN_POINT('Ctrl Pts',(10.4048365005968,-35.2752263409407,-1.45312921361135));
#39907=CARTESIAN_POINT('Ctrl Pts',(10.2502270180083,-35.233680194394,-2.3589931954694));
#39908=CARTESIAN_POINT('Ctrl Pts',(10.0984985832242,-35.2058952957441,-2.9414765672684));
#39909=CARTESIAN_POINT('Ctrl Pts',(9.7189969494072,-35.1536207816812,-4.01231125877075));
#39910=CARTESIAN_POINT('Ctrl Pts',(9.50186491486644,-35.1292077395162,-4.50245821762584));
#39911=CARTESIAN_POINT('Ctrl Pts',(8.94491295605328,-35.0761157967444,-5.53803274620426));
#39912=CARTESIAN_POINT('Ctrl Pts',(8.59054820514668,-35.0476739799937,-6.07319819802585));
#39913=CARTESIAN_POINT('Ctrl Pts',(7.95252901874559,-35.0015091557408,-6.86817256939595));
#39914=CARTESIAN_POINT('Ctrl Pts',(7.69960773783804,-34.9840962893052,-7.15056194832371));
#39915=CARTESIAN_POINT('Ctrl Pts',(7.10915040816292,-34.9455877054709,-7.74208042091357));
#39916=CARTESIAN_POINT('Ctrl Pts',(6.76553720762311,-34.9245435703629,-8.04408761375559));
#39917=CARTESIAN_POINT('Ctrl Pts',(5.96350937284006,-34.878365307719,-8.66115028556577));
#39918=CARTESIAN_POINT('Ctrl Pts',(5.49753811294207,-34.8534117254717,-8.96415423137284));
#39919=CARTESIAN_POINT('Ctrl Pts',(4.72532047071464,-34.8139917942495,-9.38334294513234));
#39920=CARTESIAN_POINT('Ctrl Pts',(4.43385347036161,-34.7994966265131,-9.52453243285095));
#39921=CARTESIAN_POINT('Ctrl Pts',(3.80579782369832,-34.7686116746212,-9.7936828310673));
#39922=CARTESIAN_POINT('Ctrl Pts',(3.46821353185075,-34.7521346167262,-9.91825586971638));
#39923=CARTESIAN_POINT('Ctrl Pts',(2.67199181621678,-34.7137327959388,-10.1664414903612));
#39924=CARTESIAN_POINT('Ctrl Pts',(2.21001433240182,-34.6918541348475,-10.2767660044488));
#39925=CARTESIAN_POINT('Ctrl Pts',(1.09370362756925,-34.6401282866476,-10.4645693604838));
#39926=CARTESIAN_POINT('Ctrl Pts',(0.436426405672702,-34.6106322098475,
-10.5125142452268));
#39927=CARTESIAN_POINT('Ctrl Pts',(-0.506336637879259,-34.5683282613747,
-10.4926673374378));
#39928=CARTESIAN_POINT('Ctrl Pts',(-0.791290451375485,-34.5555249039931,
-10.4750322533597));
#39929=CARTESIAN_POINT('Ctrl Pts',(-1.42001494035827,-34.5269060974491,
-10.4103188109693));
#39930=CARTESIAN_POINT('Ctrl Pts',(-1.76288243823466,-34.5109946972992,
-10.3577706002858));
#39931=CARTESIAN_POINT('Ctrl Pts',(-2.56139976309308,-34.4734572615843,
-10.1945870267306));
#39932=CARTESIAN_POINT('Ctrl Pts',(-3.01350602193879,-34.4518668767639,
-10.0702117665141));
#39933=CARTESIAN_POINT('Ctrl Pts',(-4.07187183734195,-34.4006734594418,
-9.70136611575844));
#39934=CARTESIAN_POINT('Ctrl Pts',(-4.66660095032496,-34.3714179089478,
-9.42971385312827));
#39935=CARTESIAN_POINT('Ctrl Pts',(-5.47719771372925,-34.3294740674089,
-8.96387775873138));
#39936=CARTESIAN_POINT('Ctrl Pts',(-5.71633828839724,-34.3167985665749,
-8.81330088655491));
#39937=CARTESIAN_POINT('Ctrl Pts',(-6.25572641135615,-34.2871554022145,
-8.44247205014709));
#39938=CARTESIAN_POINT('Ctrl Pts',(-6.55090970155185,-34.2700577442309,
-8.21553486900428));
#39939=CARTESIAN_POINT('Ctrl Pts',(-7.18208544873548,-34.2317600323225,
-7.67460171699667));
#39940=CARTESIAN_POINT('Ctrl Pts',(-7.5107832298162,-34.2106090653874,-7.35323116707836));
#39941=CARTESIAN_POINT('Ctrl Pts',(-8.19765991623217,-34.1636543634845,
-6.58739254236621));
#39942=CARTESIAN_POINT('Ctrl Pts',(-8.54281049591999,-34.1380528074637,
-6.13317018380521));
#39943=CARTESIAN_POINT('Ctrl Pts',(-9.02072917736931,-34.0982268464365,
-5.38504385855398));
#39944=CARTESIAN_POINT('Ctrl Pts',(-9.17975325764311,-34.0839744000038,
-5.1092444357065));
#39945=CARTESIAN_POINT('Ctrl Pts',(-9.60193117811469,-34.0424492306008,
-4.29351694970631));
#39946=CARTESIAN_POINT('Ctrl Pts',(-9.8316221518757,-34.014689211405,-3.73771738646204));
#39947=CARTESIAN_POINT('Ctrl Pts',(-10.1740057745545,-33.9624254866379,
-2.6547031755924));
#39948=CARTESIAN_POINT('Ctrl Pts',(-10.296146051545,-33.9379991811499,-2.13242643317201));
#39949=CARTESIAN_POINT('Ctrl Pts',(-10.4757628900599,-33.8848742327228,
-0.969654362529974));
#39950=CARTESIAN_POINT('Ctrl Pts',(-10.5154101758528,-33.8564132653698,
-0.328583048387017));
#39951=CARTESIAN_POINT('Ctrl Pts',(-10.4850561816332,-33.8101568923869,
0.692317100695039));
#39952=CARTESIAN_POINT('Ctrl Pts',(-10.4530984977893,-33.792670546092,1.071644069824));
#39953=CARTESIAN_POINT('Ctrl Pts',(-10.3376718048425,-33.754111913925,1.90050423182263));
#39954=CARTESIAN_POINT('Ctrl Pts',(-10.245295955518,-33.7330917338209,2.3480408756075));
#39955=CARTESIAN_POINT('Ctrl Pts',(-9.97603185027046,-33.6868155929063,
3.32577058738486));
#39956=CARTESIAN_POINT('Ctrl Pts',(-9.78538152204616,-33.6617450340211,
3.85075162473856));
#39957=CARTESIAN_POINT('Ctrl Pts',(-9.42056376507948,-33.622308830007,4.65051258649645));
#39958=CARTESIAN_POINT('Ctrl Pts',(-9.27383127641737,-33.6079156844688,
4.93663232644258));
#39959=CARTESIAN_POINT('Ctrl Pts',(-8.93286593476369,-33.57688328798,5.53246954001651));
#39960=CARTESIAN_POINT('Ctrl Pts',(-8.7351223270134,-33.56014779091,5.83968615944232));
#39961=CARTESIAN_POINT('Ctrl Pts',(-8.24611489485502,-33.5216091080782,
6.51883189001247));
#39962=CARTESIAN_POINT('Ctrl Pts',(-7.94494948766482,-33.4998559812311,
6.88268608859146));
#39963=CARTESIAN_POINT('Ctrl Pts',(-7.16964126349981,-33.4483743654112,
7.70041144061197));
#39964=CARTESIAN_POINT('Ctrl Pts',(-6.67544960018752,-33.4189948270847,
8.13255731919555));
#39965=CARTESIAN_POINT('Ctrl Pts',(-5.91363380191436,-33.376850463152,8.68221075323397));
#39966=CARTESIAN_POINT('Ctrl Pts',(-5.67638980168292,-33.3640932965017,
8.83914270618776));
#39967=CARTESIAN_POINT('Ctrl Pts',(-5.12453884880811,-33.33489203208,9.17279090510368));
#39968=CARTESIAN_POINT('Ctrl Pts',(-4.80661127922917,-33.3183338833939,
9.34331120445838));
#39969=CARTESIAN_POINT('Ctrl Pts',(-4.06149293300488,-33.2803813268329,
9.694842779255));
#39970=CARTESIAN_POINT('Ctrl Pts',(-3.62979863535035,-33.2590307431067,
9.86459697759156));
#39971=CARTESIAN_POINT('Ctrl Pts',(-2.61783051914968,-33.2105362469365,
10.1870727448933));
#39972=CARTESIAN_POINT('Ctrl Pts',(-2.03284907472676,-33.1836409446823,
10.3197399799795));
#39973=CARTESIAN_POINT('Ctrl Pts',(-1.13606991607934,-33.1430286348071,
10.4438658339172));
#39974=CARTESIAN_POINT('Ctrl Pts',(-0.830699212903186,-33.1292897620925,
10.4725796083236));
#39975=CARTESIAN_POINT('Ctrl Pts',(0.060114311591093,-33.0889460452616,
10.5171304286933));
#39976=CARTESIAN_POINT('Ctrl Pts',(0.646146550315748,-33.0618783915075,
10.4974330077627));
#39977=CARTESIAN_POINT('Ctrl Pts',(1.76254461393008,-33.010148515081,10.3660369150008));
#39978=CARTESIAN_POINT('Ctrl Pts',(2.29200124002334,-32.985570223744,10.2619705275232));
#39979=CARTESIAN_POINT('Ctrl Pts',(3.42871971173839,-32.9322940999666,9.94614158870403));
#39980=CARTESIAN_POINT('Ctrl Pts',(4.02928450183857,-32.9038312804666,9.71836913395691));
#39981=CARTESIAN_POINT('Ctrl Pts',(4.92583995362263,-32.8586592000492,9.28085670850687));
#39982=CARTESIAN_POINT('Ctrl Pts',(5.23817635121195,-32.8422830250682,9.10822124185743));
#39983=CARTESIAN_POINT('Ctrl Pts',(5.9360015240174,-32.8044418227782,8.67473324104618));
#39984=CARTESIAN_POINT('Ctrl Pts',(6.31416943620977,-32.7830185409868,8.40347460828719));
#39985=CARTESIAN_POINT('Ctrl Pts',(7.13503851943344,-32.7344713780611,7.72787977332649));
#39986=CARTESIAN_POINT('Ctrl Pts',(7.56363051133854,-32.7075935546774,7.30892707934504));
#39987=CARTESIAN_POINT('Ctrl Pts',(8.15569447950756,-32.666912001127,6.62200001851131));
#39988=CARTESIAN_POINT('Ctrl Pts',(8.34676680538963,-32.6530835085583,6.37947623164878));
#39989=CARTESIAN_POINT('Ctrl Pts',(8.87134935273919,-32.6124326314509,5.64964597992332));
#39990=CARTESIAN_POINT('Ctrl Pts',(9.1747927854714,-32.5851389945684,5.14222466064249));
#39991=CARTESIAN_POINT('Ctrl Pts',(9.66988887554798,-32.5332666650535,4.12949538277679));
#39992=CARTESIAN_POINT('Ctrl Pts',(9.8684211523254,-32.508767778717,3.62956893963857));
#39993=CARTESIAN_POINT('Ctrl Pts',(10.1681068586645,-32.4631728371292,2.6653267239165));
#39994=CARTESIAN_POINT('Ctrl Pts',(10.2776883767546,-32.4420714192779,2.20524653635747));
#39995=CARTESIAN_POINT('Ctrl Pts',(10.3559140635165,-32.4208472785242,1.73955307739134));
#39996=CARTESIAN_POINT('Origin',(0.,-20.,0.));
#39997=CARTESIAN_POINT('',(10.3559140644695,-29.4200231052784,1.73955307171784));
#39998=CARTESIAN_POINT('',(10.355914067582,-30.237883364692,1.73955305318817));
#39999=CARTESIAN_POINT('',(10.355914065439,-20.,1.73955306594593));
#40000=CARTESIAN_POINT('Ctrl Pts',(10.355914067582,-30.237883364692,1.73955305318817));
#40001=CARTESIAN_POINT('Ctrl Pts',(10.3114209382312,-30.2501434056922,2.00442972556705));
#40002=CARTESIAN_POINT('Ctrl Pts',(10.2567761710981,-30.2625054479786,2.26753619013086));
#40003=CARTESIAN_POINT('Ctrl Pts',(10.0820564267382,-30.2959410316655,2.97186972395602));
#40004=CARTESIAN_POINT('Ctrl Pts',(9.94317807314309,-30.3169874168048,3.40779866310292));
#40005=CARTESIAN_POINT('Ctrl Pts',(9.57385491146637,-30.3631565176171,4.34971157992326));
#40006=CARTESIAN_POINT('Ctrl Pts',(9.33076649203003,-30.3880991411306,4.84927865134335));
#40007=CARTESIAN_POINT('Ctrl Pts',(8.88502861779431,-30.4275175836397,5.60644141465374));
#40008=CARTESIAN_POINT('Ctrl Pts',(8.70787865924656,-30.4420223380472,5.87781969895527));
#40009=CARTESIAN_POINT('Ctrl Pts',(8.30845915225981,-30.4728957279828,6.43191194896451));
#40010=CARTESIAN_POINT('Ctrl Pts',(8.08364542633716,-30.489350864679,6.71227573994664));
#40011=CARTESIAN_POINT('Ctrl Pts',(7.52939490863498,-30.5277414435198,7.33515542024652));
#40012=CARTESIAN_POINT('Ctrl Pts',(7.19018783800821,-30.5496311385861,7.66795289461622));
#40013=CARTESIAN_POINT('Ctrl Pts',(6.32995937279302,-30.6013788961666,8.40448202845157));
#40014=CARTESIAN_POINT('Ctrl Pts',(5.79118879226009,-30.6308856372514,8.78441008173817));
#40015=CARTESIAN_POINT('Ctrl Pts',(4.97272527999633,-30.6732036226496,9.25335046784924));
#40016=CARTESIAN_POINT('Ctrl Pts',(4.71935310668115,-30.6860106091723,9.38510492680094));
#40017=CARTESIAN_POINT('Ctrl Pts',(4.13939223540417,-30.7150184476288,9.65725564221272));
#40018=CARTESIAN_POINT('Ctrl Pts',(3.81041435540575,-30.7313259023401,9.79172519873317));
#40019=CARTESIAN_POINT('Ctrl Pts',(3.03603056528935,-30.7691257738906,10.0633085023197));
#40020=CARTESIAN_POINT('Ctrl Pts',(2.58703129253767,-30.7905772727537,10.187980121067));
#40021=CARTESIAN_POINT('Ctrl Pts',(1.4928232939646,-30.841607684484,10.414776413859));
#40022=CARTESIAN_POINT('Ctrl Pts',(0.843463013178343,-30.870836559206,10.4873581835484));
#40023=CARTESIAN_POINT('Ctrl Pts',(-0.0881747803281585,-30.9126415796335,
10.5043565938054));
#40024=CARTESIAN_POINT('Ctrl Pts',(-0.368005461647002,-30.9251980391295,
10.4982784745436));
#40025=CARTESIAN_POINT('Ctrl Pts',(-0.990582168471628,-30.9534506824108,
10.459831295581));
#40026=CARTESIAN_POINT('Ctrl Pts',(-1.33264996115336,-30.9692424697433,
10.421773096229));
#40027=CARTESIAN_POINT('Ctrl Pts',(-2.13383636408253,-31.006620875628,10.2925397906981));
#40028=CARTESIAN_POINT('Ctrl Pts',(-2.58996854881396,-31.0281734756231,
10.1873306652452));
#40029=CARTESIAN_POINT('Ctrl Pts',(-3.66171524524308,-31.0793098558509,
9.86346650533591));
#40030=CARTESIAN_POINT('Ctrl Pts',(-4.26694314194246,-31.1085460403157,
9.61713830124803));
#40031=CARTESIAN_POINT('Ctrl Pts',(-5.09552466190136,-31.1504467639704,
9.1861909744127));
#40032=CARTESIAN_POINT('Ctrl Pts',(-5.34029022692644,-31.1630970076259,
9.04609159653255));
#40033=CARTESIAN_POINT('Ctrl Pts',(-5.89828934047953,-31.1929261460113,
8.69615535105665));
#40034=CARTESIAN_POINT('Ctrl Pts',(-6.20644769996021,-31.2102414674031,
8.47896959673581));
#40035=CARTESIAN_POINT('Ctrl Pts',(-6.86161829068408,-31.2486841049203,
7.9623261161646));
#40036=CARTESIAN_POINT('Ctrl Pts',(-7.20207319923924,-31.2697605674337,
7.65575566726518));
#40037=CARTESIAN_POINT('Ctrl Pts',(-7.93599382821493,-31.3177570010518,
6.90245623910987));
#40038=CARTESIAN_POINT('Ctrl Pts',(-8.31369470361352,-31.3444305781048,
6.44254610247563));
#40039=CARTESIAN_POINT('Ctrl Pts',(-8.82173608076159,-31.3846310470289,
5.70431655461814));
#40040=CARTESIAN_POINT('Ctrl Pts',(-8.98217157755633,-31.3981715821894,
5.4481964953158));
#40041=CARTESIAN_POINT('Ctrl Pts',(-9.41496419997131,-31.4378225798877,
4.68607875418314));
#40042=CARTESIAN_POINT('Ctrl Pts',(-9.65712582975631,-31.4643767905422,
4.164224602004));
#40043=CARTESIAN_POINT('Ctrl Pts',(-10.0427664017817,-31.5157901472222,
3.11583356842777));
#40044=CARTESIAN_POINT('Ctrl Pts',(-10.1903673845999,-31.5405562692237,
2.59268448520782));
#40045=CARTESIAN_POINT('Ctrl Pts',(-10.3855356098675,-31.5854785372323,
1.61736055470674));
#40046=CARTESIAN_POINT('Ctrl Pts',(-10.4455090940491,-31.6056782382681,
1.16899405645754));
#40047=CARTESIAN_POINT('Ctrl Pts',(-10.4928009493489,-31.6367390070053,
0.479107454901651));
#40048=CARTESIAN_POINT('Ctrl Pts',(-10.501000940797,-31.647525162036,0.239566678794278));
#40049=CARTESIAN_POINT('Ctrl Pts',(-10.5009983454372,-31.6775509147193,
-0.421392116697277));
#40050=CARTESIAN_POINT('Ctrl Pts',(-10.4756367617688,-31.6969890494979,
-0.842353769006203));
#40051=CARTESIAN_POINT('Ctrl Pts',(-10.3561890637257,-31.7428354182167,
-1.83014236019911));
#40052=CARTESIAN_POINT('Ctrl Pts',(-10.2407712106508,-31.7691114954583,
-2.39305363997429));
#40053=CARTESIAN_POINT('Ctrl Pts',(-9.95108184501951,-31.8158885846558,
-3.38501340156538));
#40054=CARTESIAN_POINT('Ctrl Pts',(-9.79336889849711,-31.836466111034,-3.81736511616227));
#40055=CARTESIAN_POINT('Ctrl Pts',(-9.45828426385376,-31.8737271435713,
-4.5770262651996));
#40056=CARTESIAN_POINT('Ctrl Pts',(-9.29090075953251,-31.8903862934732,
-4.90789873504563));
#40057=CARTESIAN_POINT('Ctrl Pts',(-8.96560477009884,-31.9202273653525,
-5.47438083061892));
#40058=CARTESIAN_POINT('Ctrl Pts',(-8.81499189021383,-31.9332460764668,
-5.71374043635616));
#40059=CARTESIAN_POINT('Ctrl Pts',(-8.2853071829109,-31.9763480062886,-6.4846469219686));
#40060=CARTESIAN_POINT('Ctrl Pts',(-7.86635295102467,-32.0062814177709,
-6.98695156839824));
#40061=CARTESIAN_POINT('Ctrl Pts',(-7.07107196393841,-32.0570072298445,
-7.77757295859835));
#40062=CARTESIAN_POINT('Ctrl Pts',(-6.71691114952588,-32.0779705140793,
-8.08540714081939));
#40063=CARTESIAN_POINT('Ctrl Pts',(-6.07134772840634,-32.1143385237302,
-8.57474490007928));
#40064=CARTESIAN_POINT('Ctrl Pts',(-5.78944106251115,-32.1297031700912,
-8.76754711268758));
#40065=CARTESIAN_POINT('Ctrl Pts',(-4.95173434984063,-32.1746158973024,
-9.28242590236286));
#40066=CARTESIAN_POINT('Ctrl Pts',(-4.37515198478731,-32.2043698287966,
-9.567714566424));
#40067=CARTESIAN_POINT('Ctrl Pts',(-3.27633469656313,-32.2582570306378,
-9.99117249070295));
#40068=CARTESIAN_POINT('Ctrl Pts',(-2.76252637197646,-32.2824463257335,
-10.1452631861122));
#40069=CARTESIAN_POINT('Ctrl Pts',(-1.6528006352643,-32.3334627596567,-10.3874682261819));
#40070=CARTESIAN_POINT('Ctrl Pts',(-1.05652574309616,-32.3602061085662,
-10.4649410612404));
#40071=CARTESIAN_POINT('Ctrl Pts',(-0.138988744223851,-32.4022299754543,
-10.5049007721026));
#40072=CARTESIAN_POINT('Ctrl Pts',(0.179382258015516,-32.4169053736573,
-10.5042885408753));
#40073=CARTESIAN_POINT('Ctrl Pts',(1.0661158693777,-32.4578089392958,-10.4622538380019));
#40074=CARTESIAN_POINT('Ctrl Pts',(1.63187667674151,-32.4838947553008,-10.3890502014744));
#40075=CARTESIAN_POINT('Ctrl Pts',(2.6380321696595,-32.5304638734261,-10.1746084646372));
#40076=CARTESIAN_POINT('Ctrl Pts',(3.08039007694023,-32.5510193472215,-10.0495310022941));
#40077=CARTESIAN_POINT('Ctrl Pts',(3.86376117224199,-32.5883240812183,-9.77142666594091));
#40078=CARTESIAN_POINT('Ctrl Pts',(4.20750854472331,-32.6050495749781,-9.62841095747214));
#40079=CARTESIAN_POINT('Ctrl Pts',(4.79762630811627,-32.6349498040389,-9.34524375017742));
#40080=CARTESIAN_POINT('Ctrl Pts',(5.04727137012981,-32.647958979161,-9.21280891394702));
#40081=CARTESIAN_POINT('Ctrl Pts',(5.85485408900499,-32.6910427783843,-8.74170458658902));
#40082=CARTESIAN_POINT('Ctrl Pts',(6.38658555460328,-32.7209682805492,-8.3611171823797));
#40083=CARTESIAN_POINT('Ctrl Pts',(7.23344660815099,-32.7716726285021,-7.62677250465232));
#40084=CARTESIAN_POINT('Ctrl Pts',(7.56640801567001,-32.7926225551551,-7.29656649559687));
#40085=CARTESIAN_POINT('Ctrl Pts',(8.10244086634262,-32.8290081001699,-6.68868094722597));
#40086=CARTESIAN_POINT('Ctrl Pts',(8.31599369584715,-32.8444041521484,-6.42123403183101));
#40087=CARTESIAN_POINT('Ctrl Pts',(8.89230111013309,-32.8893955639791,-5.62240119121903));
#40088=CARTESIAN_POINT('Ctrl Pts',(9.21980186414363,-32.9191971254648,-5.06751232146032));
#40089=CARTESIAN_POINT('Ctrl Pts',(9.72367002799984,-32.9731670180818,-4.00112737558665));
#40090=CARTESIAN_POINT('Ctrl Pts',(9.91534738340422,-32.9973917420132,-3.49924072900911));
#40091=CARTESIAN_POINT('Ctrl Pts',(10.2380025681877,-33.0483735734034,-2.41095010255949));
#40092=CARTESIAN_POINT('Ctrl Pts',(10.3587719016882,-33.0750495258476,-1.82351684226819));
#40093=CARTESIAN_POINT('Ctrl Pts',(10.4660945912271,-33.1170096423701,-0.912811052212753));
#40094=CARTESIAN_POINT('Ctrl Pts',(10.4889567112825,-33.1316924997962,-0.595100631778317));
#40095=CARTESIAN_POINT('Ctrl Pts',(10.5123594700041,-33.1725940482051,0.292277987890723));
#40096=CARTESIAN_POINT('Ctrl Pts',(10.4810610962923,-33.1986703698459,0.861692218080709));
#40097=CARTESIAN_POINT('Ctrl Pts',(10.3893895420749,-33.2292338362686,1.53061625619924));
#40098=CARTESIAN_POINT('Ctrl Pts',(10.3734389374652,-33.2340135101075,1.63522392315164));
#40099=CARTESIAN_POINT('Ctrl Pts',(10.3559140834541,-33.2387841926166,1.73955295869885));
#40100=CARTESIAN_POINT('Ctrl Pts',(10.3559140635165,-32.4208472785242,1.73955307739134));
#40101=CARTESIAN_POINT('Ctrl Pts',(10.3840142550594,-32.4132231534421,1.57226690913973));
#40102=CARTESIAN_POINT('Ctrl Pts',(10.4080682925852,-32.4055801058559,1.40425654582014));
#40103=CARTESIAN_POINT('Ctrl Pts',(10.4726219990082,-32.3807349184809,0.859475314855344));
#40104=CARTESIAN_POINT('Ctrl Pts',(10.4968081321096,-32.363322230047,0.481156570534235));
#40105=CARTESIAN_POINT('Ctrl Pts',(10.5049559575085,-32.3248137670465,-0.354584559322483));
#40106=CARTESIAN_POINT('Ctrl Pts',(10.479577766544,-32.3037695734766,-0.811350842458339));
#40107=CARTESIAN_POINT('Ctrl Pts',(10.357674605056,-32.2575915458211,-1.81591241340187));
#40108=CARTESIAN_POINT('Ctrl Pts',(10.2472581585425,-32.2326382453559,-2.3606523309045));
#40109=CARTESIAN_POINT('Ctrl Pts',(10.0050968633665,-32.1932183520985,-3.20527982365404));
#40110=CARTESIAN_POINT('Ctrl Pts',(9.9015450378348,-32.1787229375252,-3.51214808074864));
#40111=CARTESIAN_POINT('Ctrl Pts',(9.65338821463296,-32.1478382856919,-4.14878388955609));
#40112=CARTESIAN_POINT('Ctrl Pts',(9.50567038336643,-32.1313617946604,-4.47688803502186));
#40113=CARTESIAN_POINT('Ctrl Pts',(9.12470734526825,-32.0929602648949,-5.21879242580949));
#40114=CARTESIAN_POINT('Ctrl Pts',(8.87964062678606,-32.0710813188292,-5.62566181672868));
#40115=CARTESIAN_POINT('Ctrl Pts',(8.23126914645556,-32.0193549055306,-6.55359562379191));
#40116=CARTESIAN_POINT('Ctrl Pts',(7.80483323400473,-31.9898585540253,-7.05606191798641));
#40117=CARTESIAN_POINT('Ctrl Pts',(7.12996222725747,-31.9475542432222,-7.71466684323306));
#40118=CARTESIAN_POINT('Ctrl Pts',(6.9176793353886,-31.9347507915757,-7.90557746905834));
#40119=CARTESIAN_POINT('Ctrl Pts',(6.4308744656234,-31.9061308667628,-8.30873332574502));
#40120=CARTESIAN_POINT('Ctrl Pts',(6.15308232009626,-31.8902184156436,-8.51649927805857));
#40121=CARTESIAN_POINT('Ctrl Pts',(5.47704407567159,-31.8526802623375,-8.97175315950345));
#40122=CARTESIAN_POINT('Ctrl Pts',(5.0714820920083,-31.8310902257059,-9.20708673399354));
#40123=CARTESIAN_POINT('Ctrl Pts',(4.06665395013364,-31.7798973590638,-9.70355424353606));
#40124=CARTESIAN_POINT('Ctrl Pts',(3.45607871398721,-31.75064201096,-9.93741325689463));
#40125=CARTESIAN_POINT('Ctrl Pts',(2.55570528502285,-31.7086985765141,-10.1891691013494));
#40126=CARTESIAN_POINT('Ctrl Pts',(2.28070312194563,-31.696023293501,-10.2542277342069));
#40127=CARTESIAN_POINT('Ctrl Pts',(1.63813055474699,-31.6663786520499,-10.3791138036064));
#40128=CARTESIAN_POINT('Ctrl Pts',(1.26933972813626,-31.6492792475789,-10.4306392692092));
#40129=CARTESIAN_POINT('Ctrl Pts',(0.441105333466639,-31.6109803849645,
-10.5017749605605));
#40130=CARTESIAN_POINT('Ctrl Pts',(-0.0184858864031121,-31.5898300287752,
-10.5110189764899));
#40131=CARTESIAN_POINT('Ctrl Pts',(-1.04623331237894,-31.542872224199,-10.4642657505435));
#40132=CARTESIAN_POINT('Ctrl Pts',(-1.61221589783784,-31.5172671051563,
-10.3921239795205));
#40133=CARTESIAN_POINT('Ctrl Pts',(-2.48082846590605,-31.4774403983088,
-10.2087071239322));
#40134=CARTESIAN_POINT('Ctrl Pts',(-2.78894922061996,-31.4631908145374,
-10.1288681297465));
#40135=CARTESIAN_POINT('Ctrl Pts',(-3.44887523637628,-31.4319707435517,
-9.92547051902809));
#40136=CARTESIAN_POINT('Ctrl Pts',(-3.79868502154433,-31.4148918552876,
-9.7969219746775));
#40137=CARTESIAN_POINT('Ctrl Pts',(-4.57130897833008,-31.3761692272211,
-9.46538340870905));
#40138=CARTESIAN_POINT('Ctrl Pts',(-4.98887166049275,-31.3545800935949,
-9.25210887202356));
#40139=CARTESIAN_POINT('Ctrl Pts',(-5.9506735976996,-31.3033886531654,-8.67675682069549));
#40140=CARTESIAN_POINT('Ctrl Pts',(-6.47812054188313,-31.2741338280961,
-8.29039217654382));
#40141=CARTESIAN_POINT('Ctrl Pts',(-7.1776665519186,-31.2321914486821,-7.67019504976522));
#40142=CARTESIAN_POINT('Ctrl Pts',(-7.38137989220433,-31.2195167317465,
-7.47435728305298));
#40143=CARTESIAN_POINT('Ctrl Pts',(-7.83465925603891,-31.1898682421523,
-7.00197556760979));
#40144=CARTESIAN_POINT('Ctrl Pts',(-8.07790154431399,-31.1727642891347,
-6.71989865895839));
#40145=CARTESIAN_POINT('Ctrl Pts',(-8.58659952401769,-31.1344624286685,
-6.06235346049053));
#40146=CARTESIAN_POINT('Ctrl Pts',(-8.84343503863315,-31.1133136620866,
-5.68115199575005));
#40147=CARTESIAN_POINT('Ctrl Pts',(-9.36124837711765,-31.0663477931969,
-4.79194460638085));
#40148=CARTESIAN_POINT('Ctrl Pts',(-9.60744622474524,-31.040733411439,-4.27699665616754));
#40149=CARTESIAN_POINT('Ctrl Pts',(-9.92403605650205,-31.0009047667007,
-3.44755162367288));
#40150=CARTESIAN_POINT('Ctrl Pts',(-10.0238697397609,-30.9866626265707,
-3.1454944946359));
#40151=CARTESIAN_POINT('Ctrl Pts',(-10.2726032240647,-30.9450737385001,
-2.25985786969892));
#40152=CARTESIAN_POINT('Ctrl Pts',(-10.3852276139088,-30.9172365074899,
-1.66743429848475));
#40153=CARTESIAN_POINT('Ctrl Pts',(-10.5008966525255,-30.8649396524904,
-0.536728397058647));
#40154=CARTESIAN_POINT('Ctrl Pts',(-10.5146055243678,-30.8405548193487,
-0.00141240271758721));
#40155=CARTESIAN_POINT('Ctrl Pts',(-10.4549714258338,-30.7874695772104,
1.17279641169983));
#40156=CARTESIAN_POINT('Ctrl Pts',(-10.3639128066585,-30.7590076115737,
1.80863771145195));
#40157=CARTESIAN_POINT('Ctrl Pts',(-10.1363803408681,-30.7145138031144,
2.76429783978136));
#40158=CARTESIAN_POINT('Ctrl Pts',(-10.0411628828829,-30.6988431170466,
3.09234276003793));
#40159=CARTESIAN_POINT('Ctrl Pts',(-9.77771090054407,-30.6615342781934,
3.85837356241474));
#40160=CARTESIAN_POINT('Ctrl Pts',(-9.59577594160446,-30.6399284224677,
4.29089399154376));
#40161=CARTESIAN_POINT('Ctrl Pts',(-9.09285357153487,-30.5887101334724,
5.29310052073904));
#40162=CARTESIAN_POINT('Ctrl Pts',(-8.74641206874312,-30.5594452052334,
5.84783705291487));
#40163=CARTESIAN_POINT('Ctrl Pts',(-8.17931770227677,-30.5174831260516,
6.59163727651354));
#40164=CARTESIAN_POINT('Ctrl Pts',(-7.99890840640879,-30.5047981949374,
6.80943323918334));
#40165=CARTESIAN_POINT('Ctrl Pts',(-7.56225810640245,-30.4752170860831,
7.29524017171099));
#40166=CARTESIAN_POINT('Ctrl Pts',(-7.3001791479172,-30.4581930889484,7.55748934682704));
#40167=CARTESIAN_POINT('Ctrl Pts',(-6.68307917688385,-30.4199437237763,
8.11287939219607));
#40168=CARTESIAN_POINT('Ctrl Pts',(-6.32152632643383,-30.398766799773,8.39765887737412));
#40169=CARTESIAN_POINT('Ctrl Pts',(-5.46946745949914,-30.3515947339942,
8.98248657036692));
#40170=CARTESIAN_POINT('Ctrl Pts',(-4.97064553220629,-30.3258082299517,
9.26783910066012));
#40171=CARTESIAN_POINT('Ctrl Pts',(-4.16436479706397,-30.2858726134788,
9.64516602787655));
#40172=CARTESIAN_POINT('Ctrl Pts',(-3.87180381808485,-30.2716960682433,
9.76628349993903));
#40173=CARTESIAN_POINT('Ctrl Pts',(-3.22071534644599,-30.2403892234577,
10.0019666444914));
#40174=CARTESIAN_POINT('Ctrl Pts',(-2.86060133255844,-30.2231445594521,
10.1108499331138));
#40175=CARTESIAN_POINT('Ctrl Pts',(-2.04209450231884,-30.1843322759005,
10.3110946018336));
#40176=CARTESIAN_POINT('Ctrl Pts',(-1.58185518085002,-30.1628211623334,
10.3916584936515));
#40177=CARTESIAN_POINT('Ctrl Pts',(-0.488861678338,-30.1126184177227,10.5086673993384));
#40178=CARTESIAN_POINT('Ctrl Pts',(0.144862686984379,-30.0842356954534,
10.5190357669805));
#40179=CARTESIAN_POINT('Ctrl Pts',(1.18351196804607,-30.0375139318949,10.442104678448));
#40180=CARTESIAN_POINT('Ctrl Pts',(1.58923252694197,-30.0191758100296,10.3880982672268));
#40181=CARTESIAN_POINT('Ctrl Pts',(2.62418553411945,-29.9710647030441,10.188268816762));
#40182=CARTESIAN_POINT('Ctrl Pts',(3.2449840613249,-29.9411576434855,10.0078599991273));
#40183=CARTESIAN_POINT('Ctrl Pts',(4.33730619894142,-29.8874258788518,9.57801309186354));
#40184=CARTESIAN_POINT('Ctrl Pts',(4.81399661233378,-29.8635324481433,9.34751391885331));
#40185=CARTESIAN_POINT('Ctrl Pts',(5.79477555919283,-29.8125842367779,8.77826357532591));
#40186=CARTESIAN_POINT('Ctrl Pts',(6.29098588323357,-29.7856360743672,8.42975819579932));
#40187=CARTESIAN_POINT('Ctrl Pts',(6.98779898456601,-29.7440177658387,7.84439748658059));
#40188=CARTESIAN_POINT('Ctrl Pts',(7.21253448021068,-29.7299672068071,7.63827535935543));
#40189=CARTESIAN_POINT('Ctrl Pts',(7.85039218361032,-29.6883834983211,6.99996121811215));
#40190=CARTESIAN_POINT('Ctrl Pts',(8.23595657125194,-29.6609979484456,6.54195421658664));
#40191=CARTESIAN_POINT('Ctrl Pts',(8.84642545299348,-29.6130703647771,5.67667088791222));
#40192=CARTESIAN_POINT('Ctrl Pts',(9.08724967439003,-29.5924236753169,5.28258781613396));
#40193=CARTESIAN_POINT('Ctrl Pts',(9.47124289689141,-29.5552931414778,4.54977980894248));
#40194=CARTESIAN_POINT('Ctrl Pts',(9.62403962162961,-29.5388356072143,4.21696526539511));
#40195=CARTESIAN_POINT('Ctrl Pts',(9.86377048822363,-29.5091712328099,3.613493397077));
#40196=CARTESIAN_POINT('Ctrl Pts',(9.95768563518622,-29.4961204860429,3.34601210295084));
#40197=CARTESIAN_POINT('Ctrl Pts',(10.174812874006,-29.4619524881759,2.6370503212561));
#40198=CARTESIAN_POINT('Ctrl Pts',(10.2800944753069,-29.4408860330383,2.19092254272531));
#40199=CARTESIAN_POINT('Ctrl Pts',(10.3559140644695,-29.4200231052784,1.73955307171784));
#40200=CARTESIAN_POINT('Origin',(0.,-20.,0.));
#40201=CARTESIAN_POINT('',(10.3559140653568,-26.421010256864,1.73955306643568));
#40202=CARTESIAN_POINT('',(10.3559140724569,-27.2388808356861,1.73955302416723));
#40203=CARTESIAN_POINT('',(10.355914065439,-20.,1.73955306594593));
#40204=CARTESIAN_POINT('',(-10.5009997442766,-28.659363079701,0.000175012915686588));
#40205=CARTESIAN_POINT('Ctrl Pts',(10.3559140724569,-27.2388808356861,1.73955302416722));
#40206=CARTESIAN_POINT('Ctrl Pts',(10.3180828494693,-27.2493073019969,1.96477001328604));
#40207=CARTESIAN_POINT('Ctrl Pts',(10.2728958110239,-27.2596885430775,2.18880581571025));
#40208=CARTESIAN_POINT('Ctrl Pts',(10.1134262702403,-27.2911089272256,2.86472517941119));
#40209=CARTESIAN_POINT('Ctrl Pts',(9.97639339121059,-27.3119500059299,3.3105317825855));
#40210=CARTESIAN_POINT('Ctrl Pts',(9.68387378266125,-27.3487618546298,4.07664467838913));
#40211=CARTESIAN_POINT('Ctrl Pts',(9.54088168897673,-27.3647000906728,4.40091086813838));
#40212=CARTESIAN_POINT('Ctrl Pts',(9.09416197629864,-27.4101343112315,5.28934135904937));
#40213=CARTESIAN_POINT('Ctrl Pts',(8.75483590697131,-27.4398061706659,5.83384743376745));
#40214=CARTESIAN_POINT('Ctrl Pts',(8.04268084402705,-27.4937429142223,6.7732053918681));
#40215=CARTESIAN_POINT('Ctrl Pts',(7.68479268516474,-27.518057718188,7.17669897934601));
#40216=CARTESIAN_POINT('Ctrl Pts',(6.87612615325683,-27.5685635894673,7.95822424585137));
#40217=CARTESIAN_POINT('Ctrl Pts',(6.4213824366526,-27.594680748428,8.32948279211632));
#40218=CARTESIAN_POINT('Ctrl Pts',(5.6849545944657,-27.6355180028049,8.83439047696996));
#40219=CARTESIAN_POINT('Ctrl Pts',(5.42438449889926,-27.6496644019845,8.99673352843451));
#40220=CARTESIAN_POINT('Ctrl Pts',(4.6353646234558,-27.6914035184841,9.44156226430721));
#40221=CARTESIAN_POINT('Ctrl Pts',(4.08942764429286,-27.718844201922,9.69052713554875));
#40222=CARTESIAN_POINT('Ctrl Pts',(3.08845432594339,-27.7669295098316,10.0472616435365));
#40223=CARTESIAN_POINT('Ctrl Pts',(2.64183411088289,-27.7876771652348,10.1738259242397));
#40224=CARTESIAN_POINT('Ctrl Pts',(1.83654892234962,-27.8246337000787,10.345406873886));
#40225=CARTESIAN_POINT('Ctrl Pts',(1.48117862572945,-27.8408131593276,10.4022334959532));
#40226=CARTESIAN_POINT('Ctrl Pts',(0.840717383057913,-27.8702424298845,
10.4711574645231));
#40227=CARTESIAN_POINT('Ctrl Pts',(0.556727091361961,-27.8833459232151,
10.4900904066511));
#40228=CARTESIAN_POINT('Ctrl Pts',(-0.382942286388455,-27.9266623387551,
10.5144669957549));
#40229=CARTESIAN_POINT('Ctrl Pts',(-1.03837704787873,-27.9567183264857,
10.4700752116207));
#40230=CARTESIAN_POINT('Ctrl Pts',(-2.15149850395256,-28.0077187142414,
10.2890744141875));
#40231=CARTESIAN_POINT('Ctrl Pts',(-2.61195964182773,-28.0288328340789,
10.18192853611));
#40232=CARTESIAN_POINT('Ctrl Pts',(-3.41197046532413,-28.0663896438696,
9.93791110791496));
#40233=CARTESIAN_POINT('Ctrl Pts',(-3.7545220412476,-28.0828051548399,9.81362214620951));
#40234=CARTESIAN_POINT('Ctrl Pts',(-4.38626810774778,-28.1141948299114,
9.54647441580841));
#40235=CARTESIAN_POINT('Ctrl Pts',(-4.67669008286196,-28.1290350255201,
9.40760805081518));
#40236=CARTESIAN_POINT('Ctrl Pts',(-5.45140776757648,-28.1695327478811,
8.99242144202319));
#40237=CARTESIAN_POINT('Ctrl Pts',(-5.92082141672377,-28.1950542989414,
8.69053446185361));
#40238=CARTESIAN_POINT('Ctrl Pts',(-6.72723033061127,-28.240957643741,8.07612670194272));
#40239=CARTESIAN_POINT('Ctrl Pts',(-7.07196400813563,-28.2614004113592,
7.77603890485064));
#40240=CARTESIAN_POINT('Ctrl Pts',(-7.6659279027653,-28.2989454914261,7.1867277991972));
#40241=CARTESIAN_POINT('Ctrl Pts',(-7.92103705659126,-28.316026769149,6.90454017823679));
#40242=CARTESIAN_POINT('Ctrl Pts',(-8.56357929590211,-28.3626608096505,
6.11119497484426));
#40243=CARTESIAN_POINT('Ctrl Pts',(-8.92045034996192,-28.392359382672,5.5773804859751));
#40244=CARTESIAN_POINT('Ctrl Pts',(-9.48210855297792,-28.4461840621296,
4.54393020349883));
#40245=CARTESIAN_POINT('Ctrl Pts',(-9.7014317690898,-28.4703648199866,4.05461788758502));
#40246=CARTESIAN_POINT('Ctrl Pts',(-9.99690660037589,-28.5096138125605,
3.23223990883031));
#40247=CARTESIAN_POINT('Ctrl Pts',(-10.0958687103838,-28.5247502312717,
2.9084273328655));
#40248=CARTESIAN_POINT('Ctrl Pts',(-10.2537437865664,-28.5536815988701,
2.28565133512126));
#40249=CARTESIAN_POINT('Ctrl Pts',(-10.3156242632665,-28.5674796602456,
1.9878013057817));
#40250=CARTESIAN_POINT('Ctrl Pts',(-10.4553393248025,-28.6073421346758,
1.12977722020661));
#40251=CARTESIAN_POINT('Ctrl Pts',(-10.5009905626262,-28.6334925450997,
0.565441235913797));
#40252=CARTESIAN_POINT('Ctrl Pts',(-10.5009999985369,-28.6593635075824,
0.000175291825331297));
#40253=CARTESIAN_POINT('Ctrl Pts',(-10.5009999985413,-28.6593635194262,
0.000175033045044792));
#40254=CARTESIAN_POINT('Ctrl Pts',(-10.5010159780912,-28.7032403165628,
-0.958508249417025));
#40255=CARTESIAN_POINT('Ctrl Pts',(-10.3697509234716,-28.7456685279049,
-1.91267464266642));
#40256=CARTESIAN_POINT('Ctrl Pts',(-9.94871668281961,-28.8161435099959,
-3.41388131545287));
#40257=CARTESIAN_POINT('Ctrl Pts',(-9.73728215636369,-28.8439059520432,
-3.97703908499111));
#40258=CARTESIAN_POINT('Ctrl Pts',(-9.24776380885242,-28.8962494509905,
-5.00383191503871));
#40259=CARTESIAN_POINT('Ctrl Pts',(-8.97977178860976,-28.9207477341447,
-5.47020947191444));
#40260=CARTESIAN_POINT('Ctrl Pts',(-8.31549791319486,-28.9740076374205,
-6.44485365416914));
#40261=CARTESIAN_POINT('Ctrl Pts',(-7.90578322545317,-29.0025301998082,
-6.94134107903262));
#40262=CARTESIAN_POINT('Ctrl Pts',(-7.18642390871803,-29.0487787006893,
-7.66614792613423));
#40263=CARTESIAN_POINT('Ctrl Pts',(-6.90521670990436,-29.066191591194,-7.92038370704367));
#40264=CARTESIAN_POINT('Ctrl Pts',(-6.25584606237276,-29.104700174073,-8.44655067622578));
#40265=CARTESIAN_POINT('Ctrl Pts',(-5.8823879276126,-29.1257442841134,-8.71076064571559));
#40266=CARTESIAN_POINT('Ctrl Pts',(-5.01993443084397,-29.1719225123286,
-9.24008800767182));
#40267=CARTESIAN_POINT('Ctrl Pts',(-4.52469124889504,-29.1968760850498,
-9.4924262051184));
#40268=CARTESIAN_POINT('Ctrl Pts',(-3.71268461556848,-29.2362959981014,
-9.82811025550976));
#40269=CARTESIAN_POINT('Ctrl Pts',(-3.40798994745766,-29.2507911570666,
-9.93787598289074));
#40270=CARTESIAN_POINT('Ctrl Pts',(-2.75512093712771,-29.2816760325669,
-10.1395082730866));
#40271=CARTESIAN_POINT('Ctrl Pts',(-2.406312663009,-29.298153021054,-10.2279011969941));
#40272=CARTESIAN_POINT('Ctrl Pts',(-1.58841301769394,-29.3365547874104,
-10.3910065557595));
#40273=CARTESIAN_POINT('Ctrl Pts',(-1.11739699517865,-29.3584334646503,
-10.4521532292869));
#40274=CARTESIAN_POINT('Ctrl Pts',(0.0124719635250474,-29.4101593475656,
-10.5215609332356));
#40275=CARTESIAN_POINT('Ctrl Pts',(0.671147752100753,-29.4396554426413,
-10.5001421397514));
#40276=CARTESIAN_POINT('Ctrl Pts',(1.6066009404367,-29.4819594228499,-10.3812946328334));
#40277=CARTESIAN_POINT('Ctrl Pts',(1.8881221407293,-29.4947627948844,-10.3338006686585));
#40278=CARTESIAN_POINT('Ctrl Pts',(2.50656935637032,-29.5233820560201,-10.203347342019));
#40279=CARTESIAN_POINT('Ctrl Pts',(2.84202195402001,-29.5392939080835,-10.1150424741783));
#40280=CARTESIAN_POINT('Ctrl Pts',(3.61896460480308,-29.576831635684,-9.86881276084557));
#40281=CARTESIAN_POINT('Ctrl Pts',(4.05548667073814,-29.5984218541339,-9.69759806125798));
#40282=CARTESIAN_POINT('Ctrl Pts',(5.0692057690414,-29.64961499523,-9.21953331955728));
#40283=CARTESIAN_POINT('Ctrl Pts',(5.63207864372681,-29.678870436657,-8.88686417805851));
#40284=CARTESIAN_POINT('Ctrl Pts',(6.38920730795728,-29.7208140888407,-8.33839481878914));
#40285=CARTESIAN_POINT('Ctrl Pts',(6.61119126154604,-29.7334895044116,-8.16351302791474));
#40286=CARTESIAN_POINT('Ctrl Pts',(7.10861180975288,-29.7631330276903,-7.73802899177771));
#40287=CARTESIAN_POINT('Ctrl Pts',(7.37830861116425,-29.7802311437628,-7.48131007427148));
#40288=CARTESIAN_POINT('Ctrl Pts',(7.94912188714333,-29.8185291399234,-6.87701393956899));
#40289=CARTESIAN_POINT('Ctrl Pts',(8.24220991703396,-29.83967992921,-6.52287096297466));
#40290=CARTESIAN_POINT('Ctrl Pts',(8.84477725295011,-29.8866353695719,-5.68905149860153));
#40291=CARTESIAN_POINT('Ctrl Pts',(9.14027185246643,-29.9122378040575,-5.20104231234018));
#40292=CARTESIAN_POINT('Ctrl Pts',(9.53688871543161,-29.9520639329772,-4.40681239448226));
#40293=CARTESIAN_POINT('Ctrl Pts',(9.6660291135003,-29.9663156573816,-4.11583762468849));
#40294=CARTESIAN_POINT('Ctrl Pts',(10.000150471512,-30.0078459950931,-3.2601406203456));
#40295=CARTESIAN_POINT('Ctrl Pts',(10.1701629987673,-30.0356121576088,-2.68314482244037));
#40296=CARTESIAN_POINT('Ctrl Pts',(10.3967615251233,-30.0878785218362,-1.57006935790534));
#40297=CARTESIAN_POINT('Ctrl Pts',(10.4632942658359,-30.1123015279016,-1.03791360590769));
#40298=CARTESIAN_POINT('Ctrl Pts',(10.5196374656649,-30.1654127494571,0.136998416030386));
#40299=CARTESIAN_POINT('Ctrl Pts',(10.4916887195404,-30.1938636642477,0.778453020532126));
#40300=CARTESIAN_POINT('Ctrl Pts',(10.3906475481905,-30.2278632658661,1.52234894139183));
#40301=CARTESIAN_POINT('Ctrl Pts',(10.3741317555963,-30.2328634974621,1.63109944135982));
#40302=CARTESIAN_POINT('Ctrl Pts',(10.355914067582,-30.237883364692,1.73955305318817));
#40303=CARTESIAN_POINT('Ctrl Pts',(10.3559140644695,-29.4200231052784,1.73955307171784));
#40304=CARTESIAN_POINT('Ctrl Pts',(10.3882514180482,-29.4111249843691,1.54704221351056));
#40305=CARTESIAN_POINT('Ctrl Pts',(10.4152294293614,-29.4022599014847,1.35357803988769));
#40306=CARTESIAN_POINT('Ctrl Pts',(10.4886797662756,-29.3721694805024,0.692376564764958));
#40307=CARTESIAN_POINT('Ctrl Pts',(10.5091543523562,-29.3511563112863,0.222412656287216));
#40308=CARTESIAN_POINT('Ctrl Pts',(10.4901081552782,-29.3148513170984,-0.585977830036988));
#40309=CARTESIAN_POINT('Ctrl Pts',(10.4657500100927,-29.2996015140767,-0.92401988760244));
#40310=CARTESIAN_POINT('Ctrl Pts',(10.3913488019059,-29.2712846666844,-1.5394619260401));
#40311=CARTESIAN_POINT('Ctrl Pts',(10.3464009860695,-29.2583356301667,-1.81715629619735));
#40312=CARTESIAN_POINT('Ctrl Pts',(10.1604649521611,-29.2153416361916,-2.73144948308473));
#40313=CARTESIAN_POINT('Ctrl Pts',(9.97137368277822,-29.1854419308269,-3.35672624592777));
#40314=CARTESIAN_POINT('Ctrl Pts',(9.54949020362022,-29.1348354722116,-4.39273379916829));
#40315=CARTESIAN_POINT('Ctrl Pts',(9.34482163715318,-29.1139560856025,-4.81281480532517));
#40316=CARTESIAN_POINT('Ctrl Pts',(8.92613363013922,-29.0761303892706,-5.54404122658911));
#40317=CARTESIAN_POINT('Ctrl Pts',(8.72201361298073,-29.0592038169332,-5.85992567880135));
#40318=CARTESIAN_POINT('Ctrl Pts',(8.31558950328292,-29.0275252066659,-6.42044893060744));
#40319=CARTESIAN_POINT('Ctrl Pts',(8.11829189113292,-29.0129279808966,-6.66817273704267));
#40320=CARTESIAN_POINT('Ctrl Pts',(7.53289270146217,-28.9719163864058,-7.33862828664863));
#40321=CARTESIAN_POINT('Ctrl Pts',(7.12090889826163,-28.9456457421507,-7.73903235280617));
#40322=CARTESIAN_POINT('Ctrl Pts',(6.32352711747758,-28.8988747719585,-8.39614989545271));
#40323=CARTESIAN_POINT('Ctrl Pts',(5.94995049114923,-28.8782980508495,-8.66489599617427));
#40324=CARTESIAN_POINT('Ctrl Pts',(5.2455679906524,-28.8410353906503,-9.10452461256085));
#40325=CARTESIAN_POINT('Ctrl Pts',(4.92101182835862,-28.8243737855605,-9.28396417582404));
#40326=CARTESIAN_POINT('Ctrl Pts',(4.33336691403082,-28.7945305032247,-9.56936996621308));
#40327=CARTESIAN_POINT('Ctrl Pts',(4.07420699020443,-28.7815121233764,-9.68254848627957));
#40328=CARTESIAN_POINT('Ctrl Pts',(3.20264201786614,-28.7384108117789,-10.0219776853919));
#40329=CARTESIAN_POINT('Ctrl Pts',(2.57371132311182,-28.708477663395,-10.2016176558485));
#40330=CARTESIAN_POINT('Ctrl Pts',(1.47146700095473,-28.6577525681425,-10.4079524862632));
#40331=CARTESIAN_POINT('Ctrl Pts',(1.00550151449754,-28.6367897308613,-10.4632528868755));
#40332=CARTESIAN_POINT('Ctrl Pts',(0.196484823715644,-28.6004210999217,
-10.5047096051332));
#40333=CARTESIAN_POINT('Ctrl Pts',(-0.145070787774148,-28.5850553676004,
-10.5055452732831));
#40334=CARTESIAN_POINT('Ctrl Pts',(-1.12856998013108,-28.5400847485141,
-10.4599728064761));
#40335=CARTESIAN_POINT('Ctrl Pts',(-1.76698463185707,-28.5102728697013,
-10.3712332939238));
#40336=CARTESIAN_POINT('Ctrl Pts',(-2.91596786470437,-28.4562759682354,
-10.102292907271));
#40337=CARTESIAN_POINT('Ctrl Pts',(-3.42852853124,-28.4320347323068,-9.94004039345127));
#40338=CARTESIAN_POINT('Ctrl Pts',(-4.47456880458602,-28.3813798654914,
-9.51832511460139));
#40339=CARTESIAN_POINT('Ctrl Pts',(-5.0030487517424,-28.3550454604031,-9.25147415733906));
#40340=CARTESIAN_POINT('Ctrl Pts',(-5.76934019186021,-28.3138825271998,
-8.77958769831603));
#40341=CARTESIAN_POINT('Ctrl Pts',(-6.02512532155903,-28.2996390276929,
-8.60606232902924));
#40342=CARTESIAN_POINT('Ctrl Pts',(-6.75167554736299,-28.2578921707579,
-8.06488101360722));
#40343=CARTESIAN_POINT('Ctrl Pts',(-7.19919120879324,-28.2305424207394,
-7.66805748587392));
#40344=CARTESIAN_POINT('Ctrl Pts',(-7.93065471190074,-28.1825071544331,
-6.89866199727752));
#40345=CARTESIAN_POINT('Ctrl Pts',(-8.22805239524048,-28.1617223235682,
-6.5410992917377));
#40346=CARTESIAN_POINT('Ctrl Pts',(-8.71064440030622,-28.1248251234706,
-5.87566485854064));
#40347=CARTESIAN_POINT('Ctrl Pts',(-8.9055762136924,-28.1087433876614,-5.57579341790175));
#40348=CARTESIAN_POINT('Ctrl Pts',(-9.40599703178863,-28.0631569431029,
-4.71256572311404));
#40349=CARTESIAN_POINT('Ctrl Pts',(-9.67580842618505,-28.0334795771426,
-4.13035115468015));
#40350=CARTESIAN_POINT('Ctrl Pts',(-10.0716088133229,-27.9795617196811,
-3.02045273726026));
#40351=CARTESIAN_POINT('Ctrl Pts',(-10.2131095201338,-27.9552704449761,
-2.50057056438467));
#40352=CARTESIAN_POINT('Ctrl Pts',(-10.4245064791403,-27.9047175492257,
-1.39497431273176));
#40353=CARTESIAN_POINT('Ctrl Pts',(-10.4862215696626,-27.8785315067934,
-0.809591135208093));
#40354=CARTESIAN_POINT('Ctrl Pts',(-10.5051552217517,-27.8375911542391,
0.0853302118330865));
#40355=CARTESIAN_POINT('Ctrl Pts',(-10.4981514607938,-27.823414124343,0.392913377762777));
#40356=CARTESIAN_POINT('Ctrl Pts',(-10.4377355873879,-27.7816344134869,
1.29755611611818));
#40357=CARTESIAN_POINT('Ctrl Pts',(-10.3467201052374,-27.7541850038887,
1.8908703384309));
#40358=CARTESIAN_POINT('Ctrl Pts',(-10.0962332646097,-27.7060610410738,
2.92450402369313));
#40359=CARTESIAN_POINT('Ctrl Pts',(-9.95704563782578,-27.6852841319234,
3.36807018280015));
#40360=CARTESIAN_POINT('Ctrl Pts',(-9.65940668052789,-27.6483744816745,
4.13460533706184));
#40361=CARTESIAN_POINT('Ctrl Pts',(-9.51288954591326,-27.6322721124704,
4.46139302570563));
#40362=CARTESIAN_POINT('Ctrl Pts',(-9.05844385609214,-27.5866607065496,
5.35030438420042));
#40363=CARTESIAN_POINT('Ctrl Pts',(-8.71535936462651,-27.556979428553,5.89268077780341));
#40364=CARTESIAN_POINT('Ctrl Pts',(-7.99709418191676,-27.5030579396915,
6.82692606138143));
#40365=CARTESIAN_POINT('Ctrl Pts',(-7.63688993954271,-27.4787668262038,
7.22761144806861));
#40366=CARTESIAN_POINT('Ctrl Pts',(-6.82233854457238,-27.4282136065641,
8.00449861949725));
#40367=CARTESIAN_POINT('Ctrl Pts',(-6.36383370309586,-27.4020270905609,
8.37364400443418));
#40368=CARTESIAN_POINT('Ctrl Pts',(-5.62200618322968,-27.3610860287691,
8.87460515951703));
#40369=CARTESIAN_POINT('Ctrl Pts',(-5.35971855129559,-27.3469087878769,
9.03542942258841));
#40370=CARTESIAN_POINT('Ctrl Pts',(-4.56672153109829,-27.3051288115258,
9.47496870904137));
#40371=CARTESIAN_POINT('Ctrl Pts',(-4.01877905382267,-27.2776793556659,
9.72005267491154));
#40372=CARTESIAN_POINT('Ctrl Pts',(-3.01436264259617,-27.2295551453468,
10.069770207401));
#40373=CARTESIAN_POINT('Ctrl Pts',(-2.56615374137642,-27.2087780398319,
10.1932092011323));
#40374=CARTESIAN_POINT('Ctrl Pts',(-1.76065882230906,-27.1718686995197,
10.3585313093272));
#40375=CARTESIAN_POINT('Ctrl Pts',(-1.40663220683728,-27.155766843081,10.412515197553));
#40376=CARTESIAN_POINT('Ctrl Pts',(-0.413356374842349,-27.1101580262109,
10.5123851134107));
#40377=CARTESIAN_POINT('Ctrl Pts',(0.228351446452501,-27.0804788532733,
10.5180308699488));
#40378=CARTESIAN_POINT('Ctrl Pts',(1.40268231402333,-27.0265613658597,10.4207902608575));
#40379=CARTESIAN_POINT('Ctrl Pts',(1.93459759480564,-27.0022721538639,10.3352668020732));
#40380=CARTESIAN_POINT('Ctrl Pts',(3.02904937430544,-26.9517151118528,10.0718077381626));
#40381=CARTESIAN_POINT('Ctrl Pts',(3.58790235402662,-26.92552300815,9.88652617813119));
#40382=CARTESIAN_POINT('Ctrl Pts',(4.41112952875803,-26.8845735774232,9.53454453000986));
#40383=CARTESIAN_POINT('Ctrl Pts',(4.68848734744332,-26.8703938464143,9.40125986480505));
#40384=CARTESIAN_POINT('Ctrl Pts',(5.48771639964782,-26.8286107509462,8.97301308299686));
#40385=CARTESIAN_POINT('Ctrl Pts',(5.99066492886825,-26.801160763006,8.64534327207123));
#40386=CARTESIAN_POINT('Ctrl Pts',(6.82898261893844,-26.7530336505182,7.99072591469196));
#40387=CARTESIAN_POINT('Ctrl Pts',(7.17567339136795,-26.7322542327136,7.68091272566604));
#40388=CARTESIAN_POINT('Ctrl Pts',(7.75109503258679,-26.6953485369991,7.09362517231805));
#40389=CARTESIAN_POINT('Ctrl Pts',(7.98824421975867,-26.6792527136377,6.82546284931496));
#40390=CARTESIAN_POINT('Ctrl Pts',(8.61063702296856,-26.6336350177861,6.04470486401708));
#40391=CARTESIAN_POINT('Ctrl Pts',(8.96333652530217,-26.6039404892241,5.50818833421027));
#40392=CARTESIAN_POINT('Ctrl Pts',(9.51831946706771,-26.549991857334,4.46792743750132));
#40393=CARTESIAN_POINT('Ctrl Pts',(9.73481368309964,-26.5256868761265,3.97419224801561));
#40394=CARTESIAN_POINT('Ctrl Pts',(10.1061475258653,-26.4751614096877,2.91221475488355));
#40395=CARTESIAN_POINT('Ctrl Pts',(10.2530385291071,-26.4490155272709,2.3431614259462));
#40396=CARTESIAN_POINT('Ctrl Pts',(10.3530739892064,-26.4217918282755,1.75639771377517));
#40397=CARTESIAN_POINT('Ctrl Pts',(10.3544991746734,-26.4214010862009,1.74797619914241));
#40398=CARTESIAN_POINT('Ctrl Pts',(10.3559140653568,-26.421010256864,1.73955306643568));
#40399=CARTESIAN_POINT('Origin',(0.,-20.,0.));
#40400=CARTESIAN_POINT('',(10.3559140377345,-23.4201872127662,1.73955323087673));
#40401=CARTESIAN_POINT('',(10.3559140709193,-24.2381415361801,1.73955303332087));
#40402=CARTESIAN_POINT('',(10.355914065439,-20.,1.73955306594593));
#40403=CARTESIAN_POINT('Ctrl Pts',(10.3559140709193,-24.2381415361801,1.73955303332087));
#40404=CARTESIAN_POINT('Ctrl Pts',(10.324487938485,-24.2466601328659,1.92663921053825));
#40405=CARTESIAN_POINT('Ctrl Pts',(10.2879944391612,-24.2551927625748,2.11285960877395));
#40406=CARTESIAN_POINT('Ctrl Pts',(10.1182336378067,-24.2902807135696,2.86979724878587));
#40407=CARTESIAN_POINT('Ctrl Pts',(9.94236392548783,-24.3173779275724,3.42983186070435));
#40408=CARTESIAN_POINT('Ctrl Pts',(9.51698971186189,-24.3691263055226,4.47078879368452));
#40409=CARTESIAN_POINT('Ctrl Pts',(9.27521321078572,-24.3936940741653,4.95292735996964));
#40410=CARTESIAN_POINT('Ctrl Pts',(8.66699740385356,-24.4469621869336,5.9636461937184));
#40411=CARTESIAN_POINT('Ctrl Pts',(8.2868841451409,-24.4754272278359,6.48146988670358));
#40412=CARTESIAN_POINT('Ctrl Pts',(7.62456677287723,-24.5206666298982,7.22946709848752));
#40413=CARTESIAN_POINT('Ctrl Pts',(7.37364549015571,-24.5371090576338,7.48522212436666));
#40414=CARTESIAN_POINT('Ctrl Pts',(6.76847199429934,-24.5749904610049,8.04203810592781));
#40415=CARTESIAN_POINT('Ctrl Pts',(6.40630343053227,-24.5963869157273,8.33341926642748));
#40416=CARTESIAN_POINT('Ctrl Pts',(5.53541274582119,-24.6449447373298,8.94366321381699));
#40417=CARTESIAN_POINT('Ctrl Pts',(5.01626121662686,-24.6718579121132,9.24483912236207));
#40418=CARTESIAN_POINT('Ctrl Pts',(4.19608292035302,-24.712526852402,9.63111810984119));
#40419=CARTESIAN_POINT('Ctrl Pts',(3.91228822633343,-24.7263059673185,9.74984846907212));
#40420=CARTESIAN_POINT('Ctrl Pts',(3.07224379358609,-24.7667880875886,10.058704051096));
#40421=CARTESIAN_POINT('Ctrl Pts',(2.50476368166444,-24.7939577084118,10.2148091789403));
#40422=CARTESIAN_POINT('Ctrl Pts',(1.39835422386016,-24.8457516018512,10.4213756409963));
#40423=CARTESIAN_POINT('Ctrl Pts',(0.862657737827972,-24.8702937958779,
10.4793277585888));
#40424=CARTESIAN_POINT('Ctrl Pts',(-0.315682587887609,-24.9235290904774,
10.5158001253286));
#40425=CARTESIAN_POINT('Ctrl Pts',(-0.956700476789631,-24.9519867382644,
10.4769467269681));
#40426=CARTESIAN_POINT('Ctrl Pts',(-1.94608698095275,-24.9973108142846,
10.3253767058593));
#40427=CARTESIAN_POINT('Ctrl Pts',(-2.2989640436574,-25.0138473733298,10.2525805469767));
#40428=CARTESIAN_POINT('Ctrl Pts',(-3.09595440814296,-25.0517865568668,
10.0449455584571));
#40429=CARTESIAN_POINT('Ctrl Pts',(-3.53629243011848,-25.0731455955327,
9.89851055047748));
#40430=CARTESIAN_POINT('Ctrl Pts',(-4.51998909658421,-25.1216522668389,
9.49732996439393));
#40431=CARTESIAN_POINT('Ctrl Pts',(-5.05411063215014,-25.1485513465259,
9.22418367733075));
#40432=CARTESIAN_POINT('Ctrl Pts',(-5.82221778999046,-25.1891743890039,
8.74453365071616));
#40433=CARTESIAN_POINT('Ctrl Pts',(-6.07514792543899,-25.2029204880705,
8.5707445924514));
#40434=CARTESIAN_POINT('Ctrl Pts',(-6.78788954817592,-25.2432891502633,
8.0335959312419));
#40435=CARTESIAN_POINT('Ctrl Pts',(-7.22534305985099,-25.2703752097324,
7.64254438229231));
#40436=CARTESIAN_POINT('Ctrl Pts',(-7.99808801740006,-25.3221165935984,
6.82581303906658));
#40437=CARTESIAN_POINT('Ctrl Pts',(-8.33763701369675,-25.3466883205253,
6.40663472829547));
#40438=CARTESIAN_POINT('Ctrl Pts',(-9.00747178856978,-25.3999537393579,
5.43573215714895));
#40439=CARTESIAN_POINT('Ctrl Pts',(-9.32235157281206,-25.4284124736759,
4.87601006088883));
#40440=CARTESIAN_POINT('Ctrl Pts',(-9.73005546617197,-25.473589476729,3.96539573671134));
#40441=CARTESIAN_POINT('Ctrl Pts',(-9.85917630460047,-25.4899749751795,
3.63248819485952));
#40442=CARTESIAN_POINT('Ctrl Pts',(-10.1168812261931,-25.5278217961119,
2.85232379282939));
#40443=CARTESIAN_POINT('Ctrl Pts',(-10.2332049247408,-25.5492412627006,
2.40178350380998));
#40444=CARTESIAN_POINT('Ctrl Pts',(-10.4401845279722,-25.6002691438484,
1.30365312682006));
#40445=CARTESIAN_POINT('Ctrl Pts',(-10.5010165906538,-25.6295253206722,
0.652408809668201));
#40446=CARTESIAN_POINT('Ctrl Pts',(-10.500989925391,-25.6765803594897,-0.396387287871056));
#40447=CARTESIAN_POINT('Ctrl Pts',(-10.4785667799993,-25.694365129117,-0.792178141498095));
#40448=CARTESIAN_POINT('Ctrl Pts',(-10.3613394950743,-25.7417835205261,
-1.82369462712537));
#40449=CARTESIAN_POINT('Ctrl Pts',(-10.2304880564737,-25.7715417106329,
-2.45363924603205));
#40450=CARTESIAN_POINT('Ctrl Pts',(-9.88647827046607,-25.8254287562713,
-3.5798520113043));
#40451=CARTESIAN_POINT('Ctrl Pts',(-9.69108059040702,-25.8496138822996,
-4.07931002618793));
#40452=CARTESIAN_POINT('Ctrl Pts',(-9.19762431485055,-25.9006343639578,
-5.10246730907822));
#40453=CARTESIAN_POINT('Ctrl Pts',(-8.89092518171722,-25.9273856157321,
-5.61986717440523));
#40454=CARTESIAN_POINT('Ctrl Pts',(-8.35661210688886,-25.969416823983,-6.36704628567195));
#40455=CARTESIAN_POINT('Ctrl Pts',(-8.15986176121085,-25.984091212231,-6.61731803590292));
#40456=CARTESIAN_POINT('Ctrl Pts',(-7.58007650684482,-26.0249950507928,
-7.28956992978709));
#40457=CARTESIAN_POINT('Ctrl Pts',(-7.1736182037361,-26.051082152157,-7.68990368212843));
#40458=CARTESIAN_POINT('Ctrl Pts',(-6.38444491515332,-26.0976523350784,
-8.34989403290927));
#40459=CARTESIAN_POINT('Ctrl Pts',(-6.01324674143197,-26.1182076274909,
-8.62106351431982));
#40460=CARTESIAN_POINT('Ctrl Pts',(-5.31131245965022,-26.1555127252341,
-9.06638840623387));
#40461=CARTESIAN_POINT('Ctrl Pts',(-4.98677184026508,-26.1722387689039,
-9.24886704550868));
#40462=CARTESIAN_POINT('Ctrl Pts',(-4.39999243575498,-26.2021394902377,
-9.53891317575588));
#40463=CARTESIAN_POINT('Ctrl Pts',(-4.14181100974971,-26.2151485882327,
-9.65381774195569));
#40464=CARTESIAN_POINT('Ctrl Pts',(-3.27300226131473,-26.2582322453998,
-9.99920845997779));
#40465=CARTESIAN_POINT('Ctrl Pts',(-2.64552823940767,-26.2881576880921,
-10.1832182567101));
#40466=CARTESIAN_POINT('Ctrl Pts',(-1.54524586309445,-26.338861869509,-10.3972410569353));
#40467=CARTESIAN_POINT('Ctrl Pts',(-1.07998652906133,-26.3598116907492,
-10.4558136787306));
#40468=CARTESIAN_POINT('Ctrl Pts',(-0.270896018139364,-26.3961973752654,
-10.5030766931263));
#40469=CARTESIAN_POINT('Ctrl Pts',(0.071340704784431,-26.4115936761907,
-10.5063272370803));
#40470=CARTESIAN_POINT('Ctrl Pts',(1.05460639196492,-26.4565397577758,-10.4676137279418));
#40471=CARTESIAN_POINT('Ctrl Pts',(1.69241871094522,-26.4862948003017,-10.3835862733447));
#40472=CARTESIAN_POINT('Ctrl Pts',(2.84082739009004,-26.540176754067,-10.1236082251032));
#40473=CARTESIAN_POINT('Ctrl Pts',(3.35329434407156,-26.5643599008276,-9.96559988560545));
#40474=CARTESIAN_POINT('Ctrl Pts',(4.41010538544358,-26.615382302051,-9.54895493657161));
#40475=CARTESIAN_POINT('Ctrl Pts',(4.94879637738572,-26.6421373033285,-9.28121631427281));
#40476=CARTESIAN_POINT('Ctrl Pts',(5.73341078880083,-26.6841719841633,-8.80342196799812));
#40477=CARTESIAN_POINT('Ctrl Pts',(5.99750260540311,-26.6988458826237,-8.62567085850713));
#40478=CARTESIAN_POINT('Ctrl Pts',(6.71068601229851,-26.7397498535273,-8.09704254545277));
#40479=CARTESIAN_POINT('Ctrl Pts',(7.13991577908143,-26.765837578229,-7.72120680789644));
#40480=CARTESIAN_POINT('Ctrl Pts',(7.85631652329748,-26.8124082775159,-6.98284727235599));
#40481=CARTESIAN_POINT('Ctrl Pts',(8.15412139751634,-26.8329634819584,-6.63265971039695));
#40482=CARTESIAN_POINT('Ctrl Pts',(8.65000251261382,-26.8702687561498,-5.96547565715465));
#40483=CARTESIAN_POINT('Ctrl Pts',(8.85592167238629,-26.8869950665565,-5.65527106798478));
#40484=CARTESIAN_POINT('Ctrl Pts',(9.18845369441323,-26.9168960266871,-5.09147486122319));
#40485=CARTESIAN_POINT('Ctrl Pts',(9.32208504064439,-26.9299050872885,-4.84247100950633));
#40486=CARTESIAN_POINT('Ctrl Pts',(9.73060653772764,-26.9729886756051,-4.0015008607191));
#40487=CARTESIAN_POINT('Ctrl Pts',(9.96038934011534,-27.0029140894856,-3.3893062747658));
#40488=CARTESIAN_POINT('Ctrl Pts',(10.2549714620511,-27.0536181901952,-2.30780535843868));
#40489=CARTESIAN_POINT('Ctrl Pts',(10.3476959451791,-27.0745679603403,-1.84813368023866));
#40490=CARTESIAN_POINT('Ctrl Pts',(10.4544987947741,-27.1109537124791,-1.04473034767586));
#40491=CARTESIAN_POINT('Ctrl Pts',(10.4829796544845,-27.1263501340767,-0.703662523753121));
#40492=CARTESIAN_POINT('Ctrl Pts',(10.5044217982251,-27.1547753299759,-0.0817046725738455));
#40493=CARTESIAN_POINT('Ctrl Pts',(10.5028605497905,-27.1676811210334,0.198672253356716));
#40494=CARTESIAN_POINT('Ctrl Pts',(10.4707928935629,-27.200100246433,0.901470012425277));
#40495=CARTESIAN_POINT('Ctrl Pts',(10.4259632367834,-27.2195749503812,1.3225360568573));
#40496=CARTESIAN_POINT('Ctrl Pts',(10.3559140724569,-27.2388808356861,1.73955302416723));
#40497=CARTESIAN_POINT('Ctrl Pts',(10.3559140653568,-26.421010256864,1.73955306643568));
#40498=CARTESIAN_POINT('Ctrl Pts',(10.4053763093799,-26.4073475080301,1.44509424338123));
#40499=CARTESIAN_POINT('Ctrl Pts',(10.4422574745547,-26.3935825359074,1.14865779515576));
#40500=CARTESIAN_POINT('Ctrl Pts',(10.5150042598825,-26.3522195855432,0.253998944556693));
#40501=CARTESIAN_POINT('Ctrl Pts',(10.5123763900469,-26.3247747687406,-0.346127364410621));
#40502=CARTESIAN_POINT('Ctrl Pts',(10.4169392019792,-26.2766726747831,-1.40487089015339));
#40503=CARTESIAN_POINT('Ctrl Pts',(10.3447016192798,-26.2559126398823,-1.86371609433252));
#40504=CARTESIAN_POINT('Ctrl Pts',(10.1631875152453,-26.2189761033502,-2.66635328187233));
#40505=CARTESIAN_POINT('Ctrl Pts',(10.0661264941496,-26.2028294217224,-3.01212785376631));
#40506=CARTESIAN_POINT('Ctrl Pts',(9.86067987055812,-26.1734270709244,-3.62201909199679));
#40507=CARTESIAN_POINT('Ctrl Pts',(9.7588780768272,-26.1603165689332,-3.88797195504891));
#40508=CARTESIAN_POINT('Ctrl Pts',(9.38725267733539,-26.1169778131602,-4.7519034130016));
#40509=CARTESIAN_POINT('Ctrl Pts',(9.07223249432078,-26.0869071754513,-5.32876508686101));
#40510=CARTESIAN_POINT('Ctrl Pts',(8.44117890084041,-26.0358766706685,-6.26425055801145));
#40511=CARTESIAN_POINT('Ctrl Pts',(8.15075011012007,-26.0147471347025,-6.63774153321893));
#40512=CARTESIAN_POINT('Ctrl Pts',(7.59423778360497,-25.9772077629551,-7.26158509250741));
#40513=CARTESIAN_POINT('Ctrl Pts',(7.33841597607909,-25.9608256695678,-7.52002076294703));
#40514=CARTESIAN_POINT('Ctrl Pts',(6.83157823214244,-25.9294566036194,-7.98149458489889));
#40515=CARTESIAN_POINT('Ctrl Pts',(6.58360070608352,-25.9146022781673,-8.18724107263935));
#40516=CARTESIAN_POINT('Ctrl Pts',(5.88210965424615,-25.8741070383352,-8.71675867788197));
#40517=CARTESIAN_POINT('Ctrl Pts',(5.41166455579838,-25.848602124492,-9.01637443596638));
#40518=CARTESIAN_POINT('Ctrl Pts',(4.51626111574609,-25.8027121228259,-9.49120096410001));
#40519=CARTESIAN_POINT('Ctrl Pts',(4.09932026913625,-25.782266567676,-9.67858920945322));
#40520=CARTESIAN_POINT('Ctrl Pts',(3.31555205797358,-25.7447277412708,-9.97108141040827));
#40521=CARTESIAN_POINT('Ctrl Pts',(2.95266192269231,-25.7276555657732,-10.0844996688866));
#40522=CARTESIAN_POINT('Ctrl Pts',(1.96335650260526,-25.6810310275951,-10.3357061868763));
#40523=CARTESIAN_POINT('Ctrl Pts',(1.32915926414281,-25.6513325826279,-10.4362320760073));
#40524=CARTESIAN_POINT('Ctrl Pts',(0.155471184914087,-25.5975072837113,
-10.51349280556));
#40525=CARTESIAN_POINT('Ctrl Pts',(-0.380732389865649,-25.57332580318,-10.5077478743005));
#40526=CARTESIAN_POINT('Ctrl Pts',(-1.51243151051676,-25.5223017337623,
-10.4088524806023));
#40527=CARTESIAN_POINT('Ctrl Pts',(-2.105094063499,-25.4955435251842,-10.3053495809229));
#40528=CARTESIAN_POINT('Ctrl Pts',(-2.99324982973951,-25.4535058446851,
-10.0703866737259));
#40529=CARTESIAN_POINT('Ctrl Pts',(-3.29697789022645,-25.4388323356821,
-9.97507727961022));
#40530=CARTESIAN_POINT('Ctrl Pts',(-4.1310470222125,-25.3979282388972,-9.67108410550937));
#40531=CARTESIAN_POINT('Ctrl Pts',(-4.64944294220166,-25.3718399981342,
-9.4328216758454));
#40532=CARTESIAN_POINT('Ctrl Pts',(-5.54624320751089,-25.3252688460578,
-8.92866454615409));
#40533=CARTESIAN_POINT('Ctrl Pts',(-5.93133526126242,-25.3047136898339,
-8.67762246063726));
#40534=CARTESIAN_POINT('Ctrl Pts',(-6.59647417843472,-25.2674082686937,
-8.17899596633479));
#40535=CARTESIAN_POINT('Ctrl Pts',(-6.8821083588964,-25.2506817614338,-7.94015285595226));
#40536=CARTESIAN_POINT('Ctrl Pts',(-7.3612417254224,-25.2207805952289,-7.49419227461852));
#40537=CARTESIAN_POINT('Ctrl Pts',(-7.56016532418387,-25.2077715320452,
-7.29346935868841));
#40538=CARTESIAN_POINT('Ctrl Pts',(-8.19096809570171,-25.164687907134,-6.60338968624071));
#40539=CARTESIAN_POINT('Ctrl Pts',(-8.58535441284443,-25.1347624597448,
-6.08181250940848));
#40540=CARTESIAN_POINT('Ctrl Pts',(-9.17532162892297,-25.0840582931718,
-5.12873073611511));
#40541=CARTESIAN_POINT('Ctrl Pts',(-9.39493501539029,-25.0631084905745,
-4.71440412229259));
#40542=CARTESIAN_POINT('Ctrl Pts',(-9.72579195387837,-25.0267227414275,
-3.97454108686022));
#40543=CARTESIAN_POINT('Ctrl Pts',(-9.85008604033848,-25.0113263559998,
-3.65565422511408));
#40544=CARTESIAN_POINT('Ctrl Pts',(-10.0475090082611,-24.9829011584856,
-3.06547160656759));
#40545=CARTESIAN_POINT('Ctrl Pts',(-10.1257431666508,-24.9699953280803,
-2.79622534657591));
#40546=CARTESIAN_POINT('Ctrl Pts',(-10.3498013354513,-24.9270425516554,
-1.89143472476857));
#40547=CARTESIAN_POINT('Ctrl Pts',(-10.4472378754441,-24.8971384918907,
-1.24546120469556));
#40548=CARTESIAN_POINT('Ctrl Pts',(-10.5105315661798,-24.8465673575754,
-0.129494179720476));
#40549=CARTESIAN_POINT('Ctrl Pts',(-10.5059298138899,-24.8257262199787,
0.336876526799625));
#40550=CARTESIAN_POINT('Ctrl Pts',(-10.4433458394034,-24.7889144151198,
1.15454288161165));
#40551=CARTESIAN_POINT('Ctrl Pts',(-10.3984689036257,-24.7729762833458,
1.50608188596581));
#40552=CARTESIAN_POINT('Ctrl Pts',(-10.2227949989665,-24.7275317307321,
2.4850893482032));
#40553=CARTESIAN_POINT('Ctrl Pts',(-10.0522379450659,-24.6978492270761,
3.10382547311552));
#40554=CARTESIAN_POINT('Ctrl Pts',(-9.63637208949906,-24.6438914559049,
4.20732917911189));
#40555=CARTESIAN_POINT('Ctrl Pts',(-9.40784979141307,-24.6195662675661,
4.69613336652643));
#40556=CARTESIAN_POINT('Ctrl Pts',(-8.85489998518067,-24.5690808561733,
5.67489077709454));
#40557=CARTESIAN_POINT('Ctrl Pts',(-8.5248765942037,-24.5429938150063,6.15955437490175));
#40558=CARTESIAN_POINT('Ctrl Pts',(-7.96308858724984,-24.5022015509437,
6.85231412771111));
#40559=CARTESIAN_POINT('Ctrl Pts',(-7.7596548887701,-24.488068459494,7.08186008694194));
#40560=CARTESIAN_POINT('Ctrl Pts',(-7.13008574280455,-24.446348251407,7.73249176946044));
#40561=CARTESIAN_POINT('Ctrl Pts',(-6.67764566236236,-24.4189126050422,
8.12641565994594));
#40562=CARTESIAN_POINT('Ctrl Pts',(-5.81990455958426,-24.3708457351095,
8.75296769942309));
#40563=CARTESIAN_POINT('Ctrl Pts',(-5.42802938843548,-24.3501112091167,
9.00123515811852));
#40564=CARTESIAN_POINT('Ctrl Pts',(-4.70445600895737,-24.313133073147,9.39515960325234));
#40565=CARTESIAN_POINT('Ctrl Pts',(-4.37921949755164,-24.2969184627326,
9.55109226122527));
#40566=CARTESIAN_POINT('Ctrl Pts',(-3.45484554077471,-24.2511530434077,
9.93711692767386));
#40567=CARTESIAN_POINT('Ctrl Pts',(-2.84168985470582,-24.2214319510062,
10.1295144453064));
#40568=CARTESIAN_POINT('Ctrl Pts',(-1.68852707966416,-24.167453513004,10.3783310276351));
#40569=CARTESIAN_POINT('Ctrl Pts',(-1.15427463222685,-24.1431446261589,
10.4512462941115));
#40570=CARTESIAN_POINT('Ctrl Pts',(-0.0313600116869125,-24.0926269555234,
10.5173154052712));
#40571=CARTESIAN_POINT('Ctrl Pts',(0.555901389045456,-24.0664924976876,
10.5026602528213));
#40572=CARTESIAN_POINT('Ctrl Pts',(1.44408451207068,-24.0256293279911,10.4057621242859));
#40573=CARTESIAN_POINT('Ctrl Pts',(1.74768954867303,-24.0114752109939,10.3590947597181));
#40574=CARTESIAN_POINT('Ctrl Pts',(2.63628317027525,-23.9697254489966,10.1823275246356));
#40575=CARTESIAN_POINT('Ctrl Pts',(3.21269362732594,-23.9422821578989,10.0154088227914));
#40576=CARTESIAN_POINT('Ctrl Pts',(4.20465038560577,-23.8941865287022,9.63364391806447));
#40577=CARTESIAN_POINT('Ctrl Pts',(4.62605489440489,-23.873431323799,9.43852747246173));
#40578=CARTESIAN_POINT('Ctrl Pts',(5.34843304860398,-23.8364869856283,9.04401972794437));
#40579=CARTESIAN_POINT('Ctrl Pts',(5.65463777661911,-23.8203275156975,8.8557945456203));
#40580=CARTESIAN_POINT('Ctrl Pts',(6.18508999708405,-23.7909147123274,8.49097506618665));
#40581=CARTESIAN_POINT('Ctrl Pts',(6.41292653670309,-23.7778069954154,8.32023836861591));
#40582=CARTESIAN_POINT('Ctrl Pts',(7.14183446102848,-23.7344772695802,7.72626177473927));
#40583=CARTESIAN_POINT('Ctrl Pts',(7.61022803695759,-23.7044126029548,7.2653555028247));
#40584=CARTESIAN_POINT('Ctrl Pts',(8.33687987902412,-23.6533943336693,6.40239276922271));
#40585=CARTESIAN_POINT('Ctrl Pts',(8.6164470357158,-23.6322710425749,6.02088394807754));
#40586=CARTESIAN_POINT('Ctrl Pts',(9.064094517327,-23.5947246656876,5.31464763599177));
#40587=CARTESIAN_POINT('Ctrl Pts',(9.2427159250987,-23.5783290937117,4.99754809726775));
#40588=CARTESIAN_POINT('Ctrl Pts',(9.5477499637454,-23.5469517252478,4.38350415411119));
#40589=CARTESIAN_POINT('Ctrl Pts',(9.67763823138923,-23.5321031086549,4.08875946811593));
#40590=CARTESIAN_POINT('Ctrl Pts',(9.99473535962366,-23.4916068255762,3.26902449295443));
#40591=CARTESIAN_POINT('Ctrl Pts',(10.1540425457154,-23.4660951502127,2.73435576359926));
#40592=CARTESIAN_POINT('Ctrl Pts',(10.3020404719139,-23.4339572630673,2.04017106286942));
#40593=CARTESIAN_POINT('Ctrl Pts',(10.3306207529291,-23.427063885569,1.89012929749398));
#40594=CARTESIAN_POINT('Ctrl Pts',(10.3559140377345,-23.4201872127662,1.73955323087672));
#40595=CARTESIAN_POINT('Origin',(0.,-20.,0.));
#40596=CARTESIAN_POINT('',(10.3559140572458,-20.4205078998763,1.73955311472209));
#40597=CARTESIAN_POINT('',(10.355914065439,-21.2383993725198,1.73955306594593));
#40598=CARTESIAN_POINT('',(10.355914065439,-20.,1.73955306594593));
#40599=CARTESIAN_POINT('',(7.93381306740072,-20.,-6.87936125025729));
#40600=CARTESIAN_POINT('Ctrl Pts',(10.3559140572458,-20.4205078998763,1.73955311472209));
#40601=CARTESIAN_POINT('Ctrl Pts',(10.4511075586512,-20.3940337853284,1.17284680893575));
#40602=CARTESIAN_POINT('Ctrl Pts',(10.4996412156828,-20.3677228408922,0.599170819368804));
#40603=CARTESIAN_POINT('Ctrl Pts',(10.5020506634867,-20.3206270227268,-0.441750604526287));
#40604=CARTESIAN_POINT('Ctrl Pts',(10.4721013615195,-20.2997771298122,-0.907363802500196));
#40605=CARTESIAN_POINT('Ctrl Pts',(10.3687453289844,-20.2641925554499,-1.69313568641755));
#40606=CARTESIAN_POINT('Ctrl Pts',(10.3110983543044,-20.2495054010901,-2.0146550712014));
#40607=CARTESIAN_POINT('Ctrl Pts',(10.1851156530754,-20.2236232764559,-2.56754856983621));
#40608=CARTESIAN_POINT('Ctrl Pts',(10.1236181694273,-20.2125498532238,-2.80022127884439));
#40609=CARTESIAN_POINT('Ctrl Pts',(9.86137790754711,-20.170624768431,-3.67022565940672));
#40610=CARTESIAN_POINT('Ctrl Pts',(9.60796262449235,-20.1397884991224,-4.2900376910404));
#40611=CARTESIAN_POINT('Ctrl Pts',(8.92131961002248,-20.0726190186162,-5.59781065982524));
#40612=CARTESIAN_POINT('Ctrl Pts',(8.4637606257779,-20.0367812230352,-6.26818461470371));
#40613=CARTESIAN_POINT('Ctrl Pts',(7.93381306740072,-20.,-6.87936125025729));
#40614=CARTESIAN_POINT('',(-7.93387242656103,-20.0000000365693,-6.87929279207206));
#40615=CARTESIAN_POINT('Origin',(0.,-20.,0.));
#40616=CARTESIAN_POINT('Ctrl Pts',(-7.93387242656103,-20.0000000365693,
-6.87929279207206));
#40617=CARTESIAN_POINT('Ctrl Pts',(-7.76761933943708,-20.0115427600485,
-7.07103209197269));
#40618=CARTESIAN_POINT('Ctrl Pts',(-7.59438520903055,-20.0230854835278,
-7.25677295860134));
#40619=CARTESIAN_POINT('Ctrl Pts',(-7.41462834869705,-20.034628207007,-7.4360128732203));
#40620=CARTESIAN_POINT('Ctrl Pts',(-7.23490292970705,-20.0461689115439,
-7.61522143691495));
#40621=CARTESIAN_POINT('Ctrl Pts',(-7.04865725581925,-20.0577096160809,
-7.78793112142728));
#40622=CARTESIAN_POINT('Ctrl Pts',(-6.85638681915036,-20.0692503206178,
-7.95367592916516));
#40623=CARTESIAN_POINT('Ctrl Pts',(-6.66413668086264,-20.080789806779,-8.11940323888648));
#40624=CARTESIAN_POINT('Ctrl Pts',(-6.46586326115029,-20.0923292929403,
-8.27816695779237));
#40625=CARTESIAN_POINT('Ctrl Pts',(-6.26209628867734,-20.1038687791016,
-8.42954038316049));
#40626=CARTESIAN_POINT('Ctrl Pts',(-6.05831348529575,-20.1154091617798,
-8.58092556891764));
#40627=CARTESIAN_POINT('Ctrl Pts',(-5.84903649881054,-20.126949544458,-8.72491914519595));
#40628=CARTESIAN_POINT('Ctrl Pts',(-5.63482633728949,-20.1384899271363,
-8.86113610935916));
#40629=CARTESIAN_POINT('Ctrl Pts',(-5.42061577914819,-20.1500303311821,
-8.99735332573452));
#40630=CARTESIAN_POINT('Ctrl Pts',(-5.20147226469043,-20.1615707352279,
-9.12579375361984));
#40631=CARTESIAN_POINT('Ctrl Pts',(-4.97798450545638,-20.1731111392737,
-9.24611655039218));
#40632=CARTESIAN_POINT('Ctrl Pts',(-4.75444854472634,-20.1846540323361,
-9.36646529820017));
#40633=CARTESIAN_POINT('Ctrl Pts',(-4.52656671290687,-20.1961969253985,
-9.47869278418477));
#40634=CARTESIAN_POINT('Ctrl Pts',(-4.29495217795627,-20.2077398184608,
-9.58250420240288));
#40635=CARTESIAN_POINT('Ctrl Pts',(-4.17906943469033,-20.2135150264528,
-9.63444374034253));
#40636=CARTESIAN_POINT('Ctrl Pts',(-4.06225265218799,-20.2192902344447,
-9.6842772535272));
#40637=CARTESIAN_POINT('Ctrl Pts',(-3.94458058590528,-20.2250654424367,
-9.73197230787774));
#40638=CARTESIAN_POINT('Ctrl Pts',(-3.70889539637858,-20.236632597099,-9.8275006544021));
#40639=CARTESIAN_POINT('Ctrl Pts',(-3.46970190359019,-20.2481997517614,
-9.91447815568018));
#40640=CARTESIAN_POINT('Ctrl Pts',(-3.227639342775,-20.2597669064238,-9.99266457322425));
#40641=CARTESIAN_POINT('Ctrl Pts',(-2.98561909575511,-20.2713320390874,
-10.0708373233757));
#40642=CARTESIAN_POINT('Ctrl Pts',(-2.74073104518588,-20.282897171751,-10.1402219724847));
#40643=CARTESIAN_POINT('Ctrl Pts',(-2.49363094408252,-20.2944623044145,
-10.2006277117986));
#40644=CARTESIAN_POINT('Ctrl Pts',(-2.24655838679567,-20.306026147933,-10.2610267177903));
#40645=CARTESIAN_POINT('Ctrl Pts',(-1.99727454010465,-20.3175899914514,
-10.3124487466889));
#40646=CARTESIAN_POINT('Ctrl Pts',(-1.74644781609206,-20.3291538349698,
-10.3547535473167));
#40647=CARTESIAN_POINT('Ctrl Pts',(-1.49560122773008,-20.3407185942927,
-10.3970616982946));
#40648=CARTESIAN_POINT('Ctrl Pts',(-1.24321179031955,-20.3522833536156,
-10.4302511288727));
#40649=CARTESIAN_POINT('Ctrl Pts',(-0.989956899476713,-20.3638481129385,
-10.4542329387277));
#40650=CARTESIAN_POINT('Ctrl Pts',(-0.736706570407378,-20.3754126639502,
-10.4782143166084));
#40651=CARTESIAN_POINT('Ctrl Pts',(-0.482591094877707,-20.386977214962,
-10.4929883812208));
#40652=CARTESIAN_POINT('Ctrl Pts',(-0.228292540303652,-20.3985417659737,
-10.4985181581041));
#40653=CARTESIAN_POINT('Ctrl Pts',(0.0260656621990141,-20.4101090295511,
-10.5040492320444));
#40654=CARTESIAN_POINT('Ctrl Pts',(0.280606752688652,-20.4216762931284,
-10.5003316777243));
#40655=CARTESIAN_POINT('Ctrl Pts',(0.534647621022751,-20.4332435567058,
-10.4873806511128));
#40656=CARTESIAN_POINT('Ctrl Pts',(0.754810692836675,-20.4432682598111,
-10.4761567176542));
#40657=CARTESIAN_POINT('Ctrl Pts',(0.974597946320386,-20.4532929629165,
-10.4579986016713));
#40658=CARTESIAN_POINT('Ctrl Pts',(1.19356681527101,-20.4633176660218,-10.4329477741185));
#40659=CARTESIAN_POINT('Ctrl Pts',(1.44621574302689,-20.4748842896372,-10.4040438264891));
#40660=CARTESIAN_POINT('Ctrl Pts',(1.69785355141683,-20.4864509132526,-10.3659536780285));
#40661=CARTESIAN_POINT('Ctrl Pts',(1.94780404330222,-20.4980175368679,-10.3187722335991));
#40662=CARTESIAN_POINT('Ctrl Pts',(2.19771061531791,-20.5095821280624,-10.271599079623));
#40663=CARTESIAN_POINT('Ctrl Pts',(2.44593019076294,-20.5211467192569,-10.2153378699943));
#40664=CARTESIAN_POINT('Ctrl Pts',(2.69179571929448,-20.5327113104513,-10.1501348171139));
#40665=CARTESIAN_POINT('Ctrl Pts',(2.93763365212993,-20.5442746036479,-10.0849390825577));
#40666=CARTESIAN_POINT('Ctrl Pts',(3.18111779808646,-20.5558378968444,-10.0108035796106));
#40667=CARTESIAN_POINT('Ctrl Pts',(3.42159418211181,-20.567401190041,-9.92792497216506));
#40668=CARTESIAN_POINT('Ctrl Pts',(3.66208940860482,-20.5789653892765,-9.84503987078675));
#40669=CARTESIAN_POINT('Ctrl Pts',(3.89957613936932,-20.5905295885121,-9.7534103830688));
#40670=CARTESIAN_POINT('Ctrl Pts',(4.13341708260761,-20.6020937877476,-9.65328256196863));
#40671=CARTESIAN_POINT('Ctrl Pts',(4.36725372089671,-20.6136577740893,-9.55315658419485));
#40672=CARTESIAN_POINT('Ctrl Pts',(4.59744445206855,-20.6252217604311,-9.44453269662927));
#40673=CARTESIAN_POINT('Ctrl Pts',(4.82337272867542,-20.6367857467728,-9.32770478307875));
#40674=CARTESIAN_POINT('Ctrl Pts',(5.049353932526,-20.6483524421598,-9.21084950075641));
#40675=CARTESIAN_POINT('Ctrl Pts',(5.27107043963594,-20.6599191375467,-9.08578647774354));
#40676=CARTESIAN_POINT('Ctrl Pts',(5.48792973200312,-20.6714858329337,-8.95285587154156));
#40677=CARTESIAN_POINT('Ctrl Pts',(5.67594100123841,-20.6815138518248,-8.83760855278735));
#40678=CARTESIAN_POINT('Ctrl Pts',(5.86030167021098,-20.6915418707158,-8.71644839631923));
#40679=CARTESIAN_POINT('Ctrl Pts',(6.04064259344008,-20.7015698896069,-8.58962386011853));
#40680=CARTESIAN_POINT('Ctrl Pts',(6.24866971656362,-20.7131374244913,-8.44332903731897));
#40681=CARTESIAN_POINT('Ctrl Pts',(6.45141193053673,-20.7247049593757,-8.2894509307573));
#40682=CARTESIAN_POINT('Ctrl Pts',(6.64832085415769,-20.7362724942601,-8.1283965712908));
#40683=CARTESIAN_POINT('Ctrl Pts',(6.84519539190618,-20.7478380091254,-7.96737033647484));
#40684=CARTESIAN_POINT('Ctrl Pts',(7.03623845868885,-20.7594035239908,-7.79917052559365));
#40685=CARTESIAN_POINT('Ctrl Pts',(7.22093426151812,-20.7709690388561,-7.624244840693));
#40686=CARTESIAN_POINT('Ctrl Pts',(7.4056094914013,-20.7825332654588,-7.4493386404619));
#40687=CARTESIAN_POINT('Ctrl Pts',(7.58393866813121,-20.7940974920614,-7.26770825235433));
#40688=CARTESIAN_POINT('Ctrl Pts',(7.75544162581868,-20.805661718664,-7.07983941827206));
#40689=CARTESIAN_POINT('Ctrl Pts',(7.92695814427787,-20.8172268596523,-6.89195572936509));
#40690=CARTESIAN_POINT('Ctrl Pts',(8.09164717607218,-20.8287920006405,-6.69783281100001));
#40691=CARTESIAN_POINT('Ctrl Pts',(8.24906684102578,-20.8403571416288,-6.49799178610508));
#40692=CARTESIAN_POINT('Ctrl Pts',(8.40648365211932,-20.8519220729527,-6.29815438412675));
#40693=CARTESIAN_POINT('Ctrl Pts',(8.55663119010718,-20.8634870042766,-6.09259930154301));
#40694=CARTESIAN_POINT('Ctrl Pts',(8.69910868029778,-20.8750519356005,-5.88187973086563));
#40695=CARTESIAN_POINT('Ctrl Pts',(8.84161952783095,-20.8866195745477,-5.67111082576427));
#40696=CARTESIAN_POINT('Ctrl Pts',(8.97645658274871,-20.8981872134949,-5.45517524491679));
#40697=CARTESIAN_POINT('Ctrl Pts',(9.10326231471628,-20.9097548524421,-5.23465531142849));
#40698=CARTESIAN_POINT('Ctrl Pts',(9.21312918916514,-20.9197772726921,-5.04359268775918));
#40699=CARTESIAN_POINT('Ctrl Pts',(9.31696772742072,-20.929799692942,-4.84908921829048));
#40700=CARTESIAN_POINT('Ctrl Pts',(9.41457305225478,-20.939822113192,-4.65153901883646));
#40701=CARTESIAN_POINT('Ctrl Pts',(9.52721930290881,-20.9513889827819,-4.42354644443251));
#40702=CARTESIAN_POINT('Ctrl Pts',(9.63159720442441,-20.9629558523718,-4.19142462929392));
#40703=CARTESIAN_POINT('Ctrl Pts',(9.72742002242571,-20.9745227219618,-3.95579330947807));
#40704=CARTESIAN_POINT('Ctrl Pts',(9.82322603763173,-20.9860875632692,-3.72020330826367));
#40705=CARTESIAN_POINT('Ctrl Pts',(9.9104798598109,-20.9976524045767,-3.48110528720753));
#40706=CARTESIAN_POINT('Ctrl Pts',(9.98894283068408,-21.0092172458841,-3.239139102497));
#40707=CARTESIAN_POINT('Ctrl Pts',(10.0673970183146,-21.0207807926089,-2.99720000378244));
#40708=CARTESIAN_POINT('Ctrl Pts',(10.1370622341292,-21.0323443393336,-2.75239364572877));
#40709=CARTESIAN_POINT('Ctrl Pts',(10.1977493055541,-21.0439078860583,-2.50537623942399));
#40710=CARTESIAN_POINT('Ctrl Pts',(10.2584411501937,-21.0554723422896,-2.25833940448198));
#40711=CARTESIAN_POINT('Ctrl Pts',(10.3101533700907,-21.0670367985209,-2.00909144186774));
#40712=CARTESIAN_POINT('Ctrl Pts',(10.3527473408365,-21.0786012547522,-1.7583013100156));
#40713=CARTESIAN_POINT('Ctrl Pts',(10.3953405331329,-21.0901654996309,-1.50751576161611));
#40714=CARTESIAN_POINT('Ctrl Pts',(10.4288157650271,-21.1017297445096,-1.25518837362847));
#40715=CARTESIAN_POINT('Ctrl Pts',(10.4530858517841,-21.1132939893884,-1.00199659442136));
#40716=CARTESIAN_POINT('Ctrl Pts',(10.477361625521,-21.1248609440073,-0.748745487178918));
#40717=CARTESIAN_POINT('Ctrl Pts',(10.492427915911,-21.1364278986261,-0.494629859558366));
#40718=CARTESIAN_POINT('Ctrl Pts',(10.4982494496924,-21.147994853245,-0.240332045374238));
#40719=CARTESIAN_POINT('Ctrl Pts',(10.5032956851473,-21.1580213477557,-0.0199010225154512));
#40720=CARTESIAN_POINT('Ctrl Pts',(10.5013963984425,-21.1680478422664,0.200666716014797));
#40721=CARTESIAN_POINT('Ctrl Pts',(10.4925603111451,-21.1780743367771,0.420926498313265));
#40722=CARTESIAN_POINT('Ctrl Pts',(10.4823664077128,-21.1896415738773,0.675032968203946));
#40723=CARTESIAN_POINT('Ctrl Pts',(10.4629357454992,-21.2012088109776,0.928808297393872));
#40724=CARTESIAN_POINT('Ctrl Pts',(10.4343131459793,-21.2127760480778,1.18157106076805));
#40725=CARTESIAN_POINT('Ctrl Pts',(10.413178564243,-21.2213171562251,1.36820803197274));
#40726=CARTESIAN_POINT('Ctrl Pts',(10.3870334654684,-21.2298582643724,1.5542929328799));
#40727=CARTESIAN_POINT('Ctrl Pts',(10.355914065439,-21.2383993725198,1.73955306594593));
#40728=CARTESIAN_POINT('Origin',(0.,-20.,0.));
#40729=CARTESIAN_POINT('',(-10.5009999965284,-22.6589303284762,0.000270018945713324));
#40730=CARTESIAN_POINT('Ctrl Pts',(10.355914065439,-21.2383993725198,1.73955306594593));
#40731=CARTESIAN_POINT('Ctrl Pts',(10.3137801598842,-21.249963549325,1.99038479606632));
#40732=CARTESIAN_POINT('Ctrl Pts',(10.262525630829,-21.2615277261302,2.23970409686379));
#40733=CARTESIAN_POINT('Ctrl Pts',(10.2022850825147,-21.2730919029355,2.48684138921193));
#40734=CARTESIAN_POINT('Ctrl Pts',(10.1401064651179,-21.2850281243877,2.74192962422017));
#40735=CARTESIAN_POINT('Ctrl Pts',(10.0683541050816,-21.2969643458399,2.99469282093897));
#40736=CARTESIAN_POINT('Ctrl Pts',(9.98723265985342,-21.3089005672922,3.24440823540398));
#40737=CARTESIAN_POINT('Ctrl Pts',(9.90863688274792,-21.3204651615632,3.48634890842686));
#40738=CARTESIAN_POINT('Ctrl Pts',(9.8212467005171,-21.3320297558341,3.72542843874294));
#40739=CARTESIAN_POINT('Ctrl Pts',(9.72529859813282,-21.3435943501051,3.96100595520327));
#40740=CARTESIAN_POINT('Ctrl Pts',(9.62472557048125,-21.355716385148,4.20793886464386));
#40741=CARTESIAN_POINT('Ctrl Pts',(9.51474940816849,-21.3678384201908,4.45102352994098));
#40742=CARTESIAN_POINT('Ctrl Pts',(9.39569915454623,-21.3799604552337,4.68954564934165));
#40743=CARTESIAN_POINT('Ctrl Pts',(9.27664890092398,-21.3920824902765,4.92806776874232));
#40744=CARTESIAN_POINT('Ctrl Pts',(9.14852472029361,-21.4042045253194,5.16202703322294));
#40745=CARTESIAN_POINT('Ctrl Pts',(9.01171144400528,-21.4163265603622,5.3907381544631));
#40746=CARTESIAN_POINT('Ctrl Pts',(8.88116158188507,-21.4278936395697,5.60897870942459));
#40747=CARTESIAN_POINT('Ctrl Pts',(8.74265991882838,-21.4394607187771,5.82250848322716));
#40748=CARTESIAN_POINT('Ctrl Pts',(8.59657188523118,-21.4510277979846,6.03075060187808));
#40749=CARTESIAN_POINT('Ctrl Pts',(8.4505094356669,-21.4625928514783,6.2389562516062));
#40750=CARTESIAN_POINT('Ctrl Pts',(8.29686342668248,-21.4741579049721,6.44187586825201));
#40751=CARTESIAN_POINT('Ctrl Pts',(8.13604225364843,-21.4857229584658,6.63896207602118));
#40752=CARTESIAN_POINT('Ctrl Pts',(7.97523905559419,-21.4972867193337,6.83602625546821));
#40753=CARTESIAN_POINT('Ctrl Pts',(7.80726246971846,-21.5088504802016,7.02725811347665));
#40754=CARTESIAN_POINT('Ctrl Pts',(7.63256145618795,-21.5204142410695,7.21214299757805));
#40755=CARTESIAN_POINT('Ctrl Pts',(7.45784667973633,-21.5319789129288,7.39704244688444));
#40756=CARTESIAN_POINT('Ctrl Pts',(7.27640660479399,-21.5435435847882,7.57559371963092));
#40757=CARTESIAN_POINT('Ctrl Pts',(7.08872830055417,-21.5551082566475,7.74731773460482));
#40758=CARTESIAN_POINT('Ctrl Pts',(6.90105341810014,-21.5666727176576,7.9190386186745));
#40759=CARTESIAN_POINT('Ctrl Pts',(6.7071407393271,-21.5782371786677,8.08393230839117));
#40760=CARTESIAN_POINT('Ctrl Pts',(6.50751234785376,-21.5898016396778,8.24155835036863));
#40761=CARTESIAN_POINT('Ctrl Pts',(6.30783719252314,-21.6013688097154,8.39922131696226));
#40762=CARTESIAN_POINT('Ctrl Pts',(6.10244386533026,-21.612935979753,8.54961306089774));
#40763=CARTESIAN_POINT('Ctrl Pts',(5.89188669093887,-21.6245031497906,8.69233410662162));
#40764=CARTESIAN_POINT('Ctrl Pts',(5.70939778698396,-21.6345283611761,8.81602975974163));
#40765=CARTESIAN_POINT('Ctrl Pts',(5.52303059208191,-21.6445535725617,8.93396407346109));
#40766=CARTESIAN_POINT('Ctrl Pts',(5.3331633740482,-21.6545787839473,9.04590346099885));
#40767=CARTESIAN_POINT('Ctrl Pts',(5.11409401130845,-21.6661459027596,9.17505946037215));
#40768=CARTESIAN_POINT('Ctrl Pts',(4.89029674129765,-21.677713021572,9.29627375453589));
#40769=CARTESIAN_POINT('Ctrl Pts',(4.66236849914987,-21.6892801403843,9.40921468445348));
#40770=CARTESIAN_POINT('Ctrl Pts',(4.4344801664234,-21.7008452338355,9.52213583881753));
#40771=CARTESIAN_POINT('Ctrl Pts',(4.20246255342235,-21.7124103272867,9.62678639796797));
#40772=CARTESIAN_POINT('Ctrl Pts',(3.96693620500328,-21.7239754207378,9.72288116483145));
#40773=CARTESIAN_POINT('Ctrl Pts',(3.73143617643087,-21.7355392218007,9.81896519319563));
#40774=CARTESIAN_POINT('Ctrl Pts',(3.49242845155076,-21.7471030228636,9.90649523377258));
#40775=CARTESIAN_POINT('Ctrl Pts',(3.25055353409967,-21.7586668239265,9.98523423470637));
#40776=CARTESIAN_POINT('Ctrl Pts',(3.00865956023713,-21.7702315360576,10.0639794391887));
#40777=CARTESIAN_POINT('Ctrl Pts',(2.76389820463271,-21.7817962481888,10.1339321311693));
#40778=CARTESIAN_POINT('Ctrl Pts',(2.51692641074983,-21.7933609603199,10.1949047294651));
#40779=CARTESIAN_POINT('Ctrl Pts',(2.26995912005407,-21.8049254615846,10.2558762160104));
#40780=CARTESIAN_POINT('Ctrl Pts',(2.02078174091657,-21.8164899628492,10.3078678717852));
#40781=CARTESIAN_POINT('Ctrl Pts',(1.77006347660718,-21.8280544641139,10.3507427892293));
#40782=CARTESIAN_POINT('Ctrl Pts',(1.51928648744899,-21.8396216740907,10.3936277491129));
#40783=CARTESIAN_POINT('Ctrl Pts',(1.26696816464985,-21.8511888840674,10.4273916553262));
#40784=CARTESIAN_POINT('Ctrl Pts',(1.01378641150786,-21.8627560940442,10.451949010201));
#40785=CARTESIAN_POINT('Ctrl Pts',(0.794361003023756,-21.8727810652069,
10.4732321696619));
#40786=CARTESIAN_POINT('Ctrl Pts',(0.574287290355624,-21.8828060363696,
10.4876009062648));
#40787=CARTESIAN_POINT('Ctrl Pts',(0.354009164658848,-21.8928310075323,
10.4950311343672));
#40788=CARTESIAN_POINT('Ctrl Pts',(0.0998454799983954,-21.9043981279682,
10.5036043603578));
#40789=CARTESIAN_POINT('Ctrl Pts',(-0.154669164764553,-21.9159652484041,
10.5029417501122));
#40790=CARTESIAN_POINT('Ctrl Pts',(-0.408851908986821,-21.92753236884,10.4930377449296));
#40791=CARTESIAN_POINT('Ctrl Pts',(-0.662990148560078,-21.9390974639982,
10.4831354738312));
#40792=CARTESIAN_POINT('Ctrl Pts',(-0.916796327124914,-21.9506625591565,
10.4639950486802));
#40793=CARTESIAN_POINT('Ctrl Pts',(-1.16958908724468,-21.9622276543147,
10.4356630056263));
#40794=CARTESIAN_POINT('Ctrl Pts',(-1.42235359973181,-21.9737914571631,
10.4073341284589));
#40795=CARTESIAN_POINT('Ctrl Pts',(-1.67410464488521,-21.9853552600116,
10.3698157149898));
#40796=CARTESIAN_POINT('Ctrl Pts',(-1.9241663796562,-21.99691906286,10.323206127139));
#40797=CARTESIAN_POINT('Ctrl Pts',(-2.17424781820299,-22.0084837768858,
10.2765928666557));
#40798=CARTESIAN_POINT('Ctrl Pts',(-2.42263940761389,-22.0200484909115,
10.220887047828));
#40799=CARTESIAN_POINT('Ctrl Pts',(-2.66867454355026,-22.0316132049373,
10.1562383381155));
#40800=CARTESIAN_POINT('Ctrl Pts',(-2.91470519460546,-22.0431777081542,
10.0915908068597));
#40801=CARTESIAN_POINT('Ctrl Pts',(-3.15837921079943,-22.0547422113712,
10.0180007828975));
#40802=CARTESIAN_POINT('Ctrl Pts',(-3.39904347241097,-22.0663067145882,
9.93566829522103));
#40803=CARTESIAN_POINT('Ctrl Pts',(-3.6397641056346,-22.0778739265982,9.85331652252478));
#40804=CARTESIAN_POINT('Ctrl Pts',(-3.87747331294342,-22.0894411386083,
9.76221828223451));
#40805=CARTESIAN_POINT('Ctrl Pts',(-4.11153493727735,-22.1010083506183,
9.66262290786243));
#40806=CARTESIAN_POINT('Ctrl Pts',(-4.31438921697679,-22.1110333107847,
9.57630654572003));
#40807=CARTESIAN_POINT('Ctrl Pts',(-4.51450390802682,-22.1210582709511,
9.48360864941968));
#40808=CARTESIAN_POINT('Ctrl Pts',(-4.71147772092378,-22.1310832311175,
9.38472049052282));
#40809=CARTESIAN_POINT('Ctrl Pts',(-4.93875220021531,-22.1426503403095,
9.27062027338817));
#40810=CARTESIAN_POINT('Ctrl Pts',(-5.16191511449861,-22.1542174495014,
9.14824246401068));
#40811=CARTESIAN_POINT('Ctrl Pts',(-5.38036420898964,-22.1657845586934,
9.01790895821328));
#40812=CARTESIAN_POINT('Ctrl Pts',(-5.59877505233851,-22.1773496424472,
8.88759827423379));
#40813=CARTESIAN_POINT('Ctrl Pts',(-5.81247348602248,-22.1889147262009,
8.74933481654849));
#40814=CARTESIAN_POINT('Ctrl Pts',(-6.02088350472526,-22.2004798099547,
8.60348550428995));
#40815=CARTESIAN_POINT('Ctrl Pts',(-6.22927023290093,-22.2120436012711,
8.45765249118719));
#40816=CARTESIAN_POINT('Ctrl Pts',(-6.43236949941675,-22.2236073925875,
8.30423547485258));
#40817=CARTESIAN_POINT('Ctrl Pts',(-6.62963494174465,-22.2351711839039,
8.14364424193484));
#40818=CARTESIAN_POINT('Ctrl Pts',(-6.82691592579408,-22.2467358862832,
7.98304035670358));
#40819=CARTESIAN_POINT('Ctrl Pts',(-7.01836195042591,-22.2583005886625,
7.81526129764087));
#40820=CARTESIAN_POINT('Ctrl Pts',(-7.20345931715591,-22.2698652910418,
7.64075747986283));
#40821=CARTESIAN_POINT('Ctrl Pts',(-7.38855330907376,-22.2814297825661,
7.46625684374865));
#40822=CARTESIAN_POINT('Ctrl Pts',(-7.56729867441535,-22.2929942740905,
7.28503188540077));
#40823=CARTESIAN_POINT('Ctrl Pts',(-7.73921765517788,-22.3045587656148,
7.09757078765566));
#40824=CARTESIAN_POINT('Ctrl Pts',(-7.91117690526097,-22.3161259659396,
6.91006578009324));
#40825=CARTESIAN_POINT('Ctrl Pts',(-8.07630638719474,-22.3276931662644,
6.71632191726792));
#40826=CARTESIAN_POINT('Ctrl Pts',(-8.23416683158492,-22.3392603665892,
6.51686255721469));
#40827=CARTESIAN_POINT('Ctrl Pts',(-8.37098088745965,-22.3492853959603,
6.34399566749777));
#40828=CARTESIAN_POINT('Ctrl Pts',(-8.50233549758968,-22.3593104253315,
6.16683632915167));
#40829=CARTESIAN_POINT('Ctrl Pts',(-8.6279698299386,-22.3693354547026,5.98574453294403));
#40830=CARTESIAN_POINT('Ctrl Pts',(-8.7729297269788,-22.3809025733261,5.776796487913));
#40831=CARTESIAN_POINT('Ctrl Pts',(-8.91031820995912,-22.3924696919496,
5.56254773761589));
#40832=CARTESIAN_POINT('Ctrl Pts',(-9.03976050121706,-22.4040368105731,
5.343569133139));
#40833=CARTESIAN_POINT('Ctrl Pts',(-9.16918012806939,-22.4156019038781,
5.12462887022624));
#40834=CARTESIAN_POINT('Ctrl Pts',(-9.29065619986459,-22.4271669971831,
4.9009606445605));
#40835=CARTESIAN_POINT('Ctrl Pts',(-9.40385853326217,-22.4387320904881,
4.67316227905604));
#40836=CARTESIAN_POINT('Ctrl Pts',(-9.51704821682695,-22.4502958914479,
4.44538936895653));
#40837=CARTESIAN_POINT('Ctrl Pts',(-9.62196588488816,-22.4618596924076,
4.2134874883438));
#40838=CARTESIAN_POINT('Ctrl Pts',(-9.71832789633379,-22.4734234933674,
3.97807791519226));
#40839=CARTESIAN_POINT('Ctrl Pts',(-9.81469750034251,-22.484988205463,3.74264979363137));
#40840=CARTESIAN_POINT('Ctrl Pts',(-9.90250999273814,-22.4965529175587,
3.50371368221689));
#40841=CARTESIAN_POINT('Ctrl Pts',(-9.98152985600637,-22.5081176296544,
3.26191090216357));
#40842=CARTESIAN_POINT('Ctrl Pts',(-10.060548278714,-22.5196821309211,3.02011253026216));
#40843=CARTESIAN_POINT('Ctrl Pts',(-10.1307743086362,-22.5312466321879,
2.77544785797645));
#40844=CARTESIAN_POINT('Ctrl Pts',(-10.1920220597857,-22.5428111334547,
2.52857416993089));
#40845=CARTESIAN_POINT('Ctrl Pts',(-10.253284157106,-22.5543783434954,2.28164265621764));
#40846=CARTESIAN_POINT('Ctrl Pts',(-10.3055637050415,-22.5659455535361,
2.03250136123242));
#40847=CARTESIAN_POINT('Ctrl Pts',(-10.3487254459157,-22.5775127635768,
1.78182003722534));
#40848=CARTESIAN_POINT('Ctrl Pts',(-10.3861324977168,-22.5875377351471,
1.56456167176555));
#40849=CARTESIAN_POINT('Ctrl Pts',(-10.4166917642207,-22.5975627067174,
1.34614685374224));
#40850=CARTESIAN_POINT('Ctrl Pts',(-10.4403464900633,-22.6075876782877,
1.12701648941934));
#40851=CARTESIAN_POINT('Ctrl Pts',(-10.4692474892472,-22.6198360424031,
0.859286204883308));
#40852=CARTESIAN_POINT('Ctrl Pts',(-10.4878466242685,-22.6320844065186,
0.590435506072792));
#40853=CARTESIAN_POINT('Ctrl Pts',(-10.496085593371,-22.644332770634,0.32122922754471));
#40854=CARTESIAN_POINT('Ctrl Pts',(-10.4993586516315,-22.6491986232481,
0.214282858074387));
#40855=CARTESIAN_POINT('Ctrl Pts',(-10.5009972449014,-22.6540644758621,
0.107280420198263));
#40856=CARTESIAN_POINT('Ctrl Pts',(-10.5009999965284,-22.6589303284762,
0.000270018945713879));
#40857=CARTESIAN_POINT('Ctrl Pts',(-10.5009999965872,-22.6588805488861,
0.000267724969670036));
#40858=CARTESIAN_POINT('Ctrl Pts',(-10.5010126771194,-22.6818006656778,
-0.497101904332627));
#40859=CARTESIAN_POINT('Ctrl Pts',(-10.4656892092644,-22.7046448522079,
-0.993853520664748));
#40860=CARTESIAN_POINT('Ctrl Pts',(-10.3242131605364,-22.7500807458748,
-1.98339130199445));
#40861=CARTESIAN_POINT('Ctrl Pts',(-10.2175600408328,-22.7726097978088,
-2.47481233318349));
#40862=CARTESIAN_POINT('Ctrl Pts',(-9.99242656851183,-22.8084782689233,
-3.24204137223171));
#40863=CARTESIAN_POINT('Ctrl Pts',(-9.89662109300719,-22.8218100622224,
-3.52367825448765));
#40864=CARTESIAN_POINT('Ctrl Pts',(-9.57874156277706,-22.8615515930728,
-4.34236563191908));
#40865=CARTESIAN_POINT('Ctrl Pts',(-9.32392563585833,-22.888417807518,-4.86547030910378));
#40866=CARTESIAN_POINT('Ctrl Pts',(-8.75263104549614,-22.9398753912165,
-5.82676945844352));
#40867=CARTESIAN_POINT('Ctrl Pts',(-8.44302268121886,-22.9643879426073,
-6.26699164878198));
#40868=CARTESIAN_POINT('Ctrl Pts',(-7.69346093331466,-23.0175828619016,
-7.17579645049292));
#40869=CARTESIAN_POINT('Ctrl Pts',(-7.24148335360625,-23.0460297043472,
-7.63166399727421));
#40870=CARTESIAN_POINT('Ctrl Pts',(-6.47325740482191,-23.0914459140182,
-8.27642591553376));
#40871=CARTESIAN_POINT('Ctrl Pts',(-6.18385667843293,-23.108087882826,-8.49483305557552));
#40872=CARTESIAN_POINT('Ctrl Pts',(-5.50052676811626,-23.1460926230776,
-8.95707975104865));
#40873=CARTESIAN_POINT('Ctrl Pts',(-5.10057640740971,-23.1674106662637,
-9.19071286829367));
#40874=CARTESIAN_POINT('Ctrl Pts',(-4.15101812912958,-23.2158562594999,
-9.66427110769821));
#40875=CARTESIAN_POINT('Ctrl Pts',(-3.59366149896661,-23.2427350604403,
-9.88507487774687));
#40876=CARTESIAN_POINT('Ctrl Pts',(-2.72749800666996,-23.28330497042,-10.1452141221778));
#40877=CARTESIAN_POINT('Ctrl Pts',(-2.43076105389523,-23.2970169167777,
-10.2203724046451));
#40878=CARTESIAN_POINT('Ctrl Pts',(-1.55943077684954,-23.337267736517,-10.4009665326054));
#40879=CARTESIAN_POINT('Ctrl Pts',(-0.978820817213086,-23.36426686629,-10.4715709498557));
#40880=CARTESIAN_POINT('Ctrl Pts',(0.143534307043352,-23.4159539037152,
-10.5138593771421));
#40881=CARTESIAN_POINT('Ctrl Pts',(0.683221821986221,-23.4405566447055,
-10.4926199329967));
#40882=CARTESIAN_POINT('Ctrl Pts',(1.85613040415187,-23.4938839262522,-10.3555490567668));
#40883=CARTESIAN_POINT('Ctrl Pts',(2.48519125001576,-23.522372779407,-10.2228382358753));
#40884=CARTESIAN_POINT('Ctrl Pts',(3.43950857927777,-23.5675979520273,-9.92816134190129));
#40885=CARTESIAN_POINT('Ctrl Pts',(3.77521664844392,-23.5840007523882,-9.80542356509557));
#40886=CARTESIAN_POINT('Ctrl Pts',(4.53170105575867,-23.6218580551176,-9.48422827044658));
#40887=CARTESIAN_POINT('Ctrl Pts',(4.94687736646116,-23.6432704977692,-9.27444418477801));
#40888=CARTESIAN_POINT('Ctrl Pts',(5.86248228431866,-23.6918487325796,-8.73277218301214));
#40889=CARTESIAN_POINT('Ctrl Pts',(6.35111776109031,-23.7187665439782,-8.38411192777041));
#40890=CARTESIAN_POINT('Ctrl Pts',(7.04173267828325,-23.759454305756,-7.79613710549295));
#40891=CARTESIAN_POINT('Ctrl Pts',(7.2672222328201,-23.7732481327237,-7.58638453490304));
#40892=CARTESIAN_POINT('Ctrl Pts',(7.89592170235234,-23.8137806611875,-6.94777403078112));
#40893=CARTESIAN_POINT('Ctrl Pts',(8.27269706695908,-23.8409873637394,-6.49458121508277));
#40894=CARTESIAN_POINT('Ctrl Pts',(8.917404410757,-23.8928046424922,-5.57136141121609));
#40895=CARTESIAN_POINT('Ctrl Pts',(9.19096995960149,-23.9173338174171,-5.10747143168864));
#40896=CARTESIAN_POINT('Ctrl Pts',(9.70990217882667,-23.9705419353012,-4.04958052614503));
#40897=CARTESIAN_POINT('Ctrl Pts',(9.93878643732868,-23.9989857837472,-3.44989966382878));
#40898=CARTESIAN_POINT('Ctrl Pts',(10.2086722175911,-24.0442828585718,-2.48665852888054));
#40899=CARTESIAN_POINT('Ctrl Pts',(10.2878717861949,-24.0608064550266,-2.13544798836442));
#40900=CARTESIAN_POINT('Ctrl Pts',(10.4275170772288,-24.0987376386477,-1.32395296018504));
#40901=CARTESIAN_POINT('Ctrl Pts',(10.4757999960315,-24.1201017840994,-0.862315821854623));
#40902=CARTESIAN_POINT('Ctrl Pts',(10.5161713237268,-24.1686157045272,0.199424976794982));
#40903=CARTESIAN_POINT('Ctrl Pts',(10.4876938255333,-24.1955169652023,0.798704439162373));
#40904=CARTESIAN_POINT('Ctrl Pts',(10.3927673562948,-24.2276343130389,1.5083423436313));
#40905=CARTESIAN_POINT('Ctrl Pts',(10.3753053972976,-24.2328851818079,1.62411251161865));
#40906=CARTESIAN_POINT('Ctrl Pts',(10.3559140709193,-24.2381415361801,1.73955303332087));
#40907=CARTESIAN_POINT('Ctrl Pts',(10.3559140377345,-23.4201872127662,1.73955323087673));
#40908=CARTESIAN_POINT('Ctrl Pts',(10.406224139909,-23.4065090324115,1.44004696449681));
#40909=CARTESIAN_POINT('Ctrl Pts',(10.4435295861151,-23.3929004977755,1.13842662890351));
#40910=CARTESIAN_POINT('Ctrl Pts',(10.4979431611934,-23.3622138170407,0.456729939028258));
#40911=CARTESIAN_POINT('Ctrl Pts',(10.5075946919293,-23.3451379950166,0.0765682733419336));
#40912=CARTESIAN_POINT('Ctrl Pts',(10.4884876459115,-23.3149182215354,-0.584724929674124));
#40913=CARTESIAN_POINT('Ctrl Pts',(10.469039939308,-23.3019523091401,-0.865723117446026));
#40914=CARTESIAN_POINT('Ctrl Pts',(10.3672043976137,-23.2589371370392,-1.79361707290191));
#40915=CARTESIAN_POINT('Ctrl Pts',(10.2358927282489,-23.2290341433094,-2.43362470669664));
#40916=CARTESIAN_POINT('Ctrl Pts',(9.91006544442555,-23.1784062867506,-3.50426303834268));
#40917=CARTESIAN_POINT('Ctrl Pts',(9.74437407547304,-23.15750927925,-3.94162844346253));
#40918=CARTESIAN_POINT('Ctrl Pts',(9.39420562564757,-23.119704904819,-4.70749177167167));
#40919=CARTESIAN_POINT('Ctrl Pts',(9.22015573169296,-23.1028177710418,-5.03987124081586));
#40920=CARTESIAN_POINT('Ctrl Pts',(8.8668634357367,-23.0711616140692,-5.63472971615912));
#40921=CARTESIAN_POINT('Ctrl Pts',(8.69277342211163,-23.0565457790609,-5.89975711545663));
#40922=CARTESIAN_POINT('Ctrl Pts',(8.171352561563,-23.0155657991684,-6.62024886433821));
#40923=CARTESIAN_POINT('Ctrl Pts',(7.79837287523769,-22.9893449493126,-7.05578526963895));
#40924=CARTESIAN_POINT('Ctrl Pts',(7.06535612250973,-22.9426303310857,-7.78221733902895));
#40925=CARTESIAN_POINT('Ctrl Pts',(6.71807931316477,-22.9220612514924,-8.08390867161846));
#40926=CARTESIAN_POINT('Ctrl Pts',(6.05662793146166,-22.8847833951965,-8.58638445909492));
#40927=CARTESIAN_POINT('Ctrl Pts',(5.74941291497919,-22.8680987420118,-8.79505471097264));
#40928=CARTESIAN_POINT('Ctrl Pts',(5.18990797552534,-22.8382339102335,-9.13322165807456));
#40929=CARTESIAN_POINT('Ctrl Pts',(4.94222124970648,-22.8252178309031,-9.26959164122858));
#40930=CARTESIAN_POINT('Ctrl Pts',(4.10539493328197,-22.782119710391,-9.68724213096674));
#40931=CARTESIAN_POINT('Ctrl Pts',(3.49553769443001,-22.7521873090204,-9.92361748713999));
#40932=CARTESIAN_POINT('Ctrl Pts',(2.41683688012316,-22.7014650792893,-10.2298359829262));
#40933=CARTESIAN_POINT('Ctrl Pts',(1.95792627690865,-22.6805043147014,-10.3274959996256));
#40934=CARTESIAN_POINT('Ctrl Pts',(1.15602594585778,-22.6441329257167,-10.4427587646851));
#40935=CARTESIAN_POINT('Ctrl Pts',(0.815865287064391,-22.628762285365,-10.4748254059024));
#40936=CARTESIAN_POINT('Ctrl Pts',(0.194645699797482,-22.600358412073,-10.5029390869844));
#40937=CARTESIAN_POINT('Ctrl Pts',(-0.0858451102346386,-22.5874473131349,
-10.5043916746554));
#40938=CARTESIAN_POINT('Ctrl Pts',(-1.01743073845812,-22.5444929550306,
-10.4718977688152));
#40939=CARTESIAN_POINT('Ctrl Pts',(-1.6652952669242,-22.5145928138781,-10.3885821791191));
#40940=CARTESIAN_POINT('Ctrl Pts',(-2.75584752866656,-22.4640236485553,
-10.1436377018274));
#40941=CARTESIAN_POINT('Ctrl Pts',(-3.20314257028947,-22.4431807456872,
-10.01139169134));
#40942=CARTESIAN_POINT('Ctrl Pts',(-3.97228551560262,-22.4063720486285,
-9.72714292012351));
#40943=CARTESIAN_POINT('Ctrl Pts',(-4.29796499089189,-22.390438848756,-9.58769290003277));
#40944=CARTESIAN_POINT('Ctrl Pts',(-4.87268905354279,-22.3612041365895,
-9.30642702146816));
#40945=CARTESIAN_POINT('Ctrl Pts',(-5.12415824032289,-22.3480402573149,
-9.1703698004908));
#40946=CARTESIAN_POINT('Ctrl Pts',(-5.9361095214585,-22.3045007329254,-8.68722756834665));
#40947=CARTESIAN_POINT('Ctrl Pts',(-6.46949146700468,-22.274288523468,-8.29765273153006));
#40948=CARTESIAN_POINT('Ctrl Pts',(-7.31903068547389,-22.2229760793682,
-7.54514475759568));
#40949=CARTESIAN_POINT('Ctrl Pts',(-7.65336598045431,-22.2017063732082,
-7.20579017911899));
#40950=CARTESIAN_POINT('Ctrl Pts',(-8.19613841000151,-22.1643093722904,
-6.57431773809772));
#40951=CARTESIAN_POINT('Ctrl Pts',(-8.41478982117273,-22.1482151012864,
-6.29203040106584));
#40952=CARTESIAN_POINT('Ctrl Pts',(-8.80430054692049,-22.1170094087629,
-5.73244242234787));
#40953=CARTESIAN_POINT('Ctrl Pts',(-8.97747011337554,-22.102019170908,-5.45725501845262));
#40954=CARTESIAN_POINT('Ctrl Pts',(-9.41030252966894,-22.0615496413099,
-4.69291805059709));
#40955=CARTESIAN_POINT('Ctrl Pts',(-9.64451601360296,-22.0362064635198,
-4.19053807975288));
#40956=CARTESIAN_POINT('Ctrl Pts',(-9.99791547121999,-21.9904499283073,
-3.24371744513277));
#40957=CARTESIAN_POINT('Ctrl Pts',(-10.1296434741463,-21.9699808940398,
-2.8054135521693));
#40958=CARTESIAN_POINT('Ctrl Pts',(-10.31734413195,-21.9325019284077,-1.99156133970853));
#40959=CARTESIAN_POINT('Ctrl Pts',(-10.3823447247696,-21.9155136750956,
-1.61889487774995));
#40960=CARTESIAN_POINT('Ctrl Pts',(-10.5030076144496,-21.8689692439359,
-0.607126987358097));
#40961=CARTESIAN_POINT('Ctrl Pts',(-10.5204832514869,-21.8392641814794,
0.0348922578667292));
#40962=CARTESIAN_POINT('Ctrl Pts',(-10.4449071686769,-21.785421023033,1.20908565829536));
#40963=CARTESIAN_POINT('Ctrl Pts',(-10.3696412030061,-21.7612284501406,
1.74026880283431));
#40964=CARTESIAN_POINT('Ctrl Pts',(-10.1247818277644,-21.710204092864,2.84958961418419));
#40965=CARTESIAN_POINT('Ctrl Pts',(-9.94536935611983,-21.6834558891121,
3.42359290542861));
#40966=CARTESIAN_POINT('Ctrl Pts',(-9.59710590798032,-21.6414012727804,
4.27412882816889));
#40967=CARTESIAN_POINT('Ctrl Pts',(-9.46294310112404,-21.6266997482495,
4.56347724468131));
#40968=CARTESIAN_POINT('Ctrl Pts',(-9.05704833891964,-21.5861763648574,
5.34371529786909));
#40969=CARTESIAN_POINT('Ctrl Pts',(-8.75883552642321,-21.5604901799677,
5.81964293282196));
#40970=CARTESIAN_POINT('Ctrl Pts',(-8.15172709732509,-21.514445948901,6.63538914960673));
#40971=CARTESIAN_POINT('Ctrl Pts',(-7.85585685223666,-21.4940221454076,
6.98316279103273));
#40972=CARTESIAN_POINT('Ctrl Pts',(-7.27284316228942,-21.4564448514398,
7.58433648259945));
#40973=CARTESIAN_POINT('Ctrl Pts',(-6.99266881941011,-21.4393122697469,
7.8434040017997));
#40974=CARTESIAN_POINT('Ctrl Pts',(-6.20550144937807,-21.3926213532581,
8.49549654692277));
#40975=CARTESIAN_POINT('Ctrl Pts',(-5.67558875802255,-21.3629161952602,
8.85829639766727));
#40976=CARTESIAN_POINT('Ctrl Pts',(-4.65071984931404,-21.3092081106712,
9.43003485904779));
#40977=CARTESIAN_POINT('Ctrl Pts',(-4.16644892800853,-21.2851465828459,
9.65378040094941));
#40978=CARTESIAN_POINT('Ctrl Pts',(-3.10190238043785,-21.2341148599773,
10.0505355741598));
#40979=CARTESIAN_POINT('Ctrl Pts',(-2.51942526000138,-21.2072357234102,
10.2121276927707));
#40980=CARTESIAN_POINT('Ctrl Pts',(-1.6136871428915,-21.1650814863832,10.381143529226));
#40981=CARTESIAN_POINT('Ctrl Pts',(-1.29859330519493,-21.1504174360658,
10.4252472504763));
#40982=CARTESIAN_POINT('Ctrl Pts',(-0.413545275006808,-21.1094624247547,
10.5083756119576));
#40983=CARTESIAN_POINT('Ctrl Pts',(0.158316546435473,-21.0833144906049,
10.5153193412997));
#40984=CARTESIAN_POINT('Ctrl Pts',(1.18818365570688,-21.0365871872097,10.4437586451435));
#40985=CARTESIAN_POINT('Ctrl Pts',(1.64584983720964,-21.0159369151384,10.3814767005508));
#40986=CARTESIAN_POINT('Ctrl Pts',(2.45742091444955,-20.9787649615925,10.2160014172027));
#40987=CARTESIAN_POINT('Ctrl Pts',(2.81280671748541,-20.9622699862602,10.1239180741488));
#40988=CARTESIAN_POINT('Ctrl Pts',(3.77045720939255,-20.9163944722653,9.82145297041031));
#40989=CARTESIAN_POINT('Ctrl Pts',(4.35952789963926,-20.8868457017479,9.57453993269119));
#40990=CARTESIAN_POINT('Ctrl Pts',(5.38484932548846,-20.833709836774,9.03040909797843));
#40991=CARTESIAN_POINT('Ctrl Pts',(5.82815004985385,-20.8100559510091,8.75086152133243));
#40992=CARTESIAN_POINT('Ctrl Pts',(6.75946559695342,-20.7579892093737,8.06129183010583));
#40993=CARTESIAN_POINT('Ctrl Pts',(7.23477325212092,-20.7296956407351,7.63759444106696));
#40994=CARTESIAN_POINT('Ctrl Pts',(7.9051425651324,-20.6847591221548,6.92093582610613));
#40995=CARTESIAN_POINT('Ctrl Pts',(8.1287956607558,-20.6687988423574,6.65682438153097));
#40996=CARTESIAN_POINT('Ctrl Pts',(8.66423284190235,-20.6282304641132,5.95721583962474));
#40997=CARTESIAN_POINT('Ctrl Pts',(8.95650810981446,-20.6037577438035,5.50802474448138));
#40998=CARTESIAN_POINT('Ctrl Pts',(9.43837940585966,-20.558315149391,4.62688874302381));
#40999=CARTESIAN_POINT('Ctrl Pts',(9.63564732829537,-20.5373260610621,4.20064404240522));
#41000=CARTESIAN_POINT('Ctrl Pts',(9.93082880038755,-20.500341761071,3.4315330518541));
#41001=CARTESIAN_POINT('Ctrl Pts',(10.0410467818482,-20.484379886629,3.09421328464689));
#41002=CARTESIAN_POINT('Ctrl Pts',(10.2093893104803,-20.4550281480888,2.47429834566571));
#41003=CARTESIAN_POINT('Ctrl Pts',(10.2733465128307,-20.441775257999,2.19365705868249));
#41004=CARTESIAN_POINT('Ctrl Pts',(10.3362442290325,-20.4258473136096,1.85375707557567));
#41005=CARTESIAN_POINT('Ctrl Pts',(10.3463163024248,-20.4231771163331,1.79669050433489));
#41006=CARTESIAN_POINT('Ctrl Pts',(10.3559140572458,-20.4205078998763,1.73955311472209));
#41007=CARTESIAN_POINT('Origin',(0.,-13.3748739960349,0.));
#41008=CARTESIAN_POINT('',(-12.1744999967658,-23.8748739960011,0.000280623926547941));
#41009=CARTESIAN_POINT('Ctrl Pts',(7.41272179941102,-21.9374490664136,-9.65763976210216));
#41010=CARTESIAN_POINT('Ctrl Pts',(7.63814242828085,-21.9485939981776,-9.48461814907643));
#41011=CARTESIAN_POINT('Ctrl Pts',(7.85752362648661,-21.9597389299416,-9.30368459558577));
#41012=CARTESIAN_POINT('Ctrl Pts',(8.07031593182521,-21.9708838617056,-9.11528666639334));
#41013=CARTESIAN_POINT('Ctrl Pts',(8.28308879835672,-21.9820277753681,-8.92690594755537));
#41014=CARTESIAN_POINT('Ctrl Pts',(8.48927377437015,-21.9931716890305,-8.7310623915339));
#41015=CARTESIAN_POINT('Ctrl Pts',(8.68835576973433,-22.004315602693,-8.5282427421201));
#41016=CARTESIAN_POINT('Ctrl Pts',(8.88745520365534,-22.0154604925049,-8.32540532675024));
#41017=CARTESIAN_POINT('Ctrl Pts',(9.07945022461544,-22.0266053823167,-8.11559078522033));
#41018=CARTESIAN_POINT('Ctrl Pts',(9.26386275874899,-22.0377502721286,-7.89932256823732));
#41019=CARTESIAN_POINT('Ctrl Pts',(9.44827425420413,-22.0488950991684,-7.68305556935552));
#41020=CARTESIAN_POINT('Ctrl Pts',(9.62510317680151,-22.0600399262082,-7.46033517215365));
#41021=CARTESIAN_POINT('Ctrl Pts',(9.79391130575108,-22.071184753248,-7.23171843928408));
#41022=CARTESIAN_POINT('Ctrl Pts',(9.96275714478459,-22.0823320699331,-7.00305063567375));
#41023=CARTESIAN_POINT('Ctrl Pts',(10.1235784500975,-22.0934793866182,-6.76848407820211));
#41024=CARTESIAN_POINT('Ctrl Pts',(10.2759790307611,-22.1046267033033,-6.52860668208442));
#41025=CARTESIAN_POINT('Ctrl Pts',(10.396545869554,-22.113445545908,-6.33883536217311));
#41026=CARTESIAN_POINT('Ctrl Pts',(10.5118432533725,-22.1222643885128,-6.14574079649067));
#41027=CARTESIAN_POINT('Ctrl Pts',(10.6216946965625,-22.1310832311175,-5.94962620868038));
#41028=CARTESIAN_POINT('Ctrl Pts',(10.7605504536662,-22.142230531791,-5.70173106248375));
#41029=CARTESIAN_POINT('Ctrl Pts',(10.8907448834759,-22.1533778324646,-5.44893572672557));
#41030=CARTESIAN_POINT('Ctrl Pts',(11.0119467530863,-22.1645251331381,-5.19186661588989));
#41031=CARTESIAN_POINT('Ctrl Pts',(11.1331280357991,-22.1756705403727,-4.93484116985485));
#41032=CARTESIAN_POINT('Ctrl Pts',(11.2453196941389,-22.1868159476073,-4.67354363924067));
#41033=CARTESIAN_POINT('Ctrl Pts',(11.3482374041766,-22.197961354842,-4.4086231488353));
#41034=CARTESIAN_POINT('Ctrl Pts',(11.4511436882338,-22.2091055247074,-4.14373207004787));
#41035=CARTESIAN_POINT('Ctrl Pts',(11.5447779833641,-22.2202496945728,-3.87521908322489));
#41036=CARTESIAN_POINT('Ctrl Pts',(11.6289044340638,-22.2313938644382,-3.60375247671244));
#41037=CARTESIAN_POINT('Ctrl Pts',(11.7156802739049,-22.2428889969602,-3.32373658904568));
#41038=CARTESIAN_POINT('Ctrl Pts',(11.7923396078499,-22.2543841294822,-3.04057831121346));
#41039=CARTESIAN_POINT('Ctrl Pts',(11.8586790366336,-22.2658792620043,-2.75502844923715));
#41040=CARTESIAN_POINT('Ctrl Pts',(11.9229964655407,-22.2770240273771,-2.47818203551626));
#41041=CARTESIAN_POINT('Ctrl Pts',(11.9776137036276,-22.2881687927499,-2.19908793968349));
#41042=CARTESIAN_POINT('Ctrl Pts',(12.0223969991253,-22.2993135581228,-1.91844224448467));
#41043=CARTESIAN_POINT('Ctrl Pts',(12.0692921285266,-22.3109838742194,-1.62456221520089));
#41044=CARTESIAN_POINT('Ctrl Pts',(12.1054034747325,-22.322654190316,-1.32898104250057));
#41045=CARTESIAN_POINT('Ctrl Pts',(12.1306380526509,-22.3343245064127,-1.03250699057049));
#41046=CARTESIAN_POINT('Ctrl Pts',(12.1558726305694,-22.3459948225093,-0.736032938640407));
#41047=CARTESIAN_POINT('Ctrl Pts',(12.1702304204935,-22.3576651386059,-0.438666342520084));
#41048=CARTESIAN_POINT('Ctrl Pts',(12.1736809240298,-22.3693354547026,-0.14121972211462));
#41049=CARTESIAN_POINT('Ctrl Pts',(12.1769767929329,-22.3804827645107,0.142896800657586));
#41050=CARTESIAN_POINT('Ctrl Pts',(12.1703224929076,-22.3916300743188,0.427171187125004));
#41051=CARTESIAN_POINT('Ctrl Pts',(12.1537269468445,-22.4027773841269,0.710894894865639));
#41052=CARTESIAN_POINT('Ctrl Pts',(12.1371342194696,-22.4139228006082,0.99457041324932));
#41053=CARTESIAN_POINT('Ctrl Pts',(12.11060363268,-22.4250682170895,1.2776951734493));
#41054=CARTESIAN_POINT('Ctrl Pts',(12.074196166311,-22.4362136335708,1.55956313993394));
#41055=CARTESIAN_POINT('Ctrl Pts',(12.0377927416301,-22.4473578127703,1.84139981551791));
#41056=CARTESIAN_POINT('Ctrl Pts',(11.9915146609846,-22.4585019919697,2.12197971150438));
#41057=CARTESIAN_POINT('Ctrl Pts',(11.9354746331794,-22.4696461711692,2.40060315977681));
#41058=CARTESIAN_POINT('Ctrl Pts',(11.8776698234813,-22.4811412967624,2.68800086523175));
#41059=CARTESIAN_POINT('Ctrl Pts',(11.8094783169454,-22.4926364223556,2.97331661069409));
#41060=CARTESIAN_POINT('Ctrl Pts',(11.7310808084977,-22.5041315479488,3.25579380712257));
#41061=CARTESIAN_POINT('Ctrl Pts',(11.6550727153316,-22.5152763227554,3.52966160583902));
#41062=CARTESIAN_POINT('Ctrl Pts',(11.5694716039288,-22.5264210975619,3.80086105222759));
#41063=CARTESIAN_POINT('Ctrl Pts',(11.474493137458,-22.5375658723685,4.06871693392769));
#41064=CARTESIAN_POINT('Ctrl Pts',(11.3750360097731,-22.549236173355,4.34920342331078));
#41065=CARTESIAN_POINT('Ctrl Pts',(11.2652959853262,-22.5609064743416,4.62602313302054));
#41066=CARTESIAN_POINT('Ctrl Pts',(11.1455782047075,-22.5725767753281,4.89842186145174));
#41067=CARTESIAN_POINT('Ctrl Pts',(11.0258604240889,-22.5842470763146,5.17082058988296));
#41068=CARTESIAN_POINT('Ctrl Pts',(10.8961650303231,-22.5959173773012,5.43879803342295));
#41069=CARTESIAN_POINT('Ctrl Pts',(10.7568540674013,-22.6075876782877,5.7016261559867));
#41070=CARTESIAN_POINT('Ctrl Pts',(10.6237862289835,-22.6187349828027,5.95267581791911));
#41071=CARTESIAN_POINT('Ctrl Pts',(10.4819059659421,-22.6298822873177,6.19910251958811));
#41072=CARTESIAN_POINT('Ctrl Pts',(10.331560180348,-22.6410295918327,6.44028838561183));
#41073=CARTESIAN_POINT('Ctrl Pts',(10.1812399312278,-22.65217500296,6.68143328582788));
#41074=CARTESIAN_POINT('Ctrl Pts',(10.0224571713426,-22.6633204140874,6.91733890132943));
#41075=CARTESIAN_POINT('Ctrl Pts',(9.85560331246683,-22.6744658252148,7.14741446939331));
#41076=CARTESIAN_POINT('Ctrl Pts',(9.68876797717992,-22.6856099990138,7.37746449519372));
#41077=CARTESIAN_POINT('Ctrl Pts',(9.51386348868994,-22.6967541728128,7.60168555009459));
#41078=CARTESIAN_POINT('Ctrl Pts',(9.33132363306435,-22.7078983466118,7.81951721687565));
#41079=CARTESIAN_POINT('Ctrl Pts',(9.14303517522473,-22.7193934762169,8.04420890662349));
#41080=CARTESIAN_POINT('Ctrl Pts',(8.94662282970408,-22.7308886058219,8.2621020201305));
#41081=CARTESIAN_POINT('Ctrl Pts',(8.74260731912746,-22.742383735427,8.47261869279735));
#41082=CARTESIAN_POINT('Ctrl Pts',(8.54481000069459,-22.7535285047855,8.67671902429285));
#41083=CARTESIAN_POINT('Ctrl Pts',(8.33986632224137,-22.7646732741439,8.87388570935971));
#41084=CARTESIAN_POINT('Ctrl Pts',(8.12828876731095,-22.7758180435024,9.06362907257389));
#41085=CARTESIAN_POINT('Ctrl Pts',(7.90673410626793,-22.7874883532308,9.26231993340696));
#41086=CARTESIAN_POINT('Ctrl Pts',(7.67790509962409,-22.7991586629592,9.45287030906363));
#41087=CARTESIAN_POINT('Ctrl Pts',(7.44243059986101,-22.8108289726876,9.63476398342235));
#41088=CARTESIAN_POINT('Ctrl Pts',(7.20695610009792,-22.822499282416,9.81665765778107));
#41089=CARTESIAN_POINT('Ctrl Pts',(6.9648363780942,-22.8341695921444,9.98989443269218));
#41090=CARTESIAN_POINT('Ctrl Pts',(6.71673773003182,-22.8458399018728,10.1540082980056));
#41091=CARTESIAN_POINT('Ctrl Pts',(6.47975757864706,-22.8569872087515,10.3107674297061));
#41092=CARTESIAN_POINT('Ctrl Pts',(6.23725183406651,-22.8681345156302,10.4592501796308));
#41093=CARTESIAN_POINT('Ctrl Pts',(5.98982077868779,-22.8792818225089,10.5990800208886));
#41094=CARTESIAN_POINT('Ctrl Pts',(5.7424317492995,-22.8904272360254,10.7388861121464));
#41095=CARTESIAN_POINT('Ctrl Pts',(5.49011931144717,-22.9015726495419,10.8700420977849));
#41096=CARTESIAN_POINT('Ctrl Pts',(5.2335098553344,-22.9127180630584,10.9922165573699));
#41097=CARTESIAN_POINT('Ctrl Pts',(4.97692888674906,-22.9238622392655,11.1143774537437));
#41098=CARTESIAN_POINT('Ctrl Pts',(4.71605209324548,-22.9350064154727,11.227558700446));
#41099=CARTESIAN_POINT('Ctrl Pts',(4.45152855075324,-22.9461505916799,11.3314758002578));
#41100=CARTESIAN_POINT('Ctrl Pts',(4.17867465159937,-22.9576457194947,11.4386654500156));
#41101=CARTESIAN_POINT('Ctrl Pts',(3.90194086783386,-22.9691408473095,11.535997888534));
#41102=CARTESIAN_POINT('Ctrl Pts',(3.62206095978642,-22.9806359751244,11.6232149018071));
#41103=CARTESIAN_POINT('Ctrl Pts',(3.3507114148116,-22.9917807469079,11.7077736578494));
#41104=CARTESIAN_POINT('Ctrl Pts',(3.07640495140956,-23.0029255186914,11.7828243840286));
#41105=CARTESIAN_POINT('Ctrl Pts',(2.79982589396561,-23.014070290475,11.8481823590574));
#41106=CARTESIAN_POINT('Ctrl Pts',(2.51020469315729,-23.0257405963054,11.9166223030835));
#41107=CARTESIAN_POINT('Ctrl Pts',(2.21809172121681,-23.0374109021359,11.9744332999611));
#41108=CARTESIAN_POINT('Ctrl Pts',(1.92428618151177,-23.0490812079664,12.0214630116988));
#41109=CARTESIAN_POINT('Ctrl Pts',(1.63048064180675,-23.0607515137969,12.0684927234366));
#41110=CARTESIAN_POINT('Ctrl Pts',(1.33498286700784,-23.0724218196274,12.1047411056734));
#41111=CARTESIAN_POINT('Ctrl Pts',(1.03860091274412,-23.0840921254579,12.1301178227603));
#41112=CARTESIAN_POINT('Ctrl Pts',(0.755501187515748,-23.0952394315824,
12.1543572932515));
#41113=CARTESIAN_POINT('Ctrl Pts',(0.471510238288568,-23.1063867377068,
12.1686853376153));
#41114=CARTESIAN_POINT('Ctrl Pts',(0.187335335693578,-23.1175340438313,
12.1730586017648));
#41115=CARTESIAN_POINT('Ctrl Pts',(-0.0967912998095614,-23.1286794565864,
12.1774311231157));
#41116=CARTESIAN_POINT('Ctrl Pts',(-0.381101559686401,-23.1398248693415,
12.1718522358687));
#41117=CARTESIAN_POINT('Ctrl Pts',(-0.664886834336528,-23.1509702820966,
12.1563306860058));
#41118=CARTESIAN_POINT('Ctrl Pts',(-0.948640604399958,-23.1621144575373,
12.1408108592767));
#41119=CARTESIAN_POINT('Ctrl Pts',(-1.2318692393348,-23.1732586329779,12.1153505885898));
#41120=CARTESIAN_POINT('Ctrl Pts',(-1.51386666477452,-23.1844028084186,
12.0800106776147));
#41121=CARTESIAN_POINT('Ctrl Pts',(-1.80474476760346,-23.195897936804,12.0435578403501));
#41122=CARTESIAN_POINT('Ctrl Pts',(-2.09431256209703,-23.2073930651893,
11.9965930464181));
#41123=CARTESIAN_POINT('Ctrl Pts',(-2.38180219291559,-23.2188881935747,
11.9392407029854));
#41124=CARTESIAN_POINT('Ctrl Pts',(-2.66052949347101,-23.2300329645888,
11.8836363884227));
#41125=CARTESIAN_POINT('Ctrl Pts',(-2.93730316054586,-23.2411777356028,
11.8182684020138));
#41126=CARTESIAN_POINT('Ctrl Pts',(-3.21143391640609,-23.2523225066169,
11.743302025008));
#41127=CARTESIAN_POINT('Ctrl Pts',(-3.49849141578954,-23.2639928136879,
11.6648005790335));
#41128=CARTESIAN_POINT('Ctrl Pts',(-3.78265044479702,-23.2756631207589,
11.5757738130286));
#41129=CARTESIAN_POINT('Ctrl Pts',(-4.06313635096133,-23.2873334278299,
11.4764704174888));
#41130=CARTESIAN_POINT('Ctrl Pts',(-4.34362225712563,-23.299003734901,11.3771670219491));
#41131=CARTESIAN_POINT('Ctrl Pts',(-4.62043472711151,-23.310674041972,11.2675871171198));
#41132=CARTESIAN_POINT('Ctrl Pts',(-4.89282100638345,-23.322344349043,11.1480380717637));
#41133=CARTESIAN_POINT('Ctrl Pts',(-5.15300038646404,-23.3334916552407,
11.0338465765346));
#41134=CARTESIAN_POINT('Ctrl Pts',(-5.40921927779757,-23.3446389614383,
10.9105257231928));
#41135=CARTESIAN_POINT('Ctrl Pts',(-5.66083590451648,-23.355786267636,10.7783759032675));
#41136=CARTESIAN_POINT('Ctrl Pts',(-5.91240979416356,-23.3669316804642,
10.6462485289827));
#41137=CARTESIAN_POINT('Ctrl Pts',(-6.15938274378058,-23.3780770932925,
10.5052953060483));
#41138=CARTESIAN_POINT('Ctrl Pts',(-6.40113673390645,-23.3892225061207,
10.3558630139566));
#41139=CARTESIAN_POINT('Ctrl Pts',(-6.64286388556777,-23.4003666816343,
10.2064473111806));
#41140=CARTESIAN_POINT('Ctrl Pts',(-6.87937300783742,-23.4115108571478,
10.0485545591068));
#41141=CARTESIAN_POINT('Ctrl Pts',(-7.11007321917927,-23.4226550326614,
9.882576034006));
#41142=CARTESIAN_POINT('Ctrl Pts',(-7.34803865072143,-23.4341501609919,
9.71137050661351));
#41143=CARTESIAN_POINT('Ctrl Pts',(-7.57982312721504,-23.4456452893225,
9.53156184412831));
#41144=CARTESIAN_POINT('Ctrl Pts',(-7.80481195646738,-23.457140417653,9.34362673559812));
#41145=CARTESIAN_POINT('Ctrl Pts',(-8.02294340543191,-23.4682851887384,
9.16141965593453));
#41146=CARTESIAN_POINT('Ctrl Pts',(-8.23468710462325,-23.4794299598237,
8.97157434171908));
#41147=CARTESIAN_POINT('Ctrl Pts',(-8.43951691801119,-23.4905747309091,
8.77456576934739));
#41148=CARTESIAN_POINT('Ctrl Pts',(-8.65400555820757,-23.5022450378623,
8.56826718372596));
#41149=CARTESIAN_POINT('Ctrl Pts',(-8.86091234015456,-23.5139153448154,
8.35411373254376));
#41150=CARTESIAN_POINT('Ctrl Pts',(-9.05967607823019,-23.5255856517686,
8.13269448630303));
#41151=CARTESIAN_POINT('Ctrl Pts',(-9.2584398163058,-23.5372559587218,7.91127524006232));
#41152=CARTESIAN_POINT('Ctrl Pts',(-9.44906029292414,-23.5489262656749,
7.68259045429057));
#41153=CARTESIAN_POINT('Ctrl Pts',(-9.631023630308,-23.5605965726281,7.44727024368318));
#41154=CARTESIAN_POINT('Ctrl Pts',(-9.8048323458045,-23.5717438789489,7.22249582415408));
#41155=CARTESIAN_POINT('Ctrl Pts',(-9.97079470968131,-23.5828911852698,
6.99160050424424));
#41156=CARTESIAN_POINT('Ctrl Pts',(-10.128490951645,-23.5940384915906,6.75515516420202));
#41157=CARTESIAN_POINT('Ctrl Pts',(-10.286160408936,-23.6051839045438,6.51874998434983));
#41158=CARTESIAN_POINT('Ctrl Pts',(-10.4355663994461,-23.6163293174971,
6.27679688823947));
#41159=CARTESIAN_POINT('Ctrl Pts',(-10.5763322111555,-23.6274747304504,
6.0298961192773));
#41160=CARTESIAN_POINT('Ctrl Pts',(-10.7170823956828,-23.6386189060904,
5.78302276011893));
#41161=CARTESIAN_POINT('Ctrl Pts',(-10.8491941846832,-23.6497630817305,
5.53120305658148));
#41162=CARTESIAN_POINT('Ctrl Pts',(-10.9723359885886,-23.6609072573705,
5.27506333644663));
#41163=CARTESIAN_POINT('Ctrl Pts',(-11.0993557765869,-23.6724023856074,
5.01085725924436));
#41164=CARTESIAN_POINT('Ctrl Pts',(-11.2168313213538,-23.6838975138443,
4.74205492746937));
#41165=CARTESIAN_POINT('Ctrl Pts',(-11.3244509997133,-23.6953926420812,
4.46936906118676));
#41166=CARTESIAN_POINT('Ctrl Pts',(-11.4287905658947,-23.7065374132952,
4.20499431647958));
#41167=CARTESIAN_POINT('Ctrl Pts',(-11.5238660555388,-23.7176821845091,
3.93696952183191));
#41168=CARTESIAN_POINT('Ctrl Pts',(-11.6094427838768,-23.7288269557231,
3.66596351562464));
#41169=CARTESIAN_POINT('Ctrl Pts',(-11.6990549123853,-23.7404972624715,
3.38217812762871));
#41170=CARTESIAN_POINT('Ctrl Pts',(-11.7782507937505,-23.7521675692198,
3.09512390584126));
#41171=CARTESIAN_POINT('Ctrl Pts',(-11.8468195663286,-23.7638378759682,
2.80558664326246));
#41172=CARTESIAN_POINT('Ctrl Pts',(-11.9153883389068,-23.7755081827165,
2.51604938068365));
#41173=CARTESIAN_POINT('Ctrl Pts',(-11.9733299339243,-23.7871784894648,
2.22402940580713));
#41174=CARTESIAN_POINT('Ctrl Pts',(-12.0204946704578,-23.7988487962132,
1.93032591224761));
#41175=CARTESIAN_POINT('Ctrl Pts',(-12.0672414471629,-23.8104156841837,
1.63922513145235));
#41176=CARTESIAN_POINT('Ctrl Pts',(-12.1034122499846,-23.8219825721543,
1.34640866791079));
#41177=CARTESIAN_POINT('Ctrl Pts',(-12.1289081894145,-23.8335494601249,
1.05263307128082));
#41178=CARTESIAN_POINT('Ctrl Pts',(-12.1543967460716,-23.8451129987108,
0.758942542255195));
#41179=CARTESIAN_POINT('Ctrl Pts',(-12.1692165959912,-23.8566765372968,
0.464293654495028));
#41180=CARTESIAN_POINT('Ctrl Pts',(-12.1733207336769,-23.8682400758828,
0.169447823923155));
#41181=CARTESIAN_POINT('Ctrl Pts',(-12.1741055719096,-23.8704513825889,
0.11306416959796));
#41182=CARTESIAN_POINT('Ctrl Pts',(-12.1744986969062,-23.872662689295,0.056673323816421));
#41183=CARTESIAN_POINT('Ctrl Pts',(-12.1744999967658,-23.8748739960011,
0.000280623926556051));
#41184=CARTESIAN_POINT('Ctrl Pts',(-12.1744999967658,-23.8748739960349,
0.00028062306491734));
#41185=CARTESIAN_POINT('Ctrl Pts',(-12.1745065428157,-23.8860100974646,
-0.283712015376132));
#41186=CARTESIAN_POINT('Ctrl Pts',(-12.1645717688562,-23.8971461988943,
-0.567720156626778));
#41187=CARTESIAN_POINT('Ctrl Pts',(-12.1447184939399,-23.908282300324,-0.8510363993127));
#41188=CARTESIAN_POINT('Ctrl Pts',(-12.1248634023349,-23.9194194207708,
-1.13437856706043));
#41189=CARTESIAN_POINT('Ctrl Pts',(-12.0950880117066,-23.9305565412177,
-1.41702844262597));
#41190=CARTESIAN_POINT('Ctrl Pts',(-12.0554671639295,-23.9416936616646,
-1.6982819876032));
#41191=CARTESIAN_POINT('Ctrl Pts',(-12.0158465226463,-23.9528307240675,
-1.97953406675724));
#41192=CARTESIAN_POINT('Ctrl Pts',(-11.9663805663668,-23.9639677864705,
-2.25938956526504));
#41193=CARTESIAN_POINT('Ctrl Pts',(-11.9071957223858,-23.9751048488735,
-2.53715200151623));
#41194=CARTESIAN_POINT('Ctrl Pts',(-11.8479967642311,-23.9862445672002,
-2.81498067748367));
#41195=CARTESIAN_POINT('Ctrl Pts',(-11.7790743410825,-23.9973842855269,
-3.09071503164591));
#41196=CARTESIAN_POINT('Ctrl Pts',(-11.7006058479935,-24.0085240038537,
-3.36366957947735));
#41197=CARTESIAN_POINT('Ctrl Pts',(-11.6335067433188,-24.0180496758352,
-3.59707543519565));
#41198=CARTESIAN_POINT('Ctrl Pts',(-11.5594283093542,-24.0275753478167,
-3.82844876548518));
#41199=CARTESIAN_POINT('Ctrl Pts',(-11.4785103889095,-24.0371010197983,
-4.05736977630798));
#41200=CARTESIAN_POINT('Ctrl Pts',(-11.3838171384972,-24.0482483260728,
-4.32526191297343));
#41201=CARTESIAN_POINT('Ctrl Pts',(-11.2797273169031,-24.0593956323473,
-4.58987760285483));
#41202=CARTESIAN_POINT('Ctrl Pts',(-11.1664931690163,-24.0705429386218,
-4.85055466481025));
#41203=CARTESIAN_POINT('Ctrl Pts',(-11.053278253932,-24.081688351528,-5.11118745080703));
#41204=CARTESIAN_POINT('Ctrl Pts',(-10.9309222196804,-24.0928337644342,
-5.36788269991822));
#41205=CARTESIAN_POINT('Ctrl Pts',(-10.7997253247509,-24.1039791773405,
-5.61999850177324));
#41206=CARTESIAN_POINT('Ctrl Pts',(-10.6685429947127,-24.115123352933,-5.87208631486202));
#41207=CARTESIAN_POINT('Ctrl Pts',(-10.5285218869459,-24.1262675285254,
-6.11959545930329));
#41208=CARTESIAN_POINT('Ctrl Pts',(-10.3800086368805,-24.1374117041179,
-6.36190780727653));
#41209=CARTESIAN_POINT('Ctrl Pts',(-10.2268184035207,-24.14890683239,-6.61185106227649));
#41210=CARTESIAN_POINT('Ctrl Pts',(-10.0645926378427,-24.1604019606621,
-6.85626464349746));
#41211=CARTESIAN_POINT('Ctrl Pts',(-9.89376139950918,-24.1718970889342,
-7.09450037843273));
#41212=CARTESIAN_POINT('Ctrl Pts',(-9.72813688326918,-24.1830418601,-7.32547498667565));
#41213=CARTESIAN_POINT('Ctrl Pts',(-9.55442385726194,-24.1941866312657,
-7.55064253139713));
#41214=CARTESIAN_POINT('Ctrl Pts',(-9.37305720387854,-24.2053314024315,
-7.76944328139543));
#41215=CARTESIAN_POINT('Ctrl Pts',(-9.18313814126281,-24.2170017092568,
-7.99856165880439));
#41216=CARTESIAN_POINT('Ctrl Pts',(-8.98482646679887,-24.2286720160821,
-8.22069809174982));
#41217=CARTESIAN_POINT('Ctrl Pts',(-8.77866826149681,-24.2403423229074,
-8.43524948087421));
#41218=CARTESIAN_POINT('Ctrl Pts',(-8.57251005619474,-24.2520126297327,
-8.6498008699986));
#41219=CARTESIAN_POINT('Ctrl Pts',(-8.35850555884004,-24.263682936558,-8.85676697946432));
#41220=CARTESIAN_POINT('Ctrl Pts',(-8.13724527165577,-24.2753532433833,
-9.05558886207384));
#41221=CARTESIAN_POINT('Ctrl Pts',(-7.92590068440107,-24.2865005496194,
-9.24550061375804));
#41222=CARTESIAN_POINT('Ctrl Pts',(-7.70787322336667,-24.2976478558555,
-9.42803877404122));
#41223=CARTESIAN_POINT('Ctrl Pts',(-7.48370125772818,-24.3087951620916,
-9.60274261526766));
#41224=CARTESIAN_POINT('Ctrl Pts',(-7.25956736767171,-24.3199405749591,
-9.77741678306721));
#41225=CARTESIAN_POINT('Ctrl Pts',(-7.02929126696434,-24.3310859878265,
-9.94425912456056));
#41226=CARTESIAN_POINT('Ctrl Pts',(-6.79344378337951,-24.342231400694,-10.1028496876902));
#41227=CARTESIAN_POINT('Ctrl Pts',(-6.55762248253287,-24.3533755762473,
-10.2614226448012));
#41228=CARTESIAN_POINT('Ctrl Pts',(-6.31623125517515,-24.3645197518006,
-10.4117455039978));
#41229=CARTESIAN_POINT('Ctrl Pts',(-6.06987027004878,-24.3756639273539,
-10.5534413891762));
#41230=CARTESIAN_POINT('Ctrl Pts',(-5.81575087656889,-24.3871590556551,
-10.6995995658927));
#41231=CARTESIAN_POINT('Ctrl Pts',(-5.55634388989934,-24.3986541839563,
-10.836578445479));
#41232=CARTESIAN_POINT('Ctrl Pts',(-5.29233710829935,-24.4101493122576,
-10.9640146927172));
#41233=CARTESIAN_POINT('Ctrl Pts',(-5.03637692415595,-24.4212940833839,
-11.0875668420671));
#41234=CARTESIAN_POINT('Ctrl Pts',(-4.776093436397,-24.4324388545102,-11.2021493190998));
#41235=CARTESIAN_POINT('Ctrl Pts',(-4.51213635499412,-24.4435836256365,
-11.3074787536365));
#41236=CARTESIAN_POINT('Ctrl Pts',(-4.2357322807886,-24.4552539325252,-11.4177750362176));
#41237=CARTESIAN_POINT('Ctrl Pts',(-3.95530011241909,-24.4669242394138,
-11.517924499486));
#41238=CARTESIAN_POINT('Ctrl Pts',(-3.67160795292729,-24.4785945463025,
-11.6076589065152));
#41239=CARTESIAN_POINT('Ctrl Pts',(-3.38791579343547,-24.4902648531912,
-11.6973933135444));
#41240=CARTESIAN_POINT('Ctrl Pts',(-3.10096396534875,-24.5019351600798,
-11.7767125715228));
#41241=CARTESIAN_POINT('Ctrl Pts',(-2.81153844769576,-24.5136054669685,
-11.8454084694082));
#41242=CARTESIAN_POINT('Ctrl Pts',(-2.53508343133578,-24.5247527732184,
-11.9110257851439));
#41243=CARTESIAN_POINT('Ctrl Pts',(-2.25628900057298,-24.5359000794684,
-11.9669705731406));
#41244=CARTESIAN_POINT('Ctrl Pts',(-1.97584835600998,-24.5470473857183,
-12.0130959175415));
#41245=CARTESIAN_POINT('Ctrl Pts',(-1.69545534425414,-24.5581927985997,
-12.0592134275587));
#41246=CARTESIAN_POINT('Ctrl Pts',(-1.41341694004882,-24.5693382114811,
-12.0955147805296));
#41247=CARTESIAN_POINT('Ctrl Pts',(-1.13043533186696,-24.5804836243626,
-12.1219043970189));
#41248=CARTESIAN_POINT('Ctrl Pts',(-0.847485139039732,-24.59162779993,-12.1482910838508));
#41249=CARTESIAN_POINT('Ctrl Pts',(-0.563592216852522,-24.6027719754975,
-12.1647682066767));
#41250=CARTESIAN_POINT('Ctrl Pts',(-0.27946390335161,-24.6139161510649,
-12.1712920504244));
#41251=CARTESIAN_POINT('Ctrl Pts',(0.0136121878271691,-24.6254112793556,
-12.178021343262));
#41252=CARTESIAN_POINT('Ctrl Pts',(0.306938440053736,-24.6369064076464,
-12.1741602840482));
#41253=CARTESIAN_POINT('Ctrl Pts',(0.599737050830206,-24.6484015359371,
-12.1597189819445));
#41254=CARTESIAN_POINT('Ctrl Pts',(0.883611525722814,-24.6595463070775,
-12.1457178326884));
#41255=CARTESIAN_POINT('Ctrl Pts',(1.16698976785748,-24.670691078218,-12.1217718491365));
#41256=CARTESIAN_POINT('Ctrl Pts',(1.44916568538212,-24.6818358493585,-12.0879431280227));
#41257=CARTESIAN_POINT('Ctrl Pts',(1.7446477106438,-24.6935061562243,-12.0525192012949));
#41258=CARTESIAN_POINT('Ctrl Pts',(2.03881097517401,-24.7051764630902,-12.0062580999378));
#41259=CARTESIAN_POINT('Ctrl Pts',(2.33085267230979,-24.716846769956,-11.9492918647921));
#41260=CARTESIAN_POINT('Ctrl Pts',(2.62289436944556,-24.7285170768219,-11.8923256296464));
#41261=CARTESIAN_POINT('Ctrl Pts',(2.91281417157282,-24.7401873836877,-11.8246543335606));
#41262=CARTESIAN_POINT('Ctrl Pts',(3.19982230071158,-24.7518576905535,-11.7464712783827));
#41263=CARTESIAN_POINT('Ctrl Pts',(3.4739656115066,-24.7630048889684,-11.6717926911982));
#41264=CARTESIAN_POINT('Ctrl Pts',(3.74553441079381,-24.7741520873833,-11.5875016792656));
#41265=CARTESIAN_POINT('Ctrl Pts',(4.01384973800586,-24.7852992857982,-11.4938009609837));
#41266=CARTESIAN_POINT('Ctrl Pts',(4.28211826815581,-24.7964445400225,-11.400116585109));
#41267=CARTESIAN_POINT('Ctrl Pts',(4.54713420746316,-24.8075897942468,-11.2970258675264));
#41268=CARTESIAN_POINT('Ctrl Pts',(4.8082352784448,-24.8187350484711,-11.1847808989322));
#41269=CARTESIAN_POINT('Ctrl Pts',(5.0693226528587,-24.8298797180493,-11.0725418183675));
#41270=CARTESIAN_POINT('Ctrl Pts',(5.32649532310743,-24.8410243876275,-10.9511495489443));
#41271=CARTESIAN_POINT('Ctrl Pts',(5.57911119597613,-24.8521690572056,-10.8209042373054));
#41272=CARTESIAN_POINT('Ctrl Pts',(5.83170819246218,-24.8633128940133,-10.6906686580729));
#41273=CARTESIAN_POINT('Ctrl Pts',(6.07974883505326,-24.874456730821,-10.5515814810599));
#41274=CARTESIAN_POINT('Ctrl Pts',(6.32261488353058,-24.8856005676286,-10.403989200521));
#41275=CARTESIAN_POINT('Ctrl Pts',(6.56550075576078,-24.8967453140434,-10.2563848728767));
#41276=CARTESIAN_POINT('Ctrl Pts',(6.80321096137586,-24.9078900604581,-10.1002741921835));
#41277=CARTESIAN_POINT('Ctrl Pts',(7.03515431424307,-24.9190348068728,-9.936048209665));
#41278=CARTESIAN_POINT('Ctrl Pts',(7.1627874146331,-24.9251675048802,-9.84567842301525));
#41279=CARTESIAN_POINT('Ctrl Pts',(7.2886747830738,-24.9313002028877,-9.75285205462969));
#41280=CARTESIAN_POINT('Ctrl Pts',(7.41272179941101,-24.9374329008951,-9.65763976210217));
#41281=CARTESIAN_POINT('',(-12.1744999959752,-23.6251260039651,0.000313050724133792));
#41282=CARTESIAN_POINT('Ctrl Pts',(-12.1744999959752,-23.6251260039651,
0.000313050724133792));
#41283=CARTESIAN_POINT('Ctrl Pts',(-12.1745072760035,-23.6362300684397,
-0.28280626030774));
#41284=CARTESIAN_POINT('Ctrl Pts',(-12.1646342579426,-23.6473341329143,
-0.565958783664843));
#41285=CARTESIAN_POINT('Ctrl Pts',(-12.1449000764791,-23.6584381973888,
-0.848441148423234));
#41286=CARTESIAN_POINT('Ctrl Pts',(-12.1251680288802,-23.6695410611767,
-1.13089296825575));
#41287=CARTESIAN_POINT('Ctrl Pts',(-12.0955769658755,-23.6806439249646,
-1.41267450420121));
#41288=CARTESIAN_POINT('Ctrl Pts',(-12.0561980343215,-23.6917467887524,
-1.69308570581112));
#41289=CARTESIAN_POINT('Ctrl Pts',(-12.0168162232634,-23.7028504644146,
-1.97351741191864));
#41290=CARTESIAN_POINT('Ctrl Pts',(-11.9676451482731,-23.7139541400767,
-2.25257831493435));
#41291=CARTESIAN_POINT('Ctrl Pts',(-11.9088076155506,-23.7250578157389,
-2.52957534495496));
#41292=CARTESIAN_POINT('Ctrl Pts',(-11.8499700831609,-23.7361614913382,
-2.80657237340874));
#41293=CARTESIAN_POINT('Ctrl Pts',(-11.7814661517746,-23.7472651669375,
-3.08150526454602));
#41294=CARTESIAN_POINT('Ctrl Pts',(-11.7034695576592,-23.7583688425369,
-3.35369207932761));
#41295=CARTESIAN_POINT('Ctrl Pts',(-11.6254556305768,-23.7694749856753,
-3.62593938143092));
#41296=CARTESIAN_POINT('Ctrl Pts',(-11.5379448995412,-23.7805811288137,
-3.89543912724969));
#41297=CARTESIAN_POINT('Ctrl Pts',(-11.4411611446377,-23.7916872719521,
-4.16152398916932));
#41298=CARTESIAN_POINT('Ctrl Pts',(-11.3820531543148,-23.7984700404219,
-4.3240279285868));
#41299=CARTESIAN_POINT('Ctrl Pts',(-11.3194874657191,-23.8052528088917,
-4.48525848955029));
#41300=CARTESIAN_POINT('Ctrl Pts',(-11.2535239975975,-23.8120355773616,
-4.64506704854697));
#41301=CARTESIAN_POINT('Ctrl Pts',(-11.1451147212248,-23.8231828842355,
-4.90770833670762));
#41302=CARTESIAN_POINT('Ctrl Pts',(-11.027490726027,-23.8343301911093,-5.1665920149544));
#41303=CARTESIAN_POINT('Ctrl Pts',(-10.9009381361996,-23.8454774979832,
-5.42106982068579));
#41304=CARTESIAN_POINT('Ctrl Pts',(-10.7744070412407,-23.8566229114949,
-5.67550440354045));
#41305=CARTESIAN_POINT('Ctrl Pts',(-10.6389504981074,-23.8677683250065,
-5.9255343691766));
#41306=CARTESIAN_POINT('Ctrl Pts',(-10.4949015330221,-23.8789137385181,
-6.17053417964529));
#41307=CARTESIAN_POINT('Ctrl Pts',(-10.3508685595493,-23.8900579147204,
-6.41550679143171));
#41308=CARTESIAN_POINT('Ctrl Pts',(-10.1982452040525,-23.9012020909227,
-6.65545013324551));
#41309=CARTESIAN_POINT('Ctrl Pts',(-10.037409578847,-23.9123462671249,-6.88976481430757));
#41310=CARTESIAN_POINT('Ctrl Pts',(-9.87150892940053,-23.9238413949434,
-7.13145851688982));
#41311=CARTESIAN_POINT('Ctrl Pts',(-9.69687054816424,-23.9353365227619,
-7.36716304913461));
#41312=CARTESIAN_POINT('Ctrl Pts',(-9.51395741258113,-23.9468316505804,
-7.59625332658098));
#41313=CARTESIAN_POINT('Ctrl Pts',(-9.33661922343069,-23.957976422359,-7.8183612403992));
#41314=CARTESIAN_POINT('Ctrl Pts',(-9.1515033916188,-23.9691211941376,-8.03425189815682));
#41315=CARTESIAN_POINT('Ctrl Pts',(-8.95907314105923,-23.9802659659162,
-8.24338878757706));
#41316=CARTESIAN_POINT('Ctrl Pts',(-8.75756880151721,-23.9919362717546,
-8.4623875710529));
#41317=CARTESIAN_POINT('Ctrl Pts',(-8.54804383413787,-24.003606577593,-8.67398007541675));
#41318=CARTESIAN_POINT('Ctrl Pts',(-8.33107475358735,-24.0152768834315,
-8.87759222425425));
#41319=CARTESIAN_POINT('Ctrl Pts',(-8.11410567303683,-24.0269471892699,
-9.08120437309175));
#41320=CARTESIAN_POINT('Ctrl Pts',(-7.88969272996757,-24.0386174951083,
-9.27683594321905));
#41321=CARTESIAN_POINT('Ctrl Pts',(-7.65845451946485,-24.0502878009467,
-9.46395924670476));
#41322=CARTESIAN_POINT('Ctrl Pts',(-7.43757914943243,-24.0614351070725,
-9.64269670021316));
#41323=CARTESIAN_POINT('Ctrl Pts',(-7.21041084144513,-24.0725824131983,
-9.81372509541071));
#41324=CARTESIAN_POINT('Ctrl Pts',(-6.97751105217776,-24.0837297193241,
-9.97661213873413));
#41325=CARTESIAN_POINT('Ctrl Pts',(-6.74465082092712,-24.0948751320805,
-10.139471515702));
#41326=CARTESIAN_POINT('Ctrl Pts',(-6.50606127048044,-24.1060205448369,
-10.2941921487503));
#41327=CARTESIAN_POINT('Ctrl Pts',(-6.26233416579329,-24.1171659575934,
-10.4403841426424));
#41328=CARTESIAN_POINT('Ctrl Pts',(-6.01863411861028,-24.1283101330354,
-10.5865599069465));
#41329=CARTESIAN_POINT('Ctrl Pts',(-5.76979788477571,-24.1394543084775,
-10.7242087855524));
#41330=CARTESIAN_POINT('Ctrl Pts',(-5.51644430519778,-24.1505984839195,
-10.8529854177388));
#41331=CARTESIAN_POINT('Ctrl Pts',(-5.25511210174971,-24.1620936123039,
-10.9858174902043));
#41332=CARTESIAN_POINT('Ctrl Pts',(-4.9889736812031,-24.1735887406883,-11.1092093074788));
#41333=CARTESIAN_POINT('Ctrl Pts',(-4.71873469727067,-24.1850838690726,
-11.2228335596129));
#41334=CARTESIAN_POINT('Ctrl Pts',(-4.45673226505212,-24.196228640088,-11.3329946843513));
#41335=CARTESIAN_POINT('Ctrl Pts',(-4.19087578555295,-24.2073734111034,
-11.4339747257494));
#41336=CARTESIAN_POINT('Ctrl Pts',(-3.92182874309239,-24.2185181821189,
-11.5255242639914));
#41337=CARTESIAN_POINT('Ctrl Pts',(-3.64009468169887,-24.2301884891877,
-11.6213908566577));
#41338=CARTESIAN_POINT('Ctrl Pts',(-3.35486221345111,-24.2418587962565,
-11.7069160450841));
#41339=CARTESIAN_POINT('Ctrl Pts',(-3.06691227567061,-24.2535291033253,
-11.7818716400808));
#41340=CARTESIAN_POINT('Ctrl Pts',(-2.77896233789011,-24.2651994103942,
-11.8568272350776));
#41341=CARTESIAN_POINT('Ctrl Pts',(-2.48829525746922,-24.276869717463,-11.9212131606227));
#41342=CARTESIAN_POINT('Ctrl Pts',(-2.19570672218016,-24.2885400245318,
-11.9748620969167));
#41343=CARTESIAN_POINT('Ctrl Pts',(-1.91623044331381,-24.2996873307296,
-12.0261067742441));
#41344=CARTESIAN_POINT('Ctrl Pts',(-1.63491767399143,-24.3108346369273,
-12.0675709631649));
#41345=CARTESIAN_POINT('Ctrl Pts',(-1.35246828020352,-24.3219819431251,
-12.0991437631364));
#41346=CARTESIAN_POINT('Ctrl Pts',(-1.07006686043228,-24.3331273559534,
-12.1307112004694));
#41347=CARTESIAN_POINT('Ctrl Pts',(-0.786529466626631,-24.3442727687817,
-12.1523905734547));
#41348=CARTESIAN_POINT('Ctrl Pts',(-0.502562287985962,-24.35541818161,-12.1641227138127));
#41349=CARTESIAN_POINT('Ctrl Pts',(-0.21862663413152,-24.3665623571237,
-12.1758535517201));
#41350=CARTESIAN_POINT('Ctrl Pts',(0.065738442831518,-24.3777065326373,
-12.1776393510993));
#41351=CARTESIAN_POINT('Ctrl Pts',(0.349824290944202,-24.388850708151,-12.1694730048374));
#41352=CARTESIAN_POINT('Ctrl Pts',(0.642856581842261,-24.4003458364815,
-12.1610494836753));
#41353=CARTESIAN_POINT('Ctrl Pts',(0.935591475061994,-24.411840964812,-12.1420368316068));
#41354=CARTESIAN_POINT('Ctrl Pts',(1.22725272951179,-24.4233360931425,-12.1124853348892));
#41355=CARTESIAN_POINT('Ctrl Pts',(1.51002451090377,-24.4344808642279,-12.0838345311155));
#41356=CARTESIAN_POINT('Ctrl Pts',(1.79178685310204,-24.4456256353134,-12.0452778196724));
#41357=CARTESIAN_POINT('Ctrl Pts',(2.0718378161832,-24.4567704063989,-11.9969136995076));
#41358=CARTESIAN_POINT('Ctrl Pts',(2.36509468764143,-24.4684407133519,-11.9462689510864));
#41359=CARTESIAN_POINT('Ctrl Pts',(2.65647458170125,-24.4801110203049,-11.8848696481262));
#41360=CARTESIAN_POINT('Ctrl Pts',(2.9451825869511,-24.4917813272579,-11.812889137697));
#41361=CARTESIAN_POINT('Ctrl Pts',(3.23389059220094,-24.5034516342109,-11.7409086272678));
#41362=CARTESIAN_POINT('Ctrl Pts',(3.51992638522858,-24.5151219411639,-11.6583469990493));
#41363=CARTESIAN_POINT('Ctrl Pts',(3.80251123137941,-24.5267922481169,-11.5654381060656));
#41364=CARTESIAN_POINT('Ctrl Pts',(4.07242967029088,-24.5379394524956,-11.4766937034667));
#41365=CARTESIAN_POINT('Ctrl Pts',(4.33928034053855,-24.5490866568743,-11.3784827372588));
#41366=CARTESIAN_POINT('Ctrl Pts',(4.6023956623735,-24.5602338612531,-11.2710427386718));
#41367=CARTESIAN_POINT('Ctrl Pts',(4.86547585228003,-24.5713795772244,-11.163617085788));
#41368=CARTESIAN_POINT('Ctrl Pts',(5.12482144211058,-24.5825252931958,-11.0469649602304));
#41369=CARTESIAN_POINT('Ctrl Pts',(5.37978398500469,-24.5936710091671,-10.9213723736849));
#41370=CARTESIAN_POINT('Ctrl Pts',(5.6347135872906,-24.6048152851361,-10.7957960134295));
#41371=CARTESIAN_POINT('Ctrl Pts',(5.8852610344657,-24.6159595611051,-10.6612816171815));
#41372=CARTESIAN_POINT('Ctrl Pts',(6.13080066714201,-24.6271038370741,-10.5181620747054));
#41373=CARTESIAN_POINT('Ctrl Pts',(6.37634730179191,-24.6382484308407,-10.375038450936));
#41374=CARTESIAN_POINT('Ctrl Pts',(6.61688560493623,-24.6493930246074,-10.2233093229305));
#41375=CARTESIAN_POINT('Ctrl Pts',(6.85181594527438,-24.6605376183741,-10.0633527465792));
#41376=CARTESIAN_POINT('Ctrl Pts',(7.04258417037973,-24.6695872556807,-9.93346474607435));
#41377=CARTESIAN_POINT('Ctrl Pts',(7.22965507309842,-24.6786368929874,-9.79815263546583));
#41378=CARTESIAN_POINT('Ctrl Pts',(7.41272179941105,-24.687686530294,-9.65763976210214));
#41379=CARTESIAN_POINT('Ctrl Pts',(7.41324263166141,-21.6876995907947,-9.65831743152016));
#41380=CARTESIAN_POINT('Ctrl Pts',(8.88409813246325,-21.7604723234234,-8.52773514691198));
#41381=CARTESIAN_POINT('Ctrl Pts',(11.414685028869,-21.9126624639138,-5.45082711782888));
#41382=CARTESIAN_POINT('Ctrl Pts',(12.6811956770552,-22.1442700122659,0.50872888397338));
#41383=CARTESIAN_POINT('Ctrl Pts',(10.8914562364704,-22.382522235851,6.51518676137968));
#41384=CARTESIAN_POINT('Ctrl Pts',(6.4456037215397,-22.6207744594361,10.9327814560358));
#41385=CARTESIAN_POINT('Ctrl Pts',(0.427851551046576,-22.8590266830212,
12.6841806328137));
#41386=CARTESIAN_POINT('Ctrl Pts',(-5.69424089117864,-23.0972789066063,
11.3422716237698));
#41387=CARTESIAN_POINT('Ctrl Pts',(-10.4276708680614,-23.3355311301914,
7.23430593172712));
#41388=CARTESIAN_POINT('Ctrl Pts',(-12.0452929662932,-23.5114801626443,
2.89768759261325));
#41389=CARTESIAN_POINT('Ctrl Pts',(-12.1750513728812,-23.6080117872355,
0.436676266174656));
#41390=CARTESIAN_POINT('Ctrl Pts',(-12.1746001704992,-23.6251260039651,
0.000313053299986626));
#41391=CARTESIAN_POINT('Ctrl Pts',(7.93208051261574,-20.0005837734501,-6.87965285147223));
#41392=CARTESIAN_POINT('Ctrl Pts',(9.07668263151754,-20.0800217251941,-5.55995978932681));
#41393=CARTESIAN_POINT('Ctrl Pts',(10.6930139230921,-20.2388770847998,-2.33991560351307));
#41394=CARTESIAN_POINT('Ctrl Pts',(10.5082240576505,-20.4771498522672,3.06359191036739));
#41395=CARTESIAN_POINT('Ctrl Pts',(7.7610444220363,-20.7154020758523,7.71831352629605));
#41396=CARTESIAN_POINT('Ctrl Pts',(3.12105089944607,-20.9536542994374,10.4913407524211));
#41397=CARTESIAN_POINT('Ctrl Pts',(-2.28002032107308,-21.1919065230225,
10.7055409903604));
#41398=CARTESIAN_POINT('Ctrl Pts',(-7.12508829170954,-21.4301587466076,
8.30910926435329));
#41399=CARTESIAN_POINT('Ctrl Pts',(-10.2325364964883,-21.6684109701927,
3.88625151956404));
#41400=CARTESIAN_POINT('Ctrl Pts',(-10.8445684035224,-21.9066631937778,
-1.48431630400502));
#41401=CARTESIAN_POINT('Ctrl Pts',(-8.81191628458542,-22.1449154173629,
-6.49291954617506));
#41402=CARTESIAN_POINT('Ctrl Pts',(-4.63029122950666,-22.383167640948,-9.91807630779845));
#41403=CARTESIAN_POINT('Ctrl Pts',(0.680530483683632,-22.6214198645331,
-10.9245019479025));
#41404=CARTESIAN_POINT('Ctrl Pts',(5.82538981214024,-22.8596720881182,-9.26675138990805));
#41405=CARTESIAN_POINT('Ctrl Pts',(9.54960316733972,-23.0979243117033,-5.34910593878247));
#41406=CARTESIAN_POINT('Ctrl Pts',(10.9449409563647,-23.3361765352884,-0.126965784354505));
#41407=CARTESIAN_POINT('Ctrl Pts',(9.67112030848427,-23.5744287588735,5.12613742673736));
#41408=CARTESIAN_POINT('Ctrl Pts',(6.03878961601207,-23.8126809824586,9.12912226706514));
#41409=CARTESIAN_POINT('Ctrl Pts',(0.933770628914186,-24.0509332060437,
10.9057748640797));
#41410=CARTESIAN_POINT('Ctrl Pts',(-4.3989683509955,-24.2891854296288,10.0228204950036));
#41411=CARTESIAN_POINT('Ctrl Pts',(-8.65892458966233,-24.5274376532139,
6.69558646125051));
#41412=CARTESIAN_POINT('Ctrl Pts',(-10.8072164379082,-24.765689876799,1.7354901366115));
#41413=CARTESIAN_POINT('Ctrl Pts',(-10.3199368707579,-25.0039421003841,
-3.64784266760709));
#41414=CARTESIAN_POINT('Ctrl Pts',(-7.31591945824722,-25.2421943239692,
-8.14157083244356));
#41415=CARTESIAN_POINT('Ctrl Pts',(-2.52775824622543,-25.4804465475543,
-10.6498024110112));
#41416=CARTESIAN_POINT('Ctrl Pts',(2.8768510043701,-25.7186987711394,-10.5608513596116));
#41417=CARTESIAN_POINT('Ctrl Pts',(7.5798784633816,-25.9569509947245,-7.89641029984006));
#41418=CARTESIAN_POINT('Ctrl Pts',(10.4343900608802,-26.1952032183096,-3.30626030429192));
#41419=CARTESIAN_POINT('Ctrl Pts',(10.7442519485492,-26.4334554418947,2.09019214633302));
#41420=CARTESIAN_POINT('Ctrl Pts',(8.43389766221118,-26.6717076654798,6.97690643235821));
#41421=CARTESIAN_POINT('Ctrl Pts',(4.06675662420537,-26.9099598890649,10.1621525132199));
#41422=CARTESIAN_POINT('Ctrl Pts',(-1.29215020014935,-27.14821211265,10.8691398464998));
#41423=CARTESIAN_POINT('Ctrl Pts',(-6.33593849695176,-27.3864643362351,
8.92545441450063));
#41424=CARTESIAN_POINT('Ctrl Pts',(-9.83457236079029,-27.6247165598202,
4.80510557874393));
#41425=CARTESIAN_POINT('Ctrl Pts',(-10.934834919905,-27.8629687834053,-0.487071264723974));
#41426=CARTESIAN_POINT('Ctrl Pts',(-9.36840356171729,-28.1012210069904,
-5.66046533840602));
#41427=CARTESIAN_POINT('Ctrl Pts',(-5.51728615423312,-28.3394732305755,
-9.45343358969647));
#41428=CARTESIAN_POINT('Ctrl Pts',(-0.320660237907371,-28.5777254541606,
-10.9409793964854));
#41429=CARTESIAN_POINT('Ctrl Pts',(4.95416555177833,-28.8159776777457,-9.76033282363192));
#41430=CARTESIAN_POINT('Ctrl Pts',(9.02081186376675,-29.0542299013308,-6.1994198487454));
#41431=CARTESIAN_POINT('Ctrl Pts',(10.8875398137095,-29.2924821249159,-1.12664543996017));
#41432=CARTESIAN_POINT('Ctrl Pts',(10.0991077719128,-29.530734348501,4.22088561249689));
#41433=CARTESIAN_POINT('Ctrl Pts',(6.84779179425367,-29.7689865720861,8.53906322057902));
#41434=CARTESIAN_POINT('Ctrl Pts',(1.92649498392104,-30.0072387956712,10.7748072010324));
#41435=CARTESIAN_POINT('Ctrl Pts',(-3.46461892863269,-30.2454910192563,
10.3828834541207));
#41436=CARTESIAN_POINT('Ctrl Pts',(-8.0108112405926,-30.4837432428414,7.45887098762869));
#41437=CARTESIAN_POINT('Ctrl Pts',(-10.6033954949622,-30.7219954664265,
2.71585292678186));
#41438=CARTESIAN_POINT('Ctrl Pts',(-10.6101144412331,-30.9602476900116,
-2.68948409298712));
#41439=CARTESIAN_POINT('Ctrl Pts',(-8.02932952031574,-31.1984999135967,
-7.43893275925249));
#41440=CARTESIAN_POINT('Ctrl Pts',(-3.49042046230085,-31.4367521371818,
-10.3742381955904));
#41441=CARTESIAN_POINT('Ctrl Pts',(1.89970245342874,-31.6750043607669,-10.7795632439784));
#41442=CARTESIAN_POINT('Ctrl Pts',(6.8265421998787,-31.913256584352,-8.55606070196843));
#41443=CARTESIAN_POINT('Ctrl Pts',(10.0885832827944,-32.1515088079371,-4.24597933209919));
#41444=CARTESIAN_POINT('Ctrl Pts',(10.8903070521443,-32.3897610315222,1.09957512363163));
#41445=CARTESIAN_POINT('Ctrl Pts',(9.03619597933803,-32.6280132551074,6.1769746126635));
#41446=CARTESIAN_POINT('Ctrl Pts',(4.97841479809776,-32.8662654786924,9.7479864197984));
#41447=CARTESIAN_POINT('Ctrl Pts',(-0.293459559412273,-33.1045177022776,
10.9417427601586));
#41448=CARTESIAN_POINT('Ctrl Pts',(-5.49376751214475,-33.3427699258626,
9.46712055827954));
#41449=CARTESIAN_POINT('Ctrl Pts',(-9.35430248110292,-33.5810221494478,
5.68373805118744));
#41450=CARTESIAN_POINT('Ctrl Pts',(-10.9335902515748,-33.8192743730328,
0.514254171769246));
#41451=CARTESIAN_POINT('Ctrl Pts',(-9.84648764379592,-34.0575265966179,
-4.78064161206769));
#41452=CARTESIAN_POINT('Ctrl Pts',(-6.35810793409936,-34.295778820203,-8.90967545092837));
#41453=CARTESIAN_POINT('Ctrl Pts',(-1.3191672989035,-34.5340310437881,-10.8658939245695));
#41454=CARTESIAN_POINT('Ctrl Pts',(4.04148056253829,-34.7722832673732,-10.1722312205807));
#41455=CARTESIAN_POINT('Ctrl Pts',(8.41652674720532,-35.0105354909583,-6.9978518601521));
#41456=CARTESIAN_POINT('Ctrl Pts',(10.7390224500958,-35.2487877145434,-2.11689630296171));
#41457=CARTESIAN_POINT('Ctrl Pts',(10.4425773045532,-35.4870399381285,3.28030979990781));
#41458=CARTESIAN_POINT('Ctrl Pts',(7.59948581375965,-35.7252921617136,7.87754203452586));
#41459=CARTESIAN_POINT('Ctrl Pts',(2.90309678978814,-35.9635443852987,10.5536667643604));
#41460=CARTESIAN_POINT('Ctrl Pts',(-2.50127462534687,-36.2017966088839,
10.6560536034062));
#41461=CARTESIAN_POINT('Ctrl Pts',(-7.29565659631146,-36.4400488324689,
8.15973332519128));
#41462=CARTESIAN_POINT('Ctrl Pts',(-10.310836309689,-36.678301056054,3.67348714751024));
#41463=CARTESIAN_POINT('Ctrl Pts',(-10.811497527272,-36.9165532796391,-1.70861762580354));
#41464=CARTESIAN_POINT('Ctrl Pts',(-8.67554332886272,-37.1548055032242,
-6.67403935727874));
#41465=CARTESIAN_POINT('Ctrl Pts',(-4.42387183430699,-37.3930577268093,
-10.0118535213315));
#41466=CARTESIAN_POINT('Ctrl Pts',(0.906655509484174,-37.6313099503944,
-10.9080625518847));
#41467=CARTESIAN_POINT('Ctrl Pts',(6.01607574523276,-37.8695621739795,-9.14410671556304));
#41468=CARTESIAN_POINT('Ctrl Pts',(9.65834638546719,-38.1078143975646,-5.15016435505535));
#41469=CARTESIAN_POINT('Ctrl Pts',(10.9452233105833,-38.3460666211498,0.0997558540279738));
#41470=CARTESIAN_POINT('Ctrl Pts',(9.56287066352807,-38.5843188447348,5.32534873881454));
#41471=CARTESIAN_POINT('Ctrl Pts',(5.84841145753923,-38.82257106832,9.25224060771052));
#41472=CARTESIAN_POINT('Ctrl Pts',(0.70768278248567,-39.060823291905,10.9227763791256));
#41473=CARTESIAN_POINT('Ctrl Pts',(-4.60561153353682,-39.2990755154902,
9.92955670850569));
#41474=CARTESIAN_POINT('Ctrl Pts',(-8.79576482446728,-39.5373277390752,
6.51480629675831));
#41475=CARTESIAN_POINT('Ctrl Pts',(-10.8408098726847,-39.7755799626604,
1.51127160533644));
#41476=CARTESIAN_POINT('Ctrl Pts',(-10.2422364118163,-40.0138321862454,
-3.86080079579494));
#41477=CARTESIAN_POINT('Ctrl Pts',(-7.14558203450444,-40.2520844098305,
-8.29137091192963));
#41478=CARTESIAN_POINT('Ctrl Pts',(-2.30691296609827,-40.4903366334156,
-10.6998374196014));
#41479=CARTESIAN_POINT('Ctrl Pts',(3.09555850011698,-40.7285888570008,-10.4990832245953));
#41480=CARTESIAN_POINT('Ctrl Pts',(6.19188889114854,-40.8874236727241,-8.65783810040184));
#41481=CARTESIAN_POINT('Ctrl Pts',(7.42649694513297,-40.9668410805858,-7.4225782431051));
#41482=CARTESIAN_POINT('Ctrl Pts',(8.35397305039485,-19.6781514844946,-7.24556872889312));
#41483=CARTESIAN_POINT('Ctrl Pts',(9.5594544167933,-19.7575894362386,-5.8556836592167));
#41484=CARTESIAN_POINT('Ctrl Pts',(11.2617553489193,-19.9164447958441,-2.46437134127127));
#41485=CARTESIAN_POINT('Ctrl Pts',(11.0671368558985,-20.1547175633116,3.22653863837005));
#41486=CARTESIAN_POINT('Ctrl Pts',(8.17383986981593,-20.3929697868966,8.12883619759329));
#41487=CARTESIAN_POINT('Ctrl Pts',(3.28705376368968,-20.6312220104818,11.0493555592179));
#41488=CARTESIAN_POINT('Ctrl Pts',(-2.40129034069979,-20.8694742340669,
11.2749487074831));
#41489=CARTESIAN_POINT('Ctrl Pts',(-7.5040584214893,-21.107726457652,8.75105525678824));
#41490=CARTESIAN_POINT('Ctrl Pts',(-10.776785988605,-21.345978681237,4.0929539746676));
#41491=CARTESIAN_POINT('Ctrl Pts',(-11.4213707289154,-21.5842309048222,
-1.5632643140974));
#41492=CARTESIAN_POINT('Ctrl Pts',(-9.28060564270375,-21.8224831284072,
-6.83826580187362));
#41493=CARTESIAN_POINT('Ctrl Pts',(-4.87656776620671,-22.0607353519924,
-10.4456002501902));
#41494=CARTESIAN_POINT('Ctrl Pts',(0.716726628231168,-22.2989875755774,
-11.505555789129));
#41495=CARTESIAN_POINT('Ctrl Pts',(6.13523140886729,-22.5372397991626,-9.75963257721301));
#41496=CARTESIAN_POINT('Ctrl Pts',(10.0575287120496,-22.7754920227476,-5.63361488643787));
#41497=CARTESIAN_POINT('Ctrl Pts',(11.5270819102518,-23.0137442463328,-0.133718857131222));
#41498=CARTESIAN_POINT('Ctrl Pts',(10.1855091228218,-23.2519964699178,5.39878709595479));
#41499=CARTESIAN_POINT('Ctrl Pts',(6.35998154947282,-23.490248693503,9.61468321854845));
#41500=CARTESIAN_POINT('Ctrl Pts',(0.983436143492576,-23.7285009170881,
11.4858326467177));
#41501=CARTESIAN_POINT('Ctrl Pts',(-4.63294125611917,-23.9667531406732,
10.5559155849508));
#41502=CARTESIAN_POINT('Ctrl Pts',(-9.119476605462,-24.2050053642583,7.05171219138697));
#41503=CARTESIAN_POINT('Ctrl Pts',(-11.3820320820593,-24.4432575878434,
1.82779761342809));
#41504=CARTESIAN_POINT('Ctrl Pts',(-10.868835025435,-24.6815098114284,-3.84186460145004));
#41505=CARTESIAN_POINT('Ctrl Pts',(-7.70503954112061,-24.9197620350136,
-8.57460576880672));
#41506=CARTESIAN_POINT('Ctrl Pts',(-2.66220498308041,-25.1580142585986,
-11.216245497271));
#41507=CARTESIAN_POINT('Ctrl Pts',(3.02986533259278,-25.3962664821838,-11.1225633056928));
#41508=CARTESIAN_POINT('Ctrl Pts',(7.98303803241107,-25.6345187057688,-8.31640560566758));
#41509=CARTESIAN_POINT('Ctrl Pts',(10.9893757668322,-25.872770929354,-3.48211411063157));
#41510=CARTESIAN_POINT('Ctrl Pts',(11.3157186291889,-26.1110231529391,2.20136556012525));
#41511=CARTESIAN_POINT('Ctrl Pts',(8.88248091630454,-26.3492753765242,7.34799504598405));
#41512=CARTESIAN_POINT('Ctrl Pts',(4.28305980846921,-26.5875276001093,10.702658412811));
#41513=CARTESIAN_POINT('Ctrl Pts',(-1.3608772543271,-26.8257798236944,11.4472490810218));
#41514=CARTESIAN_POINT('Ctrl Pts',(-6.67293522403238,-27.0640320472795,
9.4001826535517));
#41515=CARTESIAN_POINT('Ctrl Pts',(-10.3576548843057,-27.3022842708645,
5.06068016396008));
#41516=CARTESIAN_POINT('Ctrl Pts',(-11.5164383526005,-27.5405364944497,
-0.512977674981265));
#41517=CARTESIAN_POINT('Ctrl Pts',(-9.86669143805761,-27.7787887180348,
-5.96153491061126));
#41518=CARTESIAN_POINT('Ctrl Pts',(-5.8107402932274,-28.0170409416198,-9.95624405430786));
#41519=CARTESIAN_POINT('Ctrl Pts',(-0.337715556662699,-28.255293165205,
-11.5229096424065));
#41520=CARTESIAN_POINT('Ctrl Pts',(5.21766835837407,-28.49354538879,-10.2794666849161));
#41521=CARTESIAN_POINT('Ctrl Pts',(9.50061198732568,-28.7317976123752,-6.52915540407486));
#41522=CARTESIAN_POINT('Ctrl Pts',(11.4666277080989,-28.9700498359603,-1.1865696052641));
#41523=CARTESIAN_POINT('Ctrl Pts',(10.6362604395415,-29.2083020595454,4.44538662958811));
#41524=CARTESIAN_POINT('Ctrl Pts',(7.21201304158794,-29.4465542831305,8.99324003417244));
#41525=CARTESIAN_POINT('Ctrl Pts',(2.02896165158692,-29.6848065067157,11.3478990584454));
#41526=CARTESIAN_POINT('Ctrl Pts',(-3.64889553423618,-29.9230587303007,
10.9351296199225));
#41527=CARTESIAN_POINT('Ctrl Pts',(-8.43689131864875,-30.1613109538859,
7.85559439518017));
#41528=CARTESIAN_POINT('Ctrl Pts',(-11.1673702840897,-30.3995631774709,
2.86030406815548));
#41529=CARTESIAN_POINT('Ctrl Pts',(-11.1744465985554,-30.637815401056,-2.83253272537331));
#41530=CARTESIAN_POINT('Ctrl Pts',(-8.45639455106058,-30.8760676246411,
-7.83459568970025));
#41531=CARTESIAN_POINT('Ctrl Pts',(-3.67606940325828,-31.1143198482261,
-10.9260245362485));
#41532=CARTESIAN_POINT('Ctrl Pts',(2.00074407647172,-31.3525720718113,-11.3529080664269));
#41533=CARTESIAN_POINT('Ctrl Pts',(7.18963322100266,-31.5908242953964,-9.01114157982946));
#41534=CARTESIAN_POINT('Ctrl Pts',(10.6251761725167,-31.8290765189815,-4.47181503723706));
#41535=CARTESIAN_POINT('Ctrl Pts',(11.4695421307741,-32.0673287425667,1.15805946940319));
#41536=CARTESIAN_POINT('Ctrl Pts',(9.51681435525202,-32.3055809661518,6.50551634783486));
#41537=CARTESIAN_POINT('Ctrl Pts',(5.24320737678452,-32.5438331897368,10.2664635989375));
#41538=CARTESIAN_POINT('Ctrl Pts',(-0.309068124915233,-32.7820854133219,
11.5237136079667));
#41539=CARTESIAN_POINT('Ctrl Pts',(-5.78597073852161,-33.0203376369069,
9.97065900716958));
#41540=CARTESIAN_POINT('Ctrl Pts',(-9.85184034731961,-33.2585898604922,
5.98604545548992));
#41541=CARTESIAN_POINT('Ctrl Pts',(-11.515127482688,-33.4968420840772,0.541606390048691));
#41542=CARTESIAN_POINT('Ctrl Pts',(-10.3702039189452,-33.7350943076624,
-5.03491500461833));
#41543=CARTESIAN_POINT('Ctrl Pts',(-6.69628381210821,-33.9733465312474,
-9.38356443639719));
#41544=CARTESIAN_POINT('Ctrl Pts',(-1.3893313420703,-34.2115987548325,-11.4438305145706));
#41545=CARTESIAN_POINT('Ctrl Pts',(4.25643936032185,-34.4498509784176,-10.7132731877799));
#41546=CARTESIAN_POINT('Ctrl Pts',(8.8641860747949,-34.6881032020028,-7.37005452193625));
#41547=CARTESIAN_POINT('Ctrl Pts',(11.3102109834865,-34.9263554255878,-2.22949006093621));
#41548=CARTESIAN_POINT('Ctrl Pts',(10.9979984746946,-35.1646076491729,3.45478334741955));
#41549=CARTESIAN_POINT('Ctrl Pts',(8.00368826111052,-35.402859872758,8.29653377258524));
#41550=CARTESIAN_POINT('Ctrl Pts',(3.05750708228506,-35.6411120963432,11.114996575248));
#41551=CARTESIAN_POINT('Ctrl Pts',(-2.63431274790397,-35.8793643199282,
11.2228291789063));
#41552=CARTESIAN_POINT('Ctrl Pts',(-7.68369893542883,-36.1176165435133,
8.59373429059882));
#41553=CARTESIAN_POINT('Ctrl Pts',(-10.8592504225313,-36.3558687670984,
3.86887306331091));
#41554=CARTESIAN_POINT('Ctrl Pts',(-11.3865408745652,-36.5941209906835,
-1.79949580399373));
#41555=CARTESIAN_POINT('Ctrl Pts',(-9.13697926434082,-36.8323732142686,
-7.02901903722545));
#41556=CARTESIAN_POINT('Ctrl Pts',(-4.65916930916454,-37.0706254378537,
-10.544365298446));
#41557=CARTESIAN_POINT('Ctrl Pts',(0.954878821536958,-37.3088776614388,
-11.4882420123614));
#41558=CARTESIAN_POINT('Ctrl Pts',(6.33605957035795,-37.5471298850239,-9.63046466185671));
#41559=CARTESIAN_POINT('Ctrl Pts',(10.1720557787132,-37.785382108609,-5.42409197168482));
#41560=CARTESIAN_POINT('Ctrl Pts',(11.5273792823635,-38.0236343321941,0.105061681464705));
#41561=CARTESIAN_POINT('Ctrl Pts',(10.0715018815638,-38.2618865557792,5.60859408540474));
#41562=CARTESIAN_POINT('Ctrl Pts',(6.15947753255869,-38.5001387793643,9.74434999363035));
#41563=CARTESIAN_POINT('Ctrl Pts',(0.74532310706011,-38.7383910029494,11.5037384405739));
#41564=CARTESIAN_POINT('Ctrl Pts',(-4.85057540333342,-38.9766432265345,
10.4576912719547));
#41565=CARTESIAN_POINT('Ctrl Pts',(-9.26359511660826,-39.2148954501196,
6.86131666781508));
#41566=CARTESIAN_POINT('Ctrl Pts',(-11.4174122888469,-39.4531476737047,
1.59165331752844));
#41567=CARTESIAN_POINT('Ctrl Pts',(-10.7870018243007,-39.6913998972898,
-4.06614957446744));
#41568=CARTESIAN_POINT('Ctrl Pts',(-7.52564218816163,-39.9296521208749,
-8.73237343455132));
#41569=CARTESIAN_POINT('Ctrl Pts',(-2.42961335525277,-40.16790434446,-11.268941774455));
#41570=CARTESIAN_POINT('Ctrl Pts',(3.26020547128437,-40.4061565680451,-11.0575098390168));
#41571=CARTESIAN_POINT('Ctrl Pts',(6.52122388891844,-40.5649913837685,-9.11833232786835));
#41572=CARTESIAN_POINT('Ctrl Pts',(7.82149843786967,-40.6444087916302,-7.81737130740481));
#41573=CARTESIAN_POINT('Ctrl Pts',(8.77586558817396,-19.3557191955389,-7.61148460631401));
#41574=CARTESIAN_POINT('Ctrl Pts',(10.0422262020691,-19.4351571472829,-6.15140752910658));
#41575=CARTESIAN_POINT('Ctrl Pts',(11.8304967747464,-19.5940125068886,-2.58882707902948));
#41576=CARTESIAN_POINT('Ctrl Pts',(11.6260496541463,-19.832285274356,3.38948536637273));
#41577=CARTESIAN_POINT('Ctrl Pts',(8.58663531759557,-20.0705374979411,8.53935886889055));
#41578=CARTESIAN_POINT('Ctrl Pts',(3.45305662793327,-20.3087897215262,11.6073703660148));
#41579=CARTESIAN_POINT('Ctrl Pts',(-2.52256036032647,-20.5470419451113,
11.8443564246056));
#41580=CARTESIAN_POINT('Ctrl Pts',(-7.8830285512691,-20.7852941686964,9.1930012492232));
#41581=CARTESIAN_POINT('Ctrl Pts',(-11.3210354807218,-21.0235463922815,
4.29965642977116));
#41582=CARTESIAN_POINT('Ctrl Pts',(-11.9981730543084,-21.2617986158666,
-1.64221232418978));
#41583=CARTESIAN_POINT('Ctrl Pts',(-9.74929500082207,-21.5000508394517,
-7.18361205757219));
#41584=CARTESIAN_POINT('Ctrl Pts',(-5.12284430290676,-21.7383030630368,
-10.973124192582));
#41585=CARTESIAN_POINT('Ctrl Pts',(0.752922772778706,-21.9765552866219,
-12.0866096303555));
#41586=CARTESIAN_POINT('Ctrl Pts',(6.44507300559435,-22.214807510207,-10.2525137645179));
#41587=CARTESIAN_POINT('Ctrl Pts',(10.5654542567593,-22.4530597337921,-5.91812383409328));
#41588=CARTESIAN_POINT('Ctrl Pts',(12.1092228641389,-22.6913119573772,-0.140471929907933));
#41589=CARTESIAN_POINT('Ctrl Pts',(10.6998979371592,-22.9295641809623,5.67143676517222));
#41590=CARTESIAN_POINT('Ctrl Pts',(6.6811734829336,-23.1678164045474,10.1002441700318));
#41591=CARTESIAN_POINT('Ctrl Pts',(1.03310165807095,-23.4060686281325,12.0658904293558));
#41592=CARTESIAN_POINT('Ctrl Pts',(-4.86691416124282,-23.6443208517176,
11.089010674898));
#41593=CARTESIAN_POINT('Ctrl Pts',(-9.58002862126169,-23.8825730753027,
7.40783792152343));
#41594=CARTESIAN_POINT('Ctrl Pts',(-11.9568477262104,-24.1208252988878,
1.92010509024468));
#41595=CARTESIAN_POINT('Ctrl Pts',(-11.4177331801119,-24.3590775224729,
-4.03588653529299));
#41596=CARTESIAN_POINT('Ctrl Pts',(-8.094159623994,-24.597329746058,-9.00764070516989));
#41597=CARTESIAN_POINT('Ctrl Pts',(-2.79665171993538,-24.8355819696431,
-11.7826885835309));
#41598=CARTESIAN_POINT('Ctrl Pts',(3.18287966081545,-25.0738341932282,-11.6842752517741));
#41599=CARTESIAN_POINT('Ctrl Pts',(8.38619760144056,-25.3120864168133,-8.73640091149512));
#41600=CARTESIAN_POINT('Ctrl Pts',(11.5443614727842,-25.5503386403984,-3.65796791697122));
#41601=CARTESIAN_POINT('Ctrl Pts',(11.8871853098286,-25.7885908639836,2.3125389739175));
#41602=CARTESIAN_POINT('Ctrl Pts',(9.33106417039787,-26.0268430875686,7.71908365960986));
#41603=CARTESIAN_POINT('Ctrl Pts',(4.49936299273306,-26.2650953111537,11.2431643124021));
#41604=CARTESIAN_POINT('Ctrl Pts',(-1.42960430850484,-26.5033475347388,
12.0253583155439));
#41605=CARTESIAN_POINT('Ctrl Pts',(-7.00993195111297,-26.7415997583239,
9.87491089260277));
#41606=CARTESIAN_POINT('Ctrl Pts',(-10.880737407821,-26.979851981909,5.31625474917623));
#41607=CARTESIAN_POINT('Ctrl Pts',(-12.098041785296,-27.2181042054941,-0.538884085238557));
#41608=CARTESIAN_POINT('Ctrl Pts',(-10.3649793143979,-27.4563564290792,
-6.26260448281651));
#41609=CARTESIAN_POINT('Ctrl Pts',(-6.10419443222168,-27.6946086526643,
-10.4590545189192));
#41610=CARTESIAN_POINT('Ctrl Pts',(-0.354770875418025,-27.9328608762494,
-12.1048398883276));
#41611=CARTESIAN_POINT('Ctrl Pts',(5.4811711649698,-28.1711130998345,-10.7986005462002));
#41612=CARTESIAN_POINT('Ctrl Pts',(9.98041211088462,-28.4093653234196,-6.85889095940433));
#41613=CARTESIAN_POINT('Ctrl Pts',(12.0457156024881,-28.6476175470047,-1.24649377056803));
#41614=CARTESIAN_POINT('Ctrl Pts',(11.1734131071702,-28.8858697705898,4.66988764667932));
#41615=CARTESIAN_POINT('Ctrl Pts',(7.57623428892219,-29.1241219941749,9.44741684776586));
#41616=CARTESIAN_POINT('Ctrl Pts',(2.13142831925279,-29.36237421776,11.9209909158584));
#41617=CARTESIAN_POINT('Ctrl Pts',(-3.83317213983967,-29.6006264413451,
11.4873757857244));
#41618=CARTESIAN_POINT('Ctrl Pts',(-8.86297139670491,-29.8388786649302,
8.25231780273166));
#41619=CARTESIAN_POINT('Ctrl Pts',(-11.7313450732173,-30.0771308885153,
3.00475520952911));
#41620=CARTESIAN_POINT('Ctrl Pts',(-11.7387787558777,-30.3153831121004,
-2.97558135775951));
#41621=CARTESIAN_POINT('Ctrl Pts',(-8.88345958180541,-30.5536353356855,
-8.23025862014802));
#41622=CARTESIAN_POINT('Ctrl Pts',(-3.86171834421572,-30.7918875592706,
-11.4778108769068));
#41623=CARTESIAN_POINT('Ctrl Pts',(2.10178569951469,-31.0301397828557,-11.9262528888754));
#41624=CARTESIAN_POINT('Ctrl Pts',(7.55272424212662,-31.2683920064408,-9.46622245769049));
#41625=CARTESIAN_POINT('Ctrl Pts',(11.1617690622389,-31.5066442300259,-4.69765074237494));
#41626=CARTESIAN_POINT('Ctrl Pts',(12.0487772094039,-31.744896453611,1.21654381517477));
#41627=CARTESIAN_POINT('Ctrl Pts',(9.99743273116598,-31.9831486771961,6.83405808300621));
#41628=CARTESIAN_POINT('Ctrl Pts',(5.50799995547128,-32.2214009007812,10.7849407780765));
#41629=CARTESIAN_POINT('Ctrl Pts',(-0.324676690418206,-32.4596531243664,
12.1056844557749));
#41630=CARTESIAN_POINT('Ctrl Pts',(-6.07817396489844,-32.6979053479514,
10.4741974560597));
#41631=CARTESIAN_POINT('Ctrl Pts',(-10.3493782135363,-32.9361575715365,
6.28835285979241));
#41632=CARTESIAN_POINT('Ctrl Pts',(-12.0966647138013,-33.1744097951216,
0.568958608328141));
#41633=CARTESIAN_POINT('Ctrl Pts',(-10.8939201940946,-33.4126620187067,
-5.28918839716898));
#41634=CARTESIAN_POINT('Ctrl Pts',(-7.03445969011705,-33.6509142422919,
-9.85745342186599));
#41635=CARTESIAN_POINT('Ctrl Pts',(-1.45949538523709,-33.8891664658769,
-12.0217671045718));
#41636=CARTESIAN_POINT('Ctrl Pts',(4.4713981581054,-34.127418689462,-11.2543151549789));
#41637=CARTESIAN_POINT('Ctrl Pts',(9.31184540238453,-34.3656709130471,-7.7422571837204));
#41638=CARTESIAN_POINT('Ctrl Pts',(11.8813995168772,-34.6039231366322,-2.34208381891072));
#41639=CARTESIAN_POINT('Ctrl Pts',(11.5534196448359,-34.8421753602173,3.62925689493129));
#41640=CARTESIAN_POINT('Ctrl Pts',(8.4078907084614,-35.0804275838025,8.71552551064461));
#41641=CARTESIAN_POINT('Ctrl Pts',(3.21191737478198,-35.3186798073875,11.6763263861354));
#41642=CARTESIAN_POINT('Ctrl Pts',(-2.76735087046105,-35.5569320309727,
11.7896047544065));
#41643=CARTESIAN_POINT('Ctrl Pts',(-8.0717412745462,-35.7951842545577,9.0277352560064));
#41644=CARTESIAN_POINT('Ctrl Pts',(-11.4076645353736,-36.0334364781429,
4.06425897911157));
#41645=CARTESIAN_POINT('Ctrl Pts',(-11.9615842218583,-36.2716887017279,
-1.89037398218391));
#41646=CARTESIAN_POINT('Ctrl Pts',(-9.59841519981894,-36.5099409253131,
-7.38399871717217));
#41647=CARTESIAN_POINT('Ctrl Pts',(-4.89446678402209,-36.7481931488981,
-11.0768770755603));
#41648=CARTESIAN_POINT('Ctrl Pts',(1.00310213358974,-36.9864453724833,-12.0684214728383));
#41649=CARTESIAN_POINT('Ctrl Pts',(6.65604339548311,-37.2246975960683,-10.1168226081503));
#41650=CARTESIAN_POINT('Ctrl Pts',(10.6857651719592,-37.4629498196534,-5.69801958831428));
#41651=CARTESIAN_POINT('Ctrl Pts',(12.1095352541438,-37.7012020432385,0.110367508901437));
#41652=CARTESIAN_POINT('Ctrl Pts',(10.5801330995995,-37.9394542668236,5.89183943199494));
#41653=CARTESIAN_POINT('Ctrl Pts',(6.47054360757812,-38.1777064904088,10.2364593795502));
#41654=CARTESIAN_POINT('Ctrl Pts',(0.782963431634552,-38.4159587139938,
12.0847005020222));
#41655=CARTESIAN_POINT('Ctrl Pts',(-5.09553927313002,-38.654210937579,10.9858258354038));
#41656=CARTESIAN_POINT('Ctrl Pts',(-9.73142540874922,-38.892463161164,7.20782703887185));
#41657=CARTESIAN_POINT('Ctrl Pts',(-11.9940147050091,-39.1307153847492,
1.67203502972045));
#41658=CARTESIAN_POINT('Ctrl Pts',(-11.3317672367851,-39.3689676083343,
-4.27149835313993));
#41659=CARTESIAN_POINT('Ctrl Pts',(-7.9057023418188,-39.6072198319193,-9.17337595717302));
#41660=CARTESIAN_POINT('Ctrl Pts',(-2.55231374440726,-39.8454720555045,
-11.8380461293086));
#41661=CARTESIAN_POINT('Ctrl Pts',(3.42485244245177,-40.0837242790895,-11.6159364534383));
#41662=CARTESIAN_POINT('Ctrl Pts',(6.85055888668833,-40.2425590948129,-9.57882655533487));
#41663=CARTESIAN_POINT('Ctrl Pts',(8.21649993060639,-40.3219765026746,-8.21216437170453));
#41664=CARTESIAN_POINT('Ctrl Pts',(9.19775812595307,-19.0332869065834,-7.9774004837349));
#41665=CARTESIAN_POINT('Ctrl Pts',(10.5249979873448,-19.1127248583274,-6.44713139899647));
#41666=CARTESIAN_POINT('Ctrl Pts',(12.3992382005735,-19.2715802179331,-2.71328281678768));
#41667=CARTESIAN_POINT('Ctrl Pts',(12.1849624523942,-19.5098529854005,3.5524320943754));
#41668=CARTESIAN_POINT('Ctrl Pts',(8.99943076537519,-19.7481052089856,8.94988154018779));
#41669=CARTESIAN_POINT('Ctrl Pts',(3.61905949217688,-19.9863574325707,12.1653851728116));
#41670=CARTESIAN_POINT('Ctrl Pts',(-2.64383037995317,-20.2246096561558,
12.4137641417282));
#41671=CARTESIAN_POINT('Ctrl Pts',(-8.26199868104885,-20.4628618797409,
9.63494724165815));
#41672=CARTESIAN_POINT('Ctrl Pts',(-11.8652849728387,-20.701114103326,4.50635888487473));
#41673=CARTESIAN_POINT('Ctrl Pts',(-12.5749753797014,-20.9393663269111,
-1.72116033428216));
#41674=CARTESIAN_POINT('Ctrl Pts',(-10.2179843589404,-21.1776185504962,
-7.52895831327075));
#41675=CARTESIAN_POINT('Ctrl Pts',(-5.36912083960681,-21.4158707740812,
-11.5006481349737));
#41676=CARTESIAN_POINT('Ctrl Pts',(0.789118917326245,-21.6541229976664,
-12.6676634715821));
#41677=CARTESIAN_POINT('Ctrl Pts',(6.7549146023214,-21.8923752212515,-10.7453949518229));
#41678=CARTESIAN_POINT('Ctrl Pts',(11.0733798014692,-22.1306274448366,-6.20263278174869));
#41679=CARTESIAN_POINT('Ctrl Pts',(12.6913638180259,-22.3688796684217,-0.147225002684643));
#41680=CARTESIAN_POINT('Ctrl Pts',(11.2142867514966,-22.6071318920068,5.94408643438964));
#41681=CARTESIAN_POINT('Ctrl Pts',(7.00236541639435,-22.8453841155919,10.585805121515));
#41682=CARTESIAN_POINT('Ctrl Pts',(1.08276717264934,-23.083636339177,12.6459482119938));
#41683=CARTESIAN_POINT('Ctrl Pts',(-5.10088706636648,-23.3218885627621,
11.6221057648454));
#41684=CARTESIAN_POINT('Ctrl Pts',(-10.0405806370614,-23.5601407863472,
7.76396365165987));
#41685=CARTESIAN_POINT('Ctrl Pts',(-12.5316633703614,-23.7983930099322,
2.01241256706129));
#41686=CARTESIAN_POINT('Ctrl Pts',(-11.966631334789,-24.0366452335174,-4.22990846913594));
#41687=CARTESIAN_POINT('Ctrl Pts',(-8.48327970686742,-24.2748974571024,
-9.44067564153303));
#41688=CARTESIAN_POINT('Ctrl Pts',(-2.93109845679036,-24.5131496806876,
-12.3491316697907));
#41689=CARTESIAN_POINT('Ctrl Pts',(3.33589398903813,-24.7514019042726,-12.2459871978553));
#41690=CARTESIAN_POINT('Ctrl Pts',(8.78935717047004,-24.9896541278578,-9.15639621732265));
#41691=CARTESIAN_POINT('Ctrl Pts',(12.0993471787362,-25.2279063514429,-3.83382172331087));
#41692=CARTESIAN_POINT('Ctrl Pts',(12.4586519904683,-25.466158575028,2.42371238770974));
#41693=CARTESIAN_POINT('Ctrl Pts',(9.77964742449122,-25.7044107986131,8.09017227323569));
#41694=CARTESIAN_POINT('Ctrl Pts',(4.71566617699691,-25.9426630221981,11.7836702119933));
#41695=CARTESIAN_POINT('Ctrl Pts',(-1.49833136268259,-26.1809152457833,
12.603467550066));
#41696=CARTESIAN_POINT('Ctrl Pts',(-7.34692867819358,-26.4191674693684,
10.3496391316539));
#41697=CARTESIAN_POINT('Ctrl Pts',(-11.4038199313364,-26.6574196929535,
5.57182933439236));
#41698=CARTESIAN_POINT('Ctrl Pts',(-12.6796452179915,-26.8956719165386,
-0.564790495495845));
#41699=CARTESIAN_POINT('Ctrl Pts',(-10.8632671907382,-27.1339241401237,
-6.56367405502175));
#41700=CARTESIAN_POINT('Ctrl Pts',(-6.39764857121597,-27.3721763637088,
-10.9618649835306));
#41701=CARTESIAN_POINT('Ctrl Pts',(-0.371826194173351,-27.6104285872939,
-12.6867701342486));
#41702=CARTESIAN_POINT('Ctrl Pts',(5.74467397156553,-27.848680810879,-11.3177344074843));
#41703=CARTESIAN_POINT('Ctrl Pts',(10.4602122344436,-28.0869330344641,-7.1886265147338));
#41704=CARTESIAN_POINT('Ctrl Pts',(12.6248034968774,-28.3251852580492,-1.30641793587195));
#41705=CARTESIAN_POINT('Ctrl Pts',(11.7105657747989,-28.5634374816343,4.89438866377053));
#41706=CARTESIAN_POINT('Ctrl Pts',(7.94045553625644,-28.8016897052194,9.90159366135931));
#41707=CARTESIAN_POINT('Ctrl Pts',(2.23389498691868,-29.0399419288045,12.4940827732714));
#41708=CARTESIAN_POINT('Ctrl Pts',(-4.01744874544316,-29.2781941523896,
12.0396219515263));
#41709=CARTESIAN_POINT('Ctrl Pts',(-9.28905147476106,-29.5164463759747,
8.64904121028314));
#41710=CARTESIAN_POINT('Ctrl Pts',(-12.2953198623448,-29.7546985995598,
3.14920635090273));
#41711=CARTESIAN_POINT('Ctrl Pts',(-12.3031109132,-29.9929508231448,-3.1186299901457));
#41712=CARTESIAN_POINT('Ctrl Pts',(-9.31052461255024,-30.23120304673,-8.62592155059579));
#41713=CARTESIAN_POINT('Ctrl Pts',(-4.04736728517316,-30.4694552703151,
-12.0295972175649));
#41714=CARTESIAN_POINT('Ctrl Pts',(2.20282732255767,-30.7077074939002,-12.4995977113237));
#41715=CARTESIAN_POINT('Ctrl Pts',(7.91581526325055,-30.9459597174853,-9.92130333555153));
#41716=CARTESIAN_POINT('Ctrl Pts',(11.6983619519613,-31.1842119410704,-4.92348644751282));
#41717=CARTESIAN_POINT('Ctrl Pts',(12.6280122880337,-31.4224641646555,1.27502816094633));
#41718=CARTESIAN_POINT('Ctrl Pts',(10.47805110708,-31.6607163882406,7.16259981817759));
#41719=CARTESIAN_POINT('Ctrl Pts',(5.77279253415804,-31.8989686118257,11.3034179572156));
#41720=CARTESIAN_POINT('Ctrl Pts',(-0.340285255921168,-32.1372208354108,
12.687655303583));
#41721=CARTESIAN_POINT('Ctrl Pts',(-6.37037719127529,-32.3754730589959,
10.9777359049497));
#41722=CARTESIAN_POINT('Ctrl Pts',(-10.846916079753,-32.613725282581,6.59066026409488));
#41723=CARTESIAN_POINT('Ctrl Pts',(-12.6782019449145,-32.8519775061661,
0.596310826607594));
#41724=CARTESIAN_POINT('Ctrl Pts',(-11.4176364692439,-33.0902297297512,
-5.54346178971962));
#41725=CARTESIAN_POINT('Ctrl Pts',(-7.3726355681259,-33.3284819533363,-10.3313424073348));
#41726=CARTESIAN_POINT('Ctrl Pts',(-1.52965942840387,-33.5667341769214,
-12.5997036945728));
#41727=CARTESIAN_POINT('Ctrl Pts',(4.68635695588895,-33.8049864005065,-11.7953571221779));
#41728=CARTESIAN_POINT('Ctrl Pts',(9.75950472997413,-34.0432386240916,-8.11445984550458));
#41729=CARTESIAN_POINT('Ctrl Pts',(12.4525880502679,-34.2814908476767,-2.45467757688521));
#41730=CARTESIAN_POINT('Ctrl Pts',(12.1088408149773,-34.5197430712618,3.80373044244303));
#41731=CARTESIAN_POINT('Ctrl Pts',(8.81209315581226,-34.7579952948469,9.13451724870398));
#41732=CARTESIAN_POINT('Ctrl Pts',(3.3663276672789,-34.996247518432,12.237656197023));
#41733=CARTESIAN_POINT('Ctrl Pts',(-2.90038899301814,-35.2344997420171,
12.3563803299066));
#41734=CARTESIAN_POINT('Ctrl Pts',(-8.45978361366358,-35.4727519656022,
9.46173622141395));
#41735=CARTESIAN_POINT('Ctrl Pts',(-11.9560786482159,-35.7110041891873,
4.25964489491223));
#41736=CARTESIAN_POINT('Ctrl Pts',(-12.5366275691515,-35.9492564127724,
-1.98125216037409));
#41737=CARTESIAN_POINT('Ctrl Pts',(-10.0598511352971,-36.1875086363575,
-7.7389783971189));
#41738=CARTESIAN_POINT('Ctrl Pts',(-5.12976425887965,-36.4257608599426,
-11.6093888526747));
#41739=CARTESIAN_POINT('Ctrl Pts',(1.05132544564253,-36.6640130835277,-12.648600933315));
#41740=CARTESIAN_POINT('Ctrl Pts',(6.97602722060827,-36.9022653071128,-10.6031805544441));
#41741=CARTESIAN_POINT('Ctrl Pts',(11.1994745652053,-37.1405175306979,-5.97194720494374));
#41742=CARTESIAN_POINT('Ctrl Pts',(12.6916912259241,-37.378769754283,0.115673336338168));
#41743=CARTESIAN_POINT('Ctrl Pts',(11.0887643176353,-37.6170219778681,6.17508477858514));
#41744=CARTESIAN_POINT('Ctrl Pts',(6.78160968259757,-37.8552742014532,10.7285687654699));
#41745=CARTESIAN_POINT('Ctrl Pts',(0.820603756208997,-38.0935264250383,
12.6656625634705));
#41746=CARTESIAN_POINT('Ctrl Pts',(-5.34050314292663,-38.3317786486234,
11.5139603988529));
#41747=CARTESIAN_POINT('Ctrl Pts',(-10.1992557008902,-38.5700308722085,
7.55433740992863));
#41748=CARTESIAN_POINT('Ctrl Pts',(-12.5706171211714,-38.8082830957936,
1.75241674191245));
#41749=CARTESIAN_POINT('Ctrl Pts',(-11.8765326492695,-39.0465353193787,
-4.47684713181242));
#41750=CARTESIAN_POINT('Ctrl Pts',(-8.28576249547599,-39.2847875429638,
-9.6143784797947));
#41751=CARTESIAN_POINT('Ctrl Pts',(-2.67501413356175,-39.5230397665489,
-12.4071504841623));
#41752=CARTESIAN_POINT('Ctrl Pts',(3.58949941361916,-39.761291990134,-12.1743630678598));
#41753=CARTESIAN_POINT('Ctrl Pts',(7.17989388445823,-39.9201268058574,-10.0393207828014));
#41754=CARTESIAN_POINT('Ctrl Pts',(8.61150142334309,-39.9995442137191,-8.60695743600425));
#41755=CARTESIAN_POINT('',(-9.92494571122256,-40.0002656632106,-3.43140318666995));
#41756=CARTESIAN_POINT('Ctrl Pts',(8.61094305413662,-40.,-8.60639936142963));
#41757=CARTESIAN_POINT('Ctrl Pts',(8.39826176691623,-40.,-8.79212327549395));
#41758=CARTESIAN_POINT('Ctrl Pts',(8.1793730811141,-40.,-8.96994937667235));
#41759=CARTESIAN_POINT('Ctrl Pts',(7.954781095098,-40.,-9.13970638711416));
#41760=CARTESIAN_POINT('Ctrl Pts',(7.72804274039455,-40.,-9.31108572227973));
#41761=CARTESIAN_POINT('Ctrl Pts',(7.495491008298,-40.,-9.47424130261635));
#41762=CARTESIAN_POINT('Ctrl Pts',(7.25761308334299,-40.,-9.62895430403488));
#41763=CARTESIAN_POINT('Ctrl Pts',(7.01927567527136,-40.,-9.78396614786213));
#41764=CARTESIAN_POINT('Ctrl Pts',(6.77559089325141,-40.,-9.93050302215559));
#41765=CARTESIAN_POINT('Ctrl Pts',(6.52702586402077,-40.,-10.0682981589458));
#41766=CARTESIAN_POINT('Ctrl Pts',(6.27982630171823,-40.,-10.2053363320443));
#41767=CARTESIAN_POINT('Ctrl Pts',(6.02779937839588,-40.,-10.333728742847));
#41768=CARTESIAN_POINT('Ctrl Pts',(5.77139073178792,-40.,-10.4531635937111));
#41769=CARTESIAN_POINT('Ctrl Pts',(5.51880872660686,-40.,-10.5708159994268));
#41770=CARTESIAN_POINT('Ctrl Pts',(5.26197426229078,-40.,-10.6797763198721));
#41771=CARTESIAN_POINT('Ctrl Pts',(5.00130823865076,-40.,-10.7796963458467));
#41772=CARTESIAN_POINT('Ctrl Pts',(4.90713970194856,-40.,-10.8157935805452));
#41773=CARTESIAN_POINT('Ctrl Pts',(4.81247110047981,-40.,-10.8507104815111));
#41774=CARTESIAN_POINT('Ctrl Pts',(4.71732232047202,-40.,-10.8844289444319));
#41775=CARTESIAN_POINT('Ctrl Pts',(4.68473084450778,-40.,-10.8959785877772));
#41776=CARTESIAN_POINT('Ctrl Pts',(4.65208303079231,-40.,-10.9073876128803));
#41777=CARTESIAN_POINT('Ctrl Pts',(4.61937968084376,-40.,-10.9186552672315));
#41778=CARTESIAN_POINT('Ctrl Pts',(4.59185356383537,-40.,-10.9281391510713));
#41779=CARTESIAN_POINT('Ctrl Pts',(4.56428866349076,-40.,-10.9375226531726));
#41780=CARTESIAN_POINT('Ctrl Pts',(4.53669821841154,-40.,-10.9468011456384));
#41781=CARTESIAN_POINT('Ctrl Pts',(4.27228656872564,-40.,-11.0357211138538));
#41782=CARTESIAN_POINT('Ctrl Pts',(4.00522676966733,-40.,-11.1151060432448));
#41783=CARTESIAN_POINT('Ctrl Pts',(3.73596790268631,-40.,-11.1847326159485));
#41784=CARTESIAN_POINT('Ctrl Pts',(3.59988597511649,-40.,-11.2199214969307));
#41785=CARTESIAN_POINT('Ctrl Pts',(3.46324208616997,-40.,-11.2526170856896));
#41786=CARTESIAN_POINT('Ctrl Pts',(3.3260929489447,-40.,-11.2827856394737));
#41787=CARTESIAN_POINT('Ctrl Pts',(3.05396201990356,-40.,-11.3426459983151));
#41788=CARTESIAN_POINT('Ctrl Pts',(2.77984200145971,-40.,-11.3925606000749));
#41789=CARTESIAN_POINT('Ctrl Pts',(2.50427786210809,-40.,-11.4325612835728));
#41790=CARTESIAN_POINT('Ctrl Pts',(2.22869992361977,-40.,-11.472563970143));
#41791=CARTESIAN_POINT('Ctrl Pts',(1.95167706452487,-40.,-11.5026516741963));
#41792=CARTESIAN_POINT('Ctrl Pts',(1.67375680517849,-40.,-11.5228042110682));
#41793=CARTESIAN_POINT('Ctrl Pts',(1.39864205208426,-40.,-11.5427533152421));
#41794=CARTESIAN_POINT('Ctrl Pts',(1.12264731884322,-40.,-11.5529666784976));
#41795=CARTESIAN_POINT('Ctrl Pts',(0.846315501342459,-40.,-11.5533754838016));
#41796=CARTESIAN_POINT('Ctrl Pts',(0.643529262156045,-40.,-11.5536754857736));
#41797=CARTESIAN_POINT('Ctrl Pts',(0.440561694344327,-40.,-11.5486943578675));
#41798=CARTESIAN_POINT('Ctrl Pts',(0.237634295057578,-40.,-11.5383883933861));
#41799=CARTESIAN_POINT('Ctrl Pts',(0.200021572236072,-40.,-11.5364781762995));
#41800=CARTESIAN_POINT('Ctrl Pts',(0.162410249405166,-40.,-11.5343849868962));
#41801=CARTESIAN_POINT('Ctrl Pts',(0.124801765584846,-40.,-11.5321084946763));
#41802=CARTESIAN_POINT('Ctrl Pts',(0.0953789719671696,-40.,-11.5303274933182));
#41803=CARTESIAN_POINT('Ctrl Pts',(0.0659671184443719,-40.,-11.5284348486951));
#41804=CARTESIAN_POINT('Ctrl Pts',(0.0365696537066474,-40.,-11.5264308156415));
#41805=CARTESIAN_POINT('Ctrl Pts',(-0.236604483961962,-40.,-11.5078084614291));
#41806=CARTESIAN_POINT('Ctrl Pts',(-0.508615486317793,-40.,-11.4795673079924));
#41807=CARTESIAN_POINT('Ctrl Pts',(-0.778950107545266,-40.,-11.4417467199426));
#41808=CARTESIAN_POINT('Ctrl Pts',(-1.05191932377333,-40.,-11.4035575445037));
#41809=CARTESIAN_POINT('Ctrl Pts',(-1.32317999343783,-40.,-11.355601299064));
#41810=CARTESIAN_POINT('Ctrl Pts',(-1.59219408909529,-40.,-11.2978654190554));
#41811=CARTESIAN_POINT('Ctrl Pts',(-1.86120818475246,-40.,-11.2401295390468));
#41812=CARTESIAN_POINT('Ctrl Pts',(-2.12797635797297,-40.,-11.1726139378876));
#41813=CARTESIAN_POINT('Ctrl Pts',(-2.39194108188819,-40.,-11.0952540671311));
#41814=CARTESIAN_POINT('Ctrl Pts',(-2.65358663251976,-40.,-11.0185738741089));
#41815=CARTESIAN_POINT('Ctrl Pts',(-2.91247824429427,-40.,-10.9322209570422));
#41816=CARTESIAN_POINT('Ctrl Pts',(-3.16812267150543,-40.,-10.8364284814823));
#41817=CARTESIAN_POINT('Ctrl Pts',(-3.42177931996214,-40.,-10.741380846128));
#41818=CARTESIAN_POINT('Ctrl Pts',(-3.6722395742201,-40.,-10.6370394679647));
#41819=CARTESIAN_POINT('Ctrl Pts',(-3.9189871528201,-40.,-10.5235942855308));
#41820=CARTESIAN_POINT('Ctrl Pts',(-3.96835687549402,-40.,-10.5008959586527));
#41821=CARTESIAN_POINT('Ctrl Pts',(-4.01757784481209,-40.,-10.4778330705644));
#41822=CARTESIAN_POINT('Ctrl Pts',(-4.06664573143816,-40.,-10.4544069809796));
#41823=CARTESIAN_POINT('Ctrl Pts',(-4.10490890648528,-40.,-10.43613929863));
#41824=CARTESIAN_POINT('Ctrl Pts',(-4.14308479220665,-40.,-10.4176478398036));
#41825=CARTESIAN_POINT('Ctrl Pts',(-4.18113965154256,-40.,-10.3989489818942));
#41826=CARTESIAN_POINT('Ctrl Pts',(-4.42108222934686,-40.,-10.28104939569));
#41827=CARTESIAN_POINT('Ctrl Pts',(-4.65640472965588,-40.,-10.154821243158));
#41828=CARTESIAN_POINT('Ctrl Pts',(-4.88668744403159,-40.,-10.0205608401689));
#41829=CARTESIAN_POINT('Ctrl Pts',(-5.1173904554137,-40.,-9.88605539383993));
#41830=CARTESIAN_POINT('Ctrl Pts',(-5.34303579577258,-40.,-9.74348797326746));
#41831=CARTESIAN_POINT('Ctrl Pts',(-5.56317346343205,-40.,-9.59311272976814));
#41832=CARTESIAN_POINT('Ctrl Pts',(-5.78203974319709,-40.,-9.44360596673486));
#41833=CARTESIAN_POINT('Ctrl Pts',(-5.99546225547574,-40.,-9.28638090105349));
#41834=CARTESIAN_POINT('Ctrl Pts',(-6.20296370257059,-40.,-9.12164999225825));
#41835=CARTESIAN_POINT('Ctrl Pts',(-6.40709362328022,-40.,-8.95959566530491));
#41836=CARTESIAN_POINT('Ctrl Pts',(-6.6054936891356,-40.,-8.79027700677452));
#41837=CARTESIAN_POINT('Ctrl Pts',(-6.79766944718012,-40.,-8.61386626213952));
#41838=CARTESIAN_POINT('Ctrl Pts',(-6.91421310879249,-40.,-8.50688318406177));
#41839=CARTESIAN_POINT('Ctrl Pts',(-7.02846683632195,-40.,-8.39729127199965));
#41840=CARTESIAN_POINT('Ctrl Pts',(-7.14031214075949,-40.,-8.28512438529733));
#41841=CARTESIAN_POINT('Ctrl Pts',(-7.2322458360855,-40.,-8.19292635839208));
#41842=CARTESIAN_POINT('Ctrl Pts',(-7.32255217347812,-40.,-8.09898847748873));
#41843=CARTESIAN_POINT('Ctrl Pts',(-7.41118873118237,-40.,-8.00335941612173));
#41844=CARTESIAN_POINT('Ctrl Pts',(-7.44595173807725,-40.,-7.9658539690945));
#41845=CARTESIAN_POINT('Ctrl Pts',(-7.4804578335956,-40.,-7.9280884190582));
#41846=CARTESIAN_POINT('Ctrl Pts',(-7.5147044485466,-40.,-7.89006554572198));
#41847=CARTESIAN_POINT('Ctrl Pts',(-7.54132180807535,-40.,-7.86051317999608));
#41848=CARTESIAN_POINT('Ctrl Pts',(-7.56778133285553,-40.,-7.83080646097683));
#41849=CARTESIAN_POINT('Ctrl Pts',(-7.59406823886229,-40.,-7.8009624892378));
#41850=CARTESIAN_POINT('Ctrl Pts',(-7.76810920704413,-40.,-7.60337081623842));
#41851=CARTESIAN_POINT('Ctrl Pts',(-7.93474820210051,-40.,-7.39958701787578));
#41852=CARTESIAN_POINT('Ctrl Pts',(-8.09372374882493,-40.,-7.1900765576583));
#41853=CARTESIAN_POINT('Ctrl Pts',(-8.25269854013783,-40.,-6.98056709298144));
#41854=CARTESIAN_POINT('Ctrl Pts',(-8.40401024363677,-40.,-6.76533041686787));
#41855=CARTESIAN_POINT('Ctrl Pts',(-8.54735114599831,-40.,-6.54480817806209));
#41856=CARTESIAN_POINT('Ctrl Pts',(-8.68948030195279,-40.,-6.32615014567713));
#41857=CARTESIAN_POINT('Ctrl Pts',(-8.82377306273544,-40.,-6.10229494090462));
#41858=CARTESIAN_POINT('Ctrl Pts',(-8.94988037165709,-40.,-5.87365868174475));
#41859=CARTESIAN_POINT('Ctrl Pts',(-8.96660934330763,-40.,-5.84332856424022));
#41860=CARTESIAN_POINT('Ctrl Pts',(-8.98319419515905,-40.,-5.81291429736071));
#41861=CARTESIAN_POINT('Ctrl Pts',(-8.9996340436321,-40.,-5.78241684186142));
#41862=CARTESIAN_POINT('Ctrl Pts',(-9.02204331979085,-40.,-5.74084554006121));
#41863=CARTESIAN_POINT('Ctrl Pts',(-9.04417775624957,-40.,-5.69912961896715));
#41864=CARTESIAN_POINT('Ctrl Pts',(-9.06603067192976,-40.,-5.65728119034538));
#41865=CARTESIAN_POINT('Ctrl Pts',(-9.18590518599412,-40.,-5.42772097427143));
#41866=CARTESIAN_POINT('Ctrl Pts',(-9.29736055437846,-40.,-5.19408576675231));
#41867=CARTESIAN_POINT('Ctrl Pts',(-9.40010767564824,-40.,-4.95680440176927));
#41868=CARTESIAN_POINT('Ctrl Pts',(-9.50150771608712,-40.,-4.72263394806383));
#41869=CARTESIAN_POINT('Ctrl Pts',(-9.59442649981932,-40.,-4.4849117408585));
#41870=CARTESIAN_POINT('Ctrl Pts',(-9.67853712371623,-40.,-4.2440387488937));
#41871=CARTESIAN_POINT('Ctrl Pts',(-9.73985884412757,-40.,-4.0684278024571));
#41872=CARTESIAN_POINT('Ctrl Pts',(-9.79649777621682,-40.,-3.89114186247201));
#41873=CARTESIAN_POINT('Ctrl Pts',(-9.84830976294177,-40.,-3.71233506504282));
#41874=CARTESIAN_POINT('Ctrl Pts',(-9.87531187063298,-40.,-3.6191488989586));
#41875=CARTESIAN_POINT('Ctrl Pts',(-9.90100270302723,-40.,-3.52554965431835));
#41876=CARTESIAN_POINT('Ctrl Pts',(-9.92537747903998,-40.,-3.43156570488038));
#41877=CARTESIAN_POINT('Ctrl Pts',(7.93381306740072,-20.,-6.87936125025729));
#41878=CARTESIAN_POINT('Ctrl Pts',(8.1133453307756,-20.,-6.70251189458692));
#41879=CARTESIAN_POINT('Ctrl Pts',(8.28605380477966,-20.,-6.51937440106505));
#41880=CARTESIAN_POINT('Ctrl Pts',(8.45179833248014,-20.,-6.3304725879375));
#41881=CARTESIAN_POINT('Ctrl Pts',(8.62014953535816,-20.,-6.13859990346896));
#41882=CARTESIAN_POINT('Ctrl Pts',(8.78131641900121,-20.,-5.94077982286031));
#41883=CARTESIAN_POINT('Ctrl Pts',(8.93512781381366,-20.,-5.73751337586325));
#41884=CARTESIAN_POINT('Ctrl Pts',(9.09135990232769,-20.,-5.53104790834766));
#41885=CARTESIAN_POINT('Ctrl Pts',(9.24000360283395,-20.,-5.3189629086236));
#41886=CARTESIAN_POINT('Ctrl Pts',(9.38084825643788,-20.,-5.10173994480306));
#41887=CARTESIAN_POINT('Ctrl Pts',(9.52214874442358,-20.,-4.88381395326448));
#41888=CARTESIAN_POINT('Ctrl Pts',(9.65560002828852,-20.,-4.66071618819661));
#41889=CARTESIAN_POINT('Ctrl Pts',(9.78095181260842,-20.,-4.43289630258322));
#41890=CARTESIAN_POINT('Ctrl Pts',(9.90574238975571,-20.,-4.20609637974551));
#41891=CARTESIAN_POINT('Ctrl Pts',(10.0225061921301,-20.,-3.97461598479587));
#41892=CARTESIAN_POINT('Ctrl Pts',(10.1309533968524,-20.,-3.73887037049945));
#41893=CARTESIAN_POINT('Ctrl Pts',(10.1620449654918,-20.,-3.67128263536989));
#41894=CARTESIAN_POINT('Ctrl Pts',(10.1924526568096,-20.,-3.6033441669511));
#41895=CARTESIAN_POINT('Ctrl Pts',(10.22216892119,-20.,-3.53506441406799));
#41896=CARTESIAN_POINT('Ctrl Pts',(10.2396840907369,-20.,-3.49481940099851));
#41897=CARTESIAN_POINT('Ctrl Pts',(10.2569611674535,-20.,-3.45445054560652));
#41898=CARTESIAN_POINT('Ctrl Pts',(10.2739835311438,-20.,-3.41399615802376));
#41899=CARTESIAN_POINT('Ctrl Pts',(10.376972988476,-20.,-3.16923723384292));
#41900=CARTESIAN_POINT('Ctrl Pts',(10.4707505425312,-20.,-2.92110624349569));
#41901=CARTESIAN_POINT('Ctrl Pts',(10.5551246852504,-20.,-2.67011766566478));
#41902=CARTESIAN_POINT('Ctrl Pts',(10.5927935636518,-20.,-2.55806368901074));
#41903=CARTESIAN_POINT('Ctrl Pts',(10.6285877022248,-20.,-2.44543962431441));
#41904=CARTESIAN_POINT('Ctrl Pts',(10.6624876486376,-20.,-2.33228893760792));
#41905=CARTESIAN_POINT('Ctrl Pts',(10.7376977925035,-20.,-2.0812537494667));
#41906=CARTESIAN_POINT('Ctrl Pts',(10.8035876329606,-20.,-1.82762824132255));
#41907=CARTESIAN_POINT('Ctrl Pts',(10.8602429504416,-20.,-1.57194508022938));
#41908=CARTESIAN_POINT('Ctrl Pts',(10.9173812906925,-20.,-1.31408205687149));
#41909=CARTESIAN_POINT('Ctrl Pts',(10.9651271234088,-20.,-1.05412557296116));
#41910=CARTESIAN_POINT('Ctrl Pts',(11.0035202229091,-20.,-0.792598803100003));
#41911=CARTESIAN_POINT('Ctrl Pts',(11.0420807378013,-20.,-0.529931630217876));
#41912=CARTESIAN_POINT('Ctrl Pts',(11.0712069012446,-20.,-0.265679827372533));
#41913=CARTESIAN_POINT('Ctrl Pts',(11.0908885652656,-20.,-0.000359128301619826));
#41914=CARTESIAN_POINT('Ctrl Pts',(11.1054206053359,-20.,0.195541534685157));
#41915=CARTESIAN_POINT('Ctrl Pts',(11.1148027799583,-19.9999999999999,0.392025269798154));
#41916=CARTESIAN_POINT('Ctrl Pts',(11.1190128627105,-20.,0.588886412300435));
#41917=CARTESIAN_POINT('Ctrl Pts',(11.1196345841872,-20.,0.617957764914658));
#41918=CARTESIAN_POINT('Ctrl Pts',(11.1201435132142,-20.,0.647039404376552));
#41919=CARTESIAN_POINT('Ctrl Pts',(11.1205394628636,-20.,0.676124093961359));
#41920=CARTESIAN_POINT('Ctrl Pts',(11.1242136969702,-20.,0.946016891253661));
#41921=CARTESIAN_POINT('Ctrl Pts',(11.1181568313559,-20.,1.21559421576539));
#41922=CARTESIAN_POINT('Ctrl Pts',(11.1024699155507,-20.,1.48430357102738));
#41923=CARTESIAN_POINT('Ctrl Pts',(11.0859047811347,-20.,1.76805639051336));
#41924=CARTESIAN_POINT('Ctrl Pts',(11.0586017438615,-20.,2.05084190407209));
#41925=CARTESIAN_POINT('Ctrl Pts',(11.0206211947832,-20.,2.33203086493937));
#41926=CARTESIAN_POINT('Ctrl Pts',(10.9826406457049,-20.,2.61321982580659));
#41927=CARTESIAN_POINT('Ctrl Pts',(10.9339826723985,-20.,2.89281305830032));
#41928=CARTESIAN_POINT('Ctrl Pts',(10.87464624646,-20.,3.17019109503699));
#41929=CARTESIAN_POINT('Ctrl Pts',(10.8153870220998,-20.,3.4472082400973));
#41930=CARTESIAN_POINT('Ctrl Pts',(10.7454772306754,-20.,3.72201679033749));
#41931=CARTESIAN_POINT('Ctrl Pts',(10.6652311260161,-20.,3.99411127683229));
#41932=CARTESIAN_POINT('Ctrl Pts',(10.5849850213568,-20.,4.26620576332708));
#41933=CARTESIAN_POINT('Ctrl Pts',(10.4944023351477,-20.,4.53558691968041));
#41934=CARTESIAN_POINT('Ctrl Pts',(10.3937362784269,-20.,4.80173496530221));
#41935=CARTESIAN_POINT('Ctrl Pts',(10.3777423329852,-20.,4.84402089026791));
#41936=CARTESIAN_POINT('Ctrl Pts',(10.3614937302683,-20.,4.88622515835007));
#41937=CARTESIAN_POINT('Ctrl Pts',(10.3449913509334,-20.,4.92834563232135));
#41938=CARTESIAN_POINT('Ctrl Pts',(10.3343844651706,-20.,4.95541851960774));
#41939=CARTESIAN_POINT('Ctrl Pts',(10.3236726703155,-20.,4.98245685781199));
#41940=CARTESIAN_POINT('Ctrl Pts',(10.3128617315938,-20.,5.00944653944195));
#41941=CARTESIAN_POINT('Ctrl Pts',(10.2113685957593,-20.,5.2628257782202));
#41942=CARTESIAN_POINT('Ctrl Pts',(10.101026009192,-20.,5.51221436662211));
#41943=CARTESIAN_POINT('Ctrl Pts',(9.98219337299323,-20.,5.75718786449156));
#41944=CARTESIAN_POINT('Ctrl Pts',(9.86134406372978,-20.,6.00631873419524));
#41945=CARTESIAN_POINT('Ctrl Pts',(9.73171400203854,-20.,6.25088396547886));
#41946=CARTESIAN_POINT('Ctrl Pts',(9.59362742899954,-20.,6.4904337301993));
#41947=CARTESIAN_POINT('Ctrl Pts',(9.45505341277439,-20.,6.73082910139681));
#41948=CARTESIAN_POINT('Ctrl Pts',(9.30796286010393,-20.,6.96617413669482));
#41949=CARTESIAN_POINT('Ctrl Pts',(9.15263229119251,-20.,7.19600189657105));
#41950=CARTESIAN_POINT('Ctrl Pts',(8.99804398991272,-20.,7.42473139415287));
#41951=CARTESIAN_POINT('Ctrl Pts',(8.83529395844639,-20.,7.64799680129097));
#41952=CARTESIAN_POINT('Ctrl Pts',(8.66460799084262,-20.,7.86531682618203));
#41953=CARTESIAN_POINT('Ctrl Pts',(8.55444285880692,-20.,8.00558078327371));
#41954=CARTESIAN_POINT('Ctrl Pts',(8.44097088267069,-20.,8.14336759878132));
#41955=CARTESIAN_POINT('Ctrl Pts',(8.32424315342715,-20.,8.27854145188553));
#41956=CARTESIAN_POINT('Ctrl Pts',(8.23663382474174,-20.,8.37999541319385));
#41957=CARTESIAN_POINT('Ctrl Pts',(8.14719031008403,-20.,8.47997733921384));
#41958=CARTESIAN_POINT('Ctrl Pts',(8.05595931410645,-20.,8.57845490970599));
#41959=CARTESIAN_POINT('Ctrl Pts',(8.01761638599056,-20.,8.61984345716124));
#41960=CARTESIAN_POINT('Ctrl Pts',(7.97895769445338,-20.,8.66096625341727));
#41961=CARTESIAN_POINT('Ctrl Pts',(7.93998660073734,-20.,8.70182079217647));
#41962=CARTESIAN_POINT('Ctrl Pts',(7.91066081922242,-20.,8.7325638677051));
#41963=CARTESIAN_POINT('Ctrl Pts',(7.88115851940967,-20.,8.76315450959376));
#41964=CARTESIAN_POINT('Ctrl Pts',(7.85149823338772,-20.,8.79357447449731));
#41965=CARTESIAN_POINT('Ctrl Pts',(7.65681753599435,-20.,8.9932414627969));
#41966=CARTESIAN_POINT('Ctrl Pts',(7.45515096990198,-20.,9.18575086334707));
#41967=CARTESIAN_POINT('Ctrl Pts',(7.2470114550717,-20.,9.37088205609219));
#41968=CARTESIAN_POINT('Ctrl Pts',(7.03612872385928,-20.,9.55845322243481));
#41969=CARTESIAN_POINT('Ctrl Pts',(6.81860091988332,-20.,9.73845086287543));
#41970=CARTESIAN_POINT('Ctrl Pts',(6.59491638211396,-20.,9.91061618523869));
#41971=CARTESIAN_POINT('Ctrl Pts',(6.37323524853758,-20.,10.0812395291883));
#41972=CARTESIAN_POINT('Ctrl Pts',(6.14550664670372,-20.,10.2441705630064));
#41973=CARTESIAN_POINT('Ctrl Pts',(5.91216887742395,-20.,10.399123041683));
#41974=CARTESIAN_POINT('Ctrl Pts',(5.86175766100922,-20.,10.4325995892675));
#41975=CARTESIAN_POINT('Ctrl Pts',(5.81108451494134,-20.,10.4657035986193));
#41976=CARTESIAN_POINT('Ctrl Pts',(5.76015366565449,-20.,10.4984319462714));
#41977=CARTESIAN_POINT('Ctrl Pts',(5.72101534189377,-20.,10.5235823744401));
#41978=CARTESIAN_POINT('Ctrl Pts',(5.68172721143778,-20.,10.5485093492459));
#41979=CARTESIAN_POINT('Ctrl Pts',(5.64230701875108,-20.,10.5732018578478));
#41980=CARTESIAN_POINT('Ctrl Pts',(5.39975652925315,-20.,10.7251336379868));
#41981=CARTESIAN_POINT('Ctrl Pts',(5.1520474980573,-20.,10.8682962687084));
#41982=CARTESIAN_POINT('Ctrl Pts',(4.8996827113077,-20.,11.0024328307128));
#41983=CARTESIAN_POINT('Ctrl Pts',(4.64696653000309,-20.,11.1367561654366));
#41984=CARTESIAN_POINT('Ctrl Pts',(4.38958112280953,-20.,11.2620286879808));
#41985=CARTESIAN_POINT('Ctrl Pts',(4.12799552796009,-20.,11.3779546570887));
#41986=CARTESIAN_POINT('Ctrl Pts',(3.90990991961388,-20.,11.4746028899953));
#41987=CARTESIAN_POINT('Ctrl Pts',(3.68890412368266,-20.,11.564754097854));
#41988=CARTESIAN_POINT('Ctrl Pts',(3.46523470555786,-20.,11.6482137561969));
#41989=CARTESIAN_POINT('Ctrl Pts',(3.36017632166552,-20.,11.6874150779477));
#41990=CARTESIAN_POINT('Ctrl Pts',(3.25453010754724,-20.,11.7251397777184));
#41991=CARTESIAN_POINT('Ctrl Pts',(3.14832787575818,-20.,11.7613864006883));
#41992=CARTESIAN_POINT('Ctrl Pts',(-9.92458237182475,-40.0002656632106,
-3.43127756744706));
#41993=CARTESIAN_POINT('Ctrl Pts',(-9.92574258937462,-40.0001771088071,
-3.42792176937577));
#41994=CARTESIAN_POINT('Ctrl Pts',(-9.92690110488082,-40.0000885544035,
-3.42456538284806));
#41995=CARTESIAN_POINT('Ctrl Pts',(-9.92805791774733,-40.,-3.42120840959077));
#41996=CARTESIAN_POINT('Ctrl Pts',(-3.14809266229074,-20.0004548598273,
11.7612561652465));
#41997=CARTESIAN_POINT('Ctrl Pts',(-5.10435921967941,-20.079872267689,11.2376294107338));
#41998=CARTESIAN_POINT('Ctrl Pts',(-8.74855648214142,-20.2387070834124,
9.19577637638592));
#41999=CARTESIAN_POINT('Ctrl Pts',(-12.0824131583272,-20.4769593069975,
3.88694525557923));
#42000=CARTESIAN_POINT('Ctrl Pts',(-12.4691756011198,-20.7152115305826,
-2.36849165908917));
#42001=CARTESIAN_POINT('Ctrl Pts',(-9.81532842158459,-20.9534637541677,
-8.04695416362741));
#42002=CARTESIAN_POINT('Ctrl Pts',(-4.76767052948596,-21.1917159777528,
-11.7626807483447));
#42003=CARTESIAN_POINT('Ctrl Pts',(1.44262007163241,-21.4299682013379,-12.6099815538241));
#42004=CARTESIAN_POINT('Ctrl Pts',(7.30112969128478,-21.668220424923,-10.3819902917566));
#42005=CARTESIAN_POINT('Ctrl Pts',(11.3790859526647,-21.9064726485081,-5.62216684002108));
#42006=CARTESIAN_POINT('Ctrl Pts',(12.6820163068472,-22.1447248720932,0.508761805007712));
#42007=CARTESIAN_POINT('Ctrl Pts',(10.8921610480429,-22.3829770956783,6.51560837433268));
#42008=CARTESIAN_POINT('Ctrl Pts',(6.44602083161166,-22.6212293192634,10.9334889418598));
#42009=CARTESIAN_POINT('Ctrl Pts',(0.427879238319787,-22.8594815428485,
12.6850014557692));
#42010=CARTESIAN_POINT('Ctrl Pts',(-5.69460937880688,-23.0977337664336,
11.343005608659));
#42011=CARTESIAN_POINT('Ctrl Pts',(-10.4283456669994,-23.3359859900187,
7.2347740805613));
#42012=CARTESIAN_POINT('Ctrl Pts',(-12.6189061760199,-23.5742382136038,
1.36218808736743));
#42013=CARTESIAN_POINT('Ctrl Pts',(-11.7320759505821,-23.8124904371889,
-4.8425968202088));
#42014=CARTESIAN_POINT('Ctrl Pts',(-7.9841274603316,-24.050742660774,-9.86641060411259));
#42015=CARTESIAN_POINT('Ctrl Pts',(-2.28907833971999,-24.2889948843591,
-12.4840886814594));
#42016=CARTESIAN_POINT('Ctrl Pts',(3.96421161517395,-24.5272471079442,-12.0572540805866));
#42017=CARTESIAN_POINT('Ctrl Pts',(9.25074357873224,-24.7654993315293,-8.68999959656226));
#42018=CARTESIAN_POINT('Ctrl Pts',(12.2812834041494,-25.0037515551144,-3.20350240934556));
#42019=CARTESIAN_POINT('Ctrl Pts',(12.3167689831387,-25.2420037786995,3.06423751515814));
#42020=CARTESIAN_POINT('Ctrl Pts',(9.34854639793627,-25.4802560022846,8.58469743127443));
#42021=CARTESIAN_POINT('Ctrl Pts',(4.10048035829083,-25.7185082258697,12.0115948386183));
#42022=CARTESIAN_POINT('Ctrl Pts',(-2.14757572311472,-25.9567604494548,
12.5092073390711));
#42023=CARTESIAN_POINT('Ctrl Pts',(-7.87189942455396,-26.1950126730399,
9.95618145611698));
#42024=CARTESIAN_POINT('Ctrl Pts',(-11.6764916927204,-26.433264896625,4.97512728354432));
#42025=CARTESIAN_POINT('Ctrl Pts',(-12.6335211398357,-26.6715171202101,
-1.21921833443057));
#42026=CARTESIAN_POINT('Ctrl Pts',(-10.5095956183063,-26.9097693437952,
-7.11623142381309));
#42027=CARTESIAN_POINT('Ctrl Pts',(-5.82267989949552,-27.1480215673803,
-11.2777989220269));
#42028=CARTESIAN_POINT('Ctrl Pts',(0.284221140002502,-27.3862737909654,
-12.6890333785201));
#42029=CARTESIAN_POINT('Ctrl Pts',(6.32180876134884,-27.6245260145505,-11.0057750168977));
#42030=CARTESIAN_POINT('Ctrl Pts',(10.8176877886728,-27.8627782381356,-6.63852247449934));
#42031=CARTESIAN_POINT('Ctrl Pts',(12.6754417380569,-28.1010304617207,-0.652323909386644));
#42032=CARTESIAN_POINT('Ctrl Pts',(11.4420174822295,-28.3392826853058,5.49295782561537));
#42033=CARTESIAN_POINT('Ctrl Pts',(7.41821196824627,-28.5775349088909,10.2986640362622));
#42034=CARTESIAN_POINT('Ctrl Pts',(1.58531643343681,-28.815787132476,12.592820237878));
#42035=CARTESIAN_POINT('Ctrl Pts',(-4.63419249983834,-29.0540393560611,
11.8159472583486));
#42036=CARTESIAN_POINT('Ctrl Pts',(-9.72355424374604,-29.2922915796462,
8.15750222841293));
#42037=CARTESIAN_POINT('Ctrl Pts',(-12.4416188307888,-29.5305438032313,
2.50967539873089));
#42038=CARTESIAN_POINT('Ctrl Pts',(-12.125527941276,-29.7687960268164,-3.75018957960365));
#42039=CARTESIAN_POINT('Ctrl Pts',(-8.85236711500349,-30.0070482504015,
-9.0954904320129));
#42040=CARTESIAN_POINT('Ctrl Pts',(-3.42036678980662,-30.2453004739866,
-12.2226609525431));
#42041=CARTESIAN_POINT('Ctrl Pts',(2.8457633032496,-30.4835526975717,-12.3690735691688));
#42042=CARTESIAN_POINT('Ctrl Pts',(8.41789300705035,-30.7218049211568,-9.4990224265177));
#42043=CARTESIAN_POINT('Ctrl Pts',(11.9371390374505,-30.9600571447419,-4.3124310241683));
#42044=CARTESIAN_POINT('Ctrl Pts',(12.5452578039889,-31.198309368327,1.92583913375176));
#42045=CARTESIAN_POINT('Ctrl Pts',(10.0939465085343,-31.4365615919121,7.69445213257468));
#42046=CARTESIAN_POINT('Ctrl Pts',(5.18100996193967,-31.6748138154972,11.5866080244356));
#42047=CARTESIAN_POINT('Ctrl Pts',(-0.995426934883139,-31.9130660390823,
12.6531211546773));
#42048=CARTESIAN_POINT('Ctrl Pts',(-6.92910763357261,-32.1513182626674,
10.6338994324754));
#42049=CARTESIAN_POINT('Ctrl Pts',(-11.1729768889136,-32.3895704862526,
6.02137336306566));
#42050=CARTESIAN_POINT('Ctrl Pts',(-12.692076202498,-32.6278227098376,-0.0595936877313756));
#42051=CARTESIAN_POINT('Ctrl Pts',(-11.1159406401054,-32.8660749334227,
-6.12602754019978));
#42052=CARTESIAN_POINT('Ctrl Pts',(-6.82894464797713,-33.1043271570078,
-10.6984982465997));
#42053=CARTESIAN_POINT('Ctrl Pts',(-0.876564103841478,-33.3425793805929,
-12.6619108000923));
#42054=CARTESIAN_POINT('Ctrl Pts',(5.28958538888388,-33.580831604178,-11.5374449576727));
#42055=CARTESIAN_POINT('Ctrl Pts',(10.1657560858716,-33.8190838277631,-7.59932582142831));
#42056=CARTESIAN_POINT('Ctrl Pts',(12.5627892268212,-34.0573360513483,-1.80794816851931));
#42057=CARTESIAN_POINT('Ctrl Pts',(11.8961168924868,-34.2955882749333,4.42433640425057));
#42058=CARTESIAN_POINT('Ctrl Pts',(8.32832142376291,-34.5338404985185,9.5776516954902));
#42059=CARTESIAN_POINT('Ctrl Pts',(2.72948623249549,-34.7720927221035,12.395251294106));
#42060=CARTESIAN_POINT('Ctrl Pts',(-3.53499269162053,-35.0103449456886,
12.1900031340674));
#42061=CARTESIAN_POINT('Ctrl Pts',(-8.93738786424591,-35.2485971692737,
9.01196137918275));
#42062=CARTESIAN_POINT('Ctrl Pts',(-12.1602094057867,-35.4868493928589,
3.63615964285339));
#42063=CARTESIAN_POINT('Ctrl Pts',(-12.4175031914886,-35.7251016164439,
-2.62639757513609));
#42064=CARTESIAN_POINT('Ctrl Pts',(-9.6465226171822,-35.9633538400291,-8.24845143865875));
#42065=CARTESIAN_POINT('Ctrl Pts',(-4.52303069773246,-36.2016060636141,
-11.858943589337));
#42066=CARTESIAN_POINT('Ctrl Pts',(1.70349921887366,-36.4398582871992,-12.5773781093279));
#42067=CARTESIAN_POINT('Ctrl Pts',(7.51459433853917,-36.6781105107843,-10.2285493487157));
#42068=CARTESIAN_POINT('Ctrl Pts',(11.4930945153334,-36.9163627343694,-5.38526953581525));
#42069=CARTESIAN_POINT('Ctrl Pts',(12.6687572341596,-37.1546149579545,0.771323677356681));
#42070=CARTESIAN_POINT('Ctrl Pts',(10.7548718477098,-37.3928671815396,6.7398131282622));
#42071=CARTESIAN_POINT('Ctrl Pts',(6.2181805169326,-37.6311194051247,11.0646545543017));
#42072=CARTESIAN_POINT('Ctrl Pts',(0.165052320677689,-37.8693716287098,
12.6911429724317));
#42073=CARTESIAN_POINT('Ctrl Pts',(-5.92832693959693,-38.107623852295,11.2226236804367));
#42074=CARTESIAN_POINT('Ctrl Pts',(-10.5759575529497,-38.34587607588,7.01722786017004));
#42075=CARTESIAN_POINT('Ctrl Pts',(-12.644412242237,-38.5841282994652,1.10052888764604));
#42076=CARTESIAN_POINT('Ctrl Pts',(-11.6292598420606,-38.8223805230502,
-5.08455422895767));
#42077=CARTESIAN_POINT('Ctrl Pts',(-7.77805527350331,-39.0606327466353,
-10.0296666573467));
#42078=CARTESIAN_POINT('Ctrl Pts',(-2.03002093474416,-39.2988849702204,
-12.528816073021));
#42079=CARTESIAN_POINT('Ctrl Pts',(4.21310916249937,-39.5371371938055,-11.972572766274));
#42080=CARTESIAN_POINT('Ctrl Pts',(9.42871875276412,-39.7753894173906,-8.49650536082229));
#42081=CARTESIAN_POINT('Ctrl Pts',(12.3450606821512,-40.0136416409757,-2.94849454622041));
#42082=CARTESIAN_POINT('Ctrl Pts',(12.2505387102373,-40.2518938645608,3.31879409118882));
#42083=CARTESIAN_POINT('Ctrl Pts',(9.16897630005181,-40.4901460881459,8.77627054946899));
#42084=CARTESIAN_POINT('Ctrl Pts',(3.84984706557644,-40.7284188590102,12.0946935166284));
#42085=CARTESIAN_POINT('Ctrl Pts',(-0.32088071557368,-40.8872742220127,
12.3384797159896));
#42086=CARTESIAN_POINT('Ctrl Pts',(-2.30975236282056,-40.9667121771536,
11.9541908119849));
#42087=CARTESIAN_POINT('Ctrl Pts',(-3.00369270810988,-19.6780228441179,
11.2217787630359));
#42088=CARTESIAN_POINT('Ctrl Pts',(-4.87022721769824,-19.7574402519795,
10.7221702594042));
#42089=CARTESIAN_POINT('Ctrl Pts',(-8.34726868959891,-19.916275067703,8.77397504146546));
#42090=CARTESIAN_POINT('Ctrl Pts',(-11.5282045966303,-20.154527291288,3.70865485023876));
#42091=CARTESIAN_POINT('Ctrl Pts',(-11.8972266216495,-20.3927795148732,
-2.25985124607116));
#42092=CARTESIAN_POINT('Ctrl Pts',(-9.36510883582578,-20.6310317384582,
-7.67784818830401));
#42093=CARTESIAN_POINT('Ctrl Pts',(-4.54898211085908,-20.8692839620433,
-11.2231380018903));
#42094=CARTESIAN_POINT('Ctrl Pts',(1.3764484894743,-21.1075361856285,-12.031573942001));
#42095=CARTESIAN_POINT('Ctrl Pts',(6.96623396044474,-21.3457884092135,-9.90577847614093));
#42096=CARTESIAN_POINT('Ctrl Pts',(10.8571383270859,-21.5840406327987,-5.364283505194));
#42097=CARTESIAN_POINT('Ctrl Pts',(12.1003045308358,-21.8222928563837,0.485425394929287));
#42098=CARTESIAN_POINT('Ctrl Pts',(10.3925481951215,-22.0605450799689,6.21674374369965));
#42099=CARTESIAN_POINT('Ctrl Pts',(6.15034811400611,-22.2987973035539,10.431980418571));
#42100=CARTESIAN_POINT('Ctrl Pts',(0.408252833052742,-22.5370495271391,
12.1031527538748));
#42101=CARTESIAN_POINT('Ctrl Pts',(-5.43340317505451,-22.7753017507242,
10.8227129534321));
#42102=CARTESIAN_POINT('Ctrl Pts',(-9.95000757532424,-23.0135539743092,
6.90292201716564));
#42103=CARTESIAN_POINT('Ctrl Pts',(-12.0400892004407,-23.2518061978944,
1.2997058422424));
#42104=CARTESIAN_POINT('Ctrl Pts',(-11.1939370164893,-23.4900584214795,
-4.62047160536659));
#42105=CARTESIAN_POINT('Ctrl Pts',(-7.61790328489481,-23.7283106450646,
-9.41384792823294));
#42106=CARTESIAN_POINT('Ctrl Pts',(-2.18408053856523,-23.9665628686497,
-11.911455653472));
#42107=CARTESIAN_POINT('Ctrl Pts',(3.78237707693078,-24.2048150922347,-11.5041995413608));
#42108=CARTESIAN_POINT('Ctrl Pts',(8.82642095160353,-24.4430673158199,-8.29139775151294));
#42109=CARTESIAN_POINT('Ctrl Pts',(11.7179528573444,-24.6813195394049,-3.05656086386032));
#42110=CARTESIAN_POINT('Ctrl Pts',(11.7518107472756,-24.9195717629901,2.92368391516781));
#42111=CARTESIAN_POINT('Ctrl Pts',(8.91973765043983,-25.1578239865751,8.19092569431719));
#42112=CARTESIAN_POINT('Ctrl Pts',(3.9123953050936,-25.3960762101603,11.4606346444945));
#42113=CARTESIAN_POINT('Ctrl Pts',(-2.04906850960975,-25.6343284337454,
11.9354221426448));
#42114=CARTESIAN_POINT('Ctrl Pts',(-7.51082304016482,-25.8725806573305,
9.49950107840742));
#42115=CARTESIAN_POINT('Ctrl Pts',(-11.1409023545732,-26.1108328809156,
4.74692302501242));
#42116=CARTESIAN_POINT('Ctrl Pts',(-12.0540337900549,-26.3490851045007,
-1.16329397307453));
#42117=CARTESIAN_POINT('Ctrl Pts',(-10.0275306702439,-26.5873373280858,
-6.78981679699862));
#42118=CARTESIAN_POINT('Ctrl Pts',(-5.55559922529289,-26.8255895516709,
-10.7604972342117));
#42119=CARTESIAN_POINT('Ctrl Pts',(0.271184192238789,-27.063841775256,-12.1069997362434));
#42120=CARTESIAN_POINT('Ctrl Pts',(6.03183353081841,-27.3020939988411,-10.500950801524));
#42121=CARTESIAN_POINT('Ctrl Pts',(10.3214909518584,-27.5403462224262,-6.3340198934194));
#42122=CARTESIAN_POINT('Ctrl Pts',(12.0940315311332,-27.7785984460113,-0.622402444953652));
#42123=CARTESIAN_POINT('Ctrl Pts',(10.9171832484849,-28.0168506695964,5.24100118284009));
#42124=CARTESIAN_POINT('Ctrl Pts',(7.07794578702809,-28.2551028931814,9.82627431509112));
#42125=CARTESIAN_POINT('Ctrl Pts',(1.51259950769554,-28.4933551167666,12.0151997989567));
#42126=CARTESIAN_POINT('Ctrl Pts',(-4.42162658884796,-28.7316073403516,
11.2739612287927));
#42127=CARTESIAN_POINT('Ctrl Pts',(-9.27754425042827,-28.9698595639368,
7.78332552068034));
#42128=CARTESIAN_POINT('Ctrl Pts',(-11.870933853621,-29.2081117875218,2.39455902463984));
#42129=CARTESIAN_POINT('Ctrl Pts',(-11.5693417463421,-29.446364011107,-3.57817202435472));
#42130=CARTESIAN_POINT('Ctrl Pts',(-8.44631762951329,-29.6846162346921,
-8.678289116001));
#42131=CARTESIAN_POINT('Ctrl Pts',(-3.26347788572639,-29.9228684582772,
-11.6620193606813));
#42132=CARTESIAN_POINT('Ctrl Pts',(2.71523090325989,-30.1611206818622,-11.801716172723));
#42133=CARTESIAN_POINT('Ctrl Pts',(8.03177242709483,-30.3993729054474,-9.06331148967571));
#42134=CARTESIAN_POINT('Ctrl Pts',(11.3895940586429,-30.6376251290325,-4.11462399969371));
#42135=CARTESIAN_POINT('Ctrl Pts',(11.9698190077354,-30.8758773526176,1.83750276233406));
#42136=CARTESIAN_POINT('Ctrl Pts',(9.63094698161567,-31.1141295762027,7.34151508319886));
#42137=CARTESIAN_POINT('Ctrl Pts',(4.94336206482527,-31.3523817997878,11.0551415628917));
#42138=CARTESIAN_POINT('Ctrl Pts',(-0.949767667762671,-31.5906340233729,
12.0727347712439));
#42139=CARTESIAN_POINT('Ctrl Pts',(-6.61127619335253,-31.828886246958,10.1461327891339));
#42140=CARTESIAN_POINT('Ctrl Pts',(-10.6604832859937,-32.0671384705431,
5.7451788125851));
#42141=CARTESIAN_POINT('Ctrl Pts',(-12.1099029888395,-32.3053906941281,
-0.0568601831300151));
#42142=CARTESIAN_POINT('Ctrl Pts',(-10.6060632345463,-32.5436429177133,
-5.84503260421468));
#42143=CARTESIAN_POINT('Ctrl Pts',(-6.51570758666586,-32.7818951412983,
-10.2077685183684));
#42144=CARTESIAN_POINT('Ctrl Pts',(-0.836356959386205,-33.0201473648835,
-12.0811212441569));
#42145=CARTESIAN_POINT('Ctrl Pts',(5.04695724234298,-33.2583995884685,-11.0082335582726));
#42146=CARTESIAN_POINT('Ctrl Pts',(9.69946272335483,-33.4966518120537,-7.25075212359403));
#42147=CARTESIAN_POINT('Ctrl Pts',(11.9865462812223,-33.7349040356388,-1.72501934122564));
#42148=CARTESIAN_POINT('Ctrl Pts',(11.3504535596434,-33.9731562592238,4.22139638863183));
#42149=CARTESIAN_POINT('Ctrl Pts',(7.94630940537469,-34.211408482809,9.13833411041546));
#42150=CARTESIAN_POINT('Ctrl Pts',(2.6042873488569,-34.4496607063941,11.8266931508312));
#42151=CARTESIAN_POINT('Ctrl Pts',(-3.37284600870548,-34.6879129299792,
11.630859524634));
#42152=CARTESIAN_POINT('Ctrl Pts',(-8.52743855952799,-34.9261651535643,
8.5985914597323));
#42153=CARTESIAN_POINT('Ctrl Pts',(-11.6024324057451,-35.1644173771494,
3.46937253010039));
#42154=CARTESIAN_POINT('Ctrl Pts',(-11.8479243752835,-35.4026696007345,
-2.5059272681298));
#42155=CARTESIAN_POINT('Ctrl Pts',(-9.20404598979087,-35.6409218243196,
-7.8701029789477));
#42156=CARTESIAN_POINT('Ctrl Pts',(-4.31556367068634,-35.8791740479047,
-11.3149853598205));
#42157=CARTESIAN_POINT('Ctrl Pts',(1.62536136349889,-36.1174262714898,-12.0004659858516));
#42158=CARTESIAN_POINT('Ctrl Pts',(7.16990719156578,-36.3556784950749,-9.75937572019344));
#42159=CARTESIAN_POINT('Ctrl Pts',(10.965917427667,-36.59393071866,-5.1382524503469));
#42160=CARTESIAN_POINT('Ctrl Pts',(12.0876536389402,-36.8321829422451,0.735943809094519));
#42161=CARTESIAN_POINT('Ctrl Pts',(10.2615563171244,-37.0704351658302,6.43066444322939));
#42162=CARTESIAN_POINT('Ctrl Pts',(5.93295861336892,-37.3086873894153,10.5571295917087));
#42163=CARTESIAN_POINT('Ctrl Pts',(0.157481530964674,-37.5469396130003,
12.1090125651303));
#42164=CARTESIAN_POINT('Ctrl Pts',(-5.65640033822935,-37.7851918365855,
10.7078528273879));
#42165=CARTESIAN_POINT('Ctrl Pts',(-10.0908486473709,-38.0234440601705,
6.69535443070501));
#42166=CARTESIAN_POINT('Ctrl Pts',(-12.0644253281625,-38.2616962837557,
1.05004869598765));
#42167=CARTESIAN_POINT('Ctrl Pts',(-11.0958369830495,-38.4999485073408,
-4.85133066267378));
#42168=CARTESIAN_POINT('Ctrl Pts',(-7.42128342921687,-38.7382007309259,
-9.56961558479783));
#42169=CARTESIAN_POINT('Ctrl Pts',(-1.93690584525694,-38.976452954511,-11.954131443005));
#42170=CARTESIAN_POINT('Ctrl Pts',(4.01985793539565,-39.2147051780961,-11.4234024767251));
#42171=CARTESIAN_POINT('Ctrl Pts',(8.99623257718483,-39.4529574016812,-8.10677890851787));
#42172=CARTESIAN_POINT('Ctrl Pts',(11.7788047335206,-39.6912096252663,-2.8132499638494));
#42173=CARTESIAN_POINT('Ctrl Pts',(11.6886183926944,-39.9294618488514,3.16656422818516));
#42174=CARTESIAN_POINT('Ctrl Pts',(8.74840425861466,-40.1677140724365,8.3737115395636));
#42175=CARTESIAN_POINT('Ctrl Pts',(3.67325831819566,-40.4059868433008,11.5399216668183));
#42176=CARTESIAN_POINT('Ctrl Pts',(-0.306162228668456,-40.5648422063033,
11.7725256298878));
#42177=CARTESIAN_POINT('Ctrl Pts',(-2.20380626429698,-40.6442801614442,
11.4058636848336));
#42178=CARTESIAN_POINT('Ctrl Pts',(-2.85929275392902,-19.3555908284084,
10.6823013608252));
#42179=CARTESIAN_POINT('Ctrl Pts',(-4.63609521571708,-19.4350082362701,
10.2067111080746));
#42180=CARTESIAN_POINT('Ctrl Pts',(-7.94598089705643,-19.5938430519935,
8.35217370654499));
#42181=CARTESIAN_POINT('Ctrl Pts',(-10.9739960349335,-19.8320952755786,
3.53036444489831));
#42182=CARTESIAN_POINT('Ctrl Pts',(-11.3252776421793,-20.0703474991637,
-2.15121083305315));
#42183=CARTESIAN_POINT('Ctrl Pts',(-8.91488925006696,-20.3085997227488,
-7.3087422129806));
#42184=CARTESIAN_POINT('Ctrl Pts',(-4.33029369223223,-20.5468519463339,
-10.683595255436));
#42185=CARTESIAN_POINT('Ctrl Pts',(1.31027690731619,-20.785104169919,-11.4531663301778));
#42186=CARTESIAN_POINT('Ctrl Pts',(6.6313382296047,-21.0233563935041,-9.42956666052528));
#42187=CARTESIAN_POINT('Ctrl Pts',(10.3351907015071,-21.2616086170892,-5.10640017036693));
#42188=CARTESIAN_POINT('Ctrl Pts',(11.5185927548245,-21.4998608406743,0.462088984850871));
#42189=CARTESIAN_POINT('Ctrl Pts',(9.89293534220016,-21.7381130642594,5.91787911306662));
#42190=CARTESIAN_POINT('Ctrl Pts',(5.85467539640056,-21.9763652878445,9.93047189528233));
#42191=CARTESIAN_POINT('Ctrl Pts',(0.388626427785698,-22.2146175114296,
11.5213040519803));
#42192=CARTESIAN_POINT('Ctrl Pts',(-5.17219697130215,-22.4528697350147,
10.3024202982052));
#42193=CARTESIAN_POINT('Ctrl Pts',(-9.47166948364905,-22.6911219585998,
6.57106995376998));
#42194=CARTESIAN_POINT('Ctrl Pts',(-11.4612722248617,-22.9293741821849,
1.23722359711736));
#42195=CARTESIAN_POINT('Ctrl Pts',(-10.6557980823965,-23.16762640577,-4.39834639052438));
#42196=CARTESIAN_POINT('Ctrl Pts',(-7.25167910945802,-23.4058786293551,
-8.96128525235328));
#42197=CARTESIAN_POINT('Ctrl Pts',(-2.07908273741047,-23.6441308529403,
-11.3388226254846));
#42198=CARTESIAN_POINT('Ctrl Pts',(3.6005425386876,-23.8823830765253,-10.9511450021349));
#42199=CARTESIAN_POINT('Ctrl Pts',(8.40209832447484,-24.1206353001105,-7.89279590646365));
#42200=CARTESIAN_POINT('Ctrl Pts',(11.1546223105393,-24.3588875236955,-2.90961931837506));
#42201=CARTESIAN_POINT('Ctrl Pts',(11.1868525114124,-24.5971397472806,2.78313031517747));
#42202=CARTESIAN_POINT('Ctrl Pts',(8.49092890294339,-24.8353919708657,7.79715395735995));
#42203=CARTESIAN_POINT('Ctrl Pts',(3.72431025189639,-25.0736441944508,10.9096744503706));
#42204=CARTESIAN_POINT('Ctrl Pts',(-1.95056129610478,-25.3118964180359,
11.3616369462185));
#42205=CARTESIAN_POINT('Ctrl Pts',(-7.14974665577569,-25.550148641621,9.04282070069786));
#42206=CARTESIAN_POINT('Ctrl Pts',(-10.6053130164261,-25.7884008652061,
4.51871876648054));
#42207=CARTESIAN_POINT('Ctrl Pts',(-11.4745464402741,-26.0266530887912,
-1.1073696117185));
#42208=CARTESIAN_POINT('Ctrl Pts',(-9.54546572218151,-26.2649053123763,
-6.46340217018414));
#42209=CARTESIAN_POINT('Ctrl Pts',(-5.28851855109026,-26.5031575359614,
-10.2431955463965));
#42210=CARTESIAN_POINT('Ctrl Pts',(0.258147244475094,-26.7414097595465,
-11.5249660939666));
#42211=CARTESIAN_POINT('Ctrl Pts',(5.74185830028796,-26.9796619831316,-9.9961265861502));
#42212=CARTESIAN_POINT('Ctrl Pts',(9.82529411504405,-27.2179142067167,-6.02951731233948));
#42213=CARTESIAN_POINT('Ctrl Pts',(11.5126213242094,-27.4561664303018,-0.592480980520653));
#42214=CARTESIAN_POINT('Ctrl Pts',(10.3923490147401,-27.6944186538869,4.98904454006482));
#42215=CARTESIAN_POINT('Ctrl Pts',(6.73767960580988,-27.932670877472,9.35388459392002));
#42216=CARTESIAN_POINT('Ctrl Pts',(1.43988258195426,-28.1709231010571,11.4375793600353));
#42217=CARTESIAN_POINT('Ctrl Pts',(-4.2090606778576,-28.4091753246422,10.7319751992368));
#42218=CARTESIAN_POINT('Ctrl Pts',(-8.83153425711049,-28.6474275482273,
7.40914881294773));
#42219=CARTESIAN_POINT('Ctrl Pts',(-11.3002488764531,-28.8856797718124,
2.27944265054878));
#42220=CARTESIAN_POINT('Ctrl Pts',(-11.0131555514081,-29.1239319953975,
-3.40615446910582));
#42221=CARTESIAN_POINT('Ctrl Pts',(-8.04026814402308,-29.3621842189826,
-8.2610877999891));
#42222=CARTESIAN_POINT('Ctrl Pts',(-3.10658898164615,-29.6004364425677,
-11.1013777688193));
#42223=CARTESIAN_POINT('Ctrl Pts',(2.58469850327018,-29.8386886661528,-11.2343587762771));
#42224=CARTESIAN_POINT('Ctrl Pts',(7.64565184713929,-30.0769408897379,-8.62760055283371));
#42225=CARTESIAN_POINT('Ctrl Pts',(10.8420490798353,-30.315193113323,-3.91681697521912));
#42226=CARTESIAN_POINT('Ctrl Pts',(11.3943802114819,-30.5534453369081,1.74916639091636));
#42227=CARTESIAN_POINT('Ctrl Pts',(9.16794745469711,-30.7916975604932,6.98857803382302));
#42228=CARTESIAN_POINT('Ctrl Pts',(4.70571416771088,-31.0299497840783,10.5236751013477));
#42229=CARTESIAN_POINT('Ctrl Pts',(-0.904108400642208,-31.2682020076634,
11.4923483878104));
#42230=CARTESIAN_POINT('Ctrl Pts',(-6.29344475313245,-31.5064542312485,
9.65836614579251));
#42231=CARTESIAN_POINT('Ctrl Pts',(-10.1479896830738,-31.7447064548336,
5.46898426210454));
#42232=CARTESIAN_POINT('Ctrl Pts',(-11.527729775181,-31.9829586784187,-0.0541266785286571));
#42233=CARTESIAN_POINT('Ctrl Pts',(-10.0961858289872,-32.2212109020038,
-5.56403766822958));
#42234=CARTESIAN_POINT('Ctrl Pts',(-6.20247052535459,-32.4594631255889,
-9.71703879013706));
#42235=CARTESIAN_POINT('Ctrl Pts',(-0.79614981493094,-32.6977153491741,
-11.5003316882214));
#42236=CARTESIAN_POINT('Ctrl Pts',(4.80432909580209,-32.9359675727591,-10.4790221588725));
#42237=CARTESIAN_POINT('Ctrl Pts',(9.23316936083815,-33.1742197963443,-6.90217842575973));
#42238=CARTESIAN_POINT('Ctrl Pts',(11.4103033356234,-33.4124720199293,-1.64209051393198));
#42239=CARTESIAN_POINT('Ctrl Pts',(10.8047902268,-33.6507242435144,4.01845637301311));
#42240=CARTESIAN_POINT('Ctrl Pts',(7.56429738698645,-33.8889764670995,8.69901652534074));
#42241=CARTESIAN_POINT('Ctrl Pts',(2.47908846521831,-34.1272286906846,11.2581350075564));
#42242=CARTESIAN_POINT('Ctrl Pts',(-3.21069932579042,-34.3654809142697,
11.0717159152007));
#42243=CARTESIAN_POINT('Ctrl Pts',(-8.11748925481006,-34.6037331378548,
8.18522154028186));
#42244=CARTESIAN_POINT('Ctrl Pts',(-11.0446554057036,-34.8419853614399,
3.30258541734742));
#42245=CARTESIAN_POINT('Ctrl Pts',(-11.2783455590783,-35.080237585025,-2.38545696112353));
#42246=CARTESIAN_POINT('Ctrl Pts',(-8.76156936239957,-35.3184898086102,
-7.49175451923665));
#42247=CARTESIAN_POINT('Ctrl Pts',(-4.10809664364021,-35.5567420321952,
-10.771027130304));
#42248=CARTESIAN_POINT('Ctrl Pts',(1.5472235081241,-35.7949942557803,-11.4235538623753));
#42249=CARTESIAN_POINT('Ctrl Pts',(6.82522004459241,-36.0332464793655,-9.2902020916712));
#42250=CARTESIAN_POINT('Ctrl Pts',(10.4387403400005,-36.2714987029505,-4.89123536487858));
#42251=CARTESIAN_POINT('Ctrl Pts',(11.5065500437207,-36.5097509265356,0.70056394083236));
#42252=CARTESIAN_POINT('Ctrl Pts',(9.76824078653887,-36.7480031501207,6.12151575819658));
#42253=CARTESIAN_POINT('Ctrl Pts',(5.64773670980524,-36.9862553737058,10.0496046291158));
#42254=CARTESIAN_POINT('Ctrl Pts',(0.149910741251658,-37.2245075972909,
11.5268821578289));
#42255=CARTESIAN_POINT('Ctrl Pts',(-5.38447373686177,-37.4627598208761,
10.1930819743391));
#42256=CARTESIAN_POINT('Ctrl Pts',(-9.60573974179206,-37.7010120444611,
6.37348100123998));
#42257=CARTESIAN_POINT('Ctrl Pts',(-11.4844384140878,-37.9392642680463,
0.999568504329265));
#42258=CARTESIAN_POINT('Ctrl Pts',(-10.5624141240384,-38.1775164916313,
-4.61810709638991));
#42259=CARTESIAN_POINT('Ctrl Pts',(-7.06451158493042,-38.4157687152165,
-9.10956451224892));
#42260=CARTESIAN_POINT('Ctrl Pts',(-1.84379075576973,-38.6540209388015,
-11.379446812989));
#42261=CARTESIAN_POINT('Ctrl Pts',(3.82660670829195,-38.8922731623866,-10.8742321871762));
#42262=CARTESIAN_POINT('Ctrl Pts',(8.56374640160554,-39.1305253859717,-7.71705245621344));
#42263=CARTESIAN_POINT('Ctrl Pts',(11.2125487848899,-39.3687776095568,-2.67800538147839));
#42264=CARTESIAN_POINT('Ctrl Pts',(11.1266980751514,-39.6070298331421,3.01433436518149));
#42265=CARTESIAN_POINT('Ctrl Pts',(8.32783221717754,-39.845282056727,7.97115252965823));
#42266=CARTESIAN_POINT('Ctrl Pts',(3.49666957081488,-40.0835548275914,10.9851498170082));
#42267=CARTESIAN_POINT('Ctrl Pts',(-0.291443741763231,-40.2424101905938,
11.2065715437861));
#42268=CARTESIAN_POINT('Ctrl Pts',(-2.09786016577339,-40.3218481457347,
10.8575365576823));
#42269=CARTESIAN_POINT('Ctrl Pts',(-2.71489279974816,-19.033158812699,10.1428239586147));
#42270=CARTESIAN_POINT('Ctrl Pts',(-4.40196321373591,-19.1125762205607,
9.69125195674494));
#42271=CARTESIAN_POINT('Ctrl Pts',(-7.54469310451393,-19.2714110362841,
7.93037237162453));
#42272=CARTESIAN_POINT('Ctrl Pts',(-10.4197874732365,-19.5096632598692,
3.35207403955784));
#42273=CARTESIAN_POINT('Ctrl Pts',(-10.7533286627092,-19.7479154834543,
-2.04257042003514));
#42274=CARTESIAN_POINT('Ctrl Pts',(-8.46466966430815,-19.9861677070394,
-6.9396362376572));
#42275=CARTESIAN_POINT('Ctrl Pts',(-4.11160527360535,-20.2244199306245,
-10.1440525089817));
#42276=CARTESIAN_POINT('Ctrl Pts',(1.24410532515808,-20.4626721542096,-10.8747587183546));
#42277=CARTESIAN_POINT('Ctrl Pts',(6.29644249876465,-20.7009243777947,-8.95335484490964));
#42278=CARTESIAN_POINT('Ctrl Pts',(9.81324307592822,-20.9391766013798,-4.84851683553984));
#42279=CARTESIAN_POINT('Ctrl Pts',(10.936880978813,-21.1774288249649,0.438752574772446));
#42280=CARTESIAN_POINT('Ctrl Pts',(9.39332248927878,-21.41568104855,5.6190144824336));
#42281=CARTESIAN_POINT('Ctrl Pts',(5.55900267879502,-21.6539332721351,9.42896337199362));
#42282=CARTESIAN_POINT('Ctrl Pts',(0.369000022518657,-21.8921854957201,
10.9394553500859));
#42283=CARTESIAN_POINT('Ctrl Pts',(-4.9109907675498,-22.1304377193054,9.78212764297827));
#42284=CARTESIAN_POINT('Ctrl Pts',(-8.99333139197383,-22.3686899428904,
6.23921789037432));
#42285=CARTESIAN_POINT('Ctrl Pts',(-10.8824552492826,-22.6069421664755,
1.17474135199233));
#42286=CARTESIAN_POINT('Ctrl Pts',(-10.1176591483038,-22.8451943900606,
-4.17622117568216));
#42287=CARTESIAN_POINT('Ctrl Pts',(-6.88545493402124,-23.0834466136456,
-8.50872257647364));
#42288=CARTESIAN_POINT('Ctrl Pts',(-1.9740849362557,-23.3216988372308,-10.766189597497));
#42289=CARTESIAN_POINT('Ctrl Pts',(3.41870800044444,-23.5599510608158,-10.398090462909));
#42290=CARTESIAN_POINT('Ctrl Pts',(7.97777569734612,-23.798203284401,-7.49419406141432));
#42291=CARTESIAN_POINT('Ctrl Pts',(10.5912917637341,-24.0364555079861,-2.76267777288981));
#42292=CARTESIAN_POINT('Ctrl Pts',(10.6218942755493,-24.2747077315712,2.64257671518715));
#42293=CARTESIAN_POINT('Ctrl Pts',(8.06212015544694,-24.5129599551563,7.4033822204027));
#42294=CARTESIAN_POINT('Ctrl Pts',(3.53622519869919,-24.7512121787415,10.3587142562468));
#42295=CARTESIAN_POINT('Ctrl Pts',(-1.85205408259982,-24.9894644023266,
10.7878517497922));
#42296=CARTESIAN_POINT('Ctrl Pts',(-6.78867027138654,-25.2277166259116,
8.5861403229883));
#42297=CARTESIAN_POINT('Ctrl Pts',(-10.0697236782791,-25.4659688494967,
4.29051450794865));
#42298=CARTESIAN_POINT('Ctrl Pts',(-10.8950590904933,-25.7042210730818,
-1.05144525036246));
#42299=CARTESIAN_POINT('Ctrl Pts',(-9.06340077411912,-25.9424732966669,
-6.13698754336968));
#42300=CARTESIAN_POINT('Ctrl Pts',(-5.02143787688763,-26.180725520252,-9.72589385858134));
#42301=CARTESIAN_POINT('Ctrl Pts',(0.245110296711381,-26.4189777438371,
-10.9429324516899));
#42302=CARTESIAN_POINT('Ctrl Pts',(5.45188306975753,-26.6572299674222,-9.49130237077641));
#42303=CARTESIAN_POINT('Ctrl Pts',(9.32909727822968,-26.8954821910073,-5.72501473125955));
#42304=CARTESIAN_POINT('Ctrl Pts',(10.9312111172857,-27.1337344145924,-0.562559516087659));
#42305=CARTESIAN_POINT('Ctrl Pts',(9.86751478099552,-27.3719866381775,4.73708789728954));
#42306=CARTESIAN_POINT('Ctrl Pts',(6.3974134245917,-27.6102388617627,8.8814948727489));
#42307=CARTESIAN_POINT('Ctrl Pts',(1.367165656213,-27.8484910853478,10.8599589211139));
#42308=CARTESIAN_POINT('Ctrl Pts',(-3.99649476686722,-28.0867433089328,
10.1899891696809));
#42309=CARTESIAN_POINT('Ctrl Pts',(-8.38552426379272,-28.3249955325179,
7.03497210521514));
#42310=CARTESIAN_POINT('Ctrl Pts',(-10.7295638992853,-28.563247756103,2.16432627645773));
#42311=CARTESIAN_POINT('Ctrl Pts',(-10.4569693564742,-28.8014999796881,
-3.23413691385691));
#42312=CARTESIAN_POINT('Ctrl Pts',(-7.63421865853288,-29.0397522032732,
-7.84388648397718));
#42313=CARTESIAN_POINT('Ctrl Pts',(-2.94970007756592,-29.2780044268583,
-10.5407361769574));
#42314=CARTESIAN_POINT('Ctrl Pts',(2.45416610328047,-29.5162566504434,-10.6670013798312));
#42315=CARTESIAN_POINT('Ctrl Pts',(7.25953126718375,-29.7545088740285,-8.19188961599172));
#42316=CARTESIAN_POINT('Ctrl Pts',(10.2945041010277,-29.9927610976136,-3.71900995074453));
#42317=CARTESIAN_POINT('Ctrl Pts',(10.8189414152284,-30.2310133211987,1.66083001949865));
#42318=CARTESIAN_POINT('Ctrl Pts',(8.70494792777857,-30.4692655447839,6.63564098444718));
#42319=CARTESIAN_POINT('Ctrl Pts',(4.46806627059647,-30.7075177683689,9.9922086398038));
#42320=CARTESIAN_POINT('Ctrl Pts',(-0.858449133521731,-30.945769991954,
10.911962004377));
#42321=CARTESIAN_POINT('Ctrl Pts',(-5.97561331291237,-31.1840222155391,
9.17059950245109));
#42322=CARTESIAN_POINT('Ctrl Pts',(-9.63549608015401,-31.4222744391242,
5.19278971162398));
#42323=CARTESIAN_POINT('Ctrl Pts',(-10.9455565615224,-31.6605266627093,
-0.0513931739272948));
#42324=CARTESIAN_POINT('Ctrl Pts',(-9.58630842342817,-31.8987788862944,
-5.28304273224449));
#42325=CARTESIAN_POINT('Ctrl Pts',(-5.88923346404332,-32.1370311098795,
-9.22630906190571));
#42326=CARTESIAN_POINT('Ctrl Pts',(-0.755942670475671,-32.3752833334646,
-10.919542132286));
#42327=CARTESIAN_POINT('Ctrl Pts',(4.56170094926121,-32.6135355570497,-9.94981075947233));
#42328=CARTESIAN_POINT('Ctrl Pts',(8.76687599832148,-32.8517877806348,-6.55360472792545));
#42329=CARTESIAN_POINT('Ctrl Pts',(10.8340603900244,-33.09004000422,-1.55916168663833));
#42330=CARTESIAN_POINT('Ctrl Pts',(10.2591268939567,-33.3282922278051,3.81551635739438));
#42331=CARTESIAN_POINT('Ctrl Pts',(7.18228536859824,-33.5665444513901,8.25969894026603));
#42332=CARTESIAN_POINT('Ctrl Pts',(2.35388958157973,-33.8047966749752,10.6895768642816));
#42333=CARTESIAN_POINT('Ctrl Pts',(-3.04855264287536,-34.0430488985603,
10.5125723057673));
#42334=CARTESIAN_POINT('Ctrl Pts',(-7.70753995009214,-34.2813011221453,
7.77185162083141));
#42335=CARTESIAN_POINT('Ctrl Pts',(-10.4868784056621,-34.5195533457305,
3.13579830459444));
#42336=CARTESIAN_POINT('Ctrl Pts',(-10.7087667428733,-34.7578055693156,
-2.26498665411725));
#42337=CARTESIAN_POINT('Ctrl Pts',(-8.31909273500825,-34.9960577929007,
-7.11340605952559));
#42338=CARTESIAN_POINT('Ctrl Pts',(-3.90062961659408,-35.2343100164858,
-10.2270689007874));
#42339=CARTESIAN_POINT('Ctrl Pts',(1.46908565274932,-35.4725622400709,-10.846641738899));
#42340=CARTESIAN_POINT('Ctrl Pts',(6.48053289761904,-35.710814463656,-8.82102846314895));
#42341=CARTESIAN_POINT('Ctrl Pts',(9.91156325233417,-35.9490666872412,-4.64421827941024));
#42342=CARTESIAN_POINT('Ctrl Pts',(10.9254464485013,-36.1873189108262,0.665184072570199));
#42343=CARTESIAN_POINT('Ctrl Pts',(9.27492525595335,-36.4255711344113,5.81236707316378));
#42344=CARTESIAN_POINT('Ctrl Pts',(5.36251480624159,-36.6638233579963,9.54207966652283));
#42345=CARTESIAN_POINT('Ctrl Pts',(0.142339951538634,-36.9020755815815,
10.9447517505275));
#42346=CARTESIAN_POINT('Ctrl Pts',(-5.11254713549418,-37.1403278051666,
9.67831112129032));
#42347=CARTESIAN_POINT('Ctrl Pts',(-9.12063083621321,-37.3785800287517,
6.05160757177495));
#42348=CARTESIAN_POINT('Ctrl Pts',(-10.9044515000132,-37.6168322523368,
0.949088312670873));
#42349=CARTESIAN_POINT('Ctrl Pts',(-10.0289912650274,-37.8550844759219,
-4.38488353010602));
#42350=CARTESIAN_POINT('Ctrl Pts',(-6.707739740644,-38.093336699507,-8.64951343970004));
#42351=CARTESIAN_POINT('Ctrl Pts',(-1.75067566628252,-38.3315889230921,
-10.8047621829729));
#42352=CARTESIAN_POINT('Ctrl Pts',(3.63335548118823,-38.5698411466772,-10.3250618976272));
#42353=CARTESIAN_POINT('Ctrl Pts',(8.13126022602624,-38.8080933702623,-7.32732600390901));
#42354=CARTESIAN_POINT('Ctrl Pts',(10.6462928362593,-39.0463455938474,-2.54276079910738));
#42355=CARTESIAN_POINT('Ctrl Pts',(10.5647777576085,-39.2845978174325,2.86210450217782));
#42356=CARTESIAN_POINT('Ctrl Pts',(7.90726017574041,-39.5228500410176,7.56859351975284));
#42357=CARTESIAN_POINT('Ctrl Pts',(3.32008082343409,-39.7611228118819,10.430377967198));
#42358=CARTESIAN_POINT('Ctrl Pts',(-0.276725254858005,-39.9199781748845,
10.6406174576843));
#42359=CARTESIAN_POINT('Ctrl Pts',(-1.99191406724981,-39.9994161300253,
10.309209430531));
#42360=CARTESIAN_POINT('Ctrl Pts',(-1.99079507083261,-40.,10.3105642903746));
#42361=CARTESIAN_POINT('Ctrl Pts',(-1.74787308387827,-40.,10.3776190639041));
#42362=CARTESIAN_POINT('Ctrl Pts',(-1.50291730396267,-40.,10.4356201925428));
#42363=CARTESIAN_POINT('Ctrl Pts',(-1.25645144932134,-40.,10.4847082098124));
#42364=CARTESIAN_POINT('Ctrl Pts',(-1.00610937592225,-40.,10.5345682443401));
#42365=CARTESIAN_POINT('Ctrl Pts',(-0.754208864891479,-40.,10.5752327782703));
#42366=CARTESIAN_POINT('Ctrl Pts',(-0.501269405627775,-40.,10.6068040933286));
#42367=CARTESIAN_POINT('Ctrl Pts',(-0.244349089886426,-40.,10.6388722896344));
#42368=CARTESIAN_POINT('Ctrl Pts',(0.0136436911868619,-40.,10.6615589819356));
#42369=CARTESIAN_POINT('Ctrl Pts',(0.272186557320881,-40.,10.6749225226571));
#42370=CARTESIAN_POINT('Ctrl Pts',(0.531566238246189,-40.,10.6883293165871));
#42371=CARTESIAN_POINT('Ctrl Pts',(0.791500205704512,-40.,10.6923526126214));
#42372=CARTESIAN_POINT('Ctrl Pts',(1.05147390013315,-40.,10.6870004794339));
#42373=CARTESIAN_POINT('Ctrl Pts',(1.31028376057683,-40.,10.6816723063417));
#42374=CARTESIAN_POINT('Ctrl Pts',(1.56913364179828,-40.,10.6670525037355));
#42375=CARTESIAN_POINT('Ctrl Pts',(1.82751901150857,-40.,10.6430977083202));
#42376=CARTESIAN_POINT('Ctrl Pts',(1.90159764111365,-40.,10.63622991074));
#42377=CARTESIAN_POINT('Ctrl Pts',(1.97563807578317,-40.,10.6285944888747));
#42378=CARTESIAN_POINT('Ctrl Pts',(2.04962835769163,-40.,10.6201896290691));
#42379=CARTESIAN_POINT('Ctrl Pts',(2.08954125923063,-40.,10.6156557587659));
#42380=CARTESIAN_POINT('Ctrl Pts',(2.12944528573599,-40.,10.6108972103674));
#42381=CARTESIAN_POINT('Ctrl Pts',(2.1693057513364,-40.,10.6059179310049));
#42382=CARTESIAN_POINT('Ctrl Pts',(2.43279869411486,-40.,10.5730029875293));
#42383=CARTESIAN_POINT('Ctrl Pts',(2.69461388759026,-40.,10.5304238386819));
#42384=CARTESIAN_POINT('Ctrl Pts',(2.95420990430362,-40.,10.4782725649795));
#42385=CARTESIAN_POINT('Ctrl Pts',(3.07376860221232,-40.,10.4542539438269));
#42386=CARTESIAN_POINT('Ctrl Pts',(3.19285681334827,-40.,10.4282042572862));
#42387=CARTESIAN_POINT('Ctrl Pts',(3.31142253876288,-40.,10.4001289044428));
#42388=CARTESIAN_POINT('Ctrl Pts',(3.56622266861186,-40.,10.3397944062138));
#42389=CARTESIAN_POINT('Ctrl Pts',(3.81860986323782,-40.,10.2701083948083));
#42390=CARTESIAN_POINT('Ctrl Pts',(4.06816673278712,-40.,10.1914106777717));
#42391=CARTESIAN_POINT('Ctrl Pts',(4.32019405273534,-40.,10.1119339046154));
#42392=CARTESIAN_POINT('Ctrl Pts',(4.56933530406408,-40.,10.0232659758112));
#42393=CARTESIAN_POINT('Ctrl Pts',(4.815156586397,-40.,9.92570343373692));
#42394=CARTESIAN_POINT('Ctrl Pts',(5.06195033757761,-40.,9.82775493430386));
#42395=CARTESIAN_POINT('Ctrl Pts',(5.30539839959129,-40.,9.72084110382949));
#42396=CARTESIAN_POINT('Ctrl Pts',(5.54504887007903,-40.,9.60521113342298));
#42397=CARTESIAN_POINT('Ctrl Pts',(5.66474353971471,-40.,9.54745914537295));
#42398=CARTESIAN_POINT('Ctrl Pts',(5.78349062335036,-40.,9.48753209533787));
#42399=CARTESIAN_POINT('Ctrl Pts',(5.90123190287221,-40.,9.42545655152217));
#42400=CARTESIAN_POINT('Ctrl Pts',(5.95755289783563,-40.,9.39576300305053));
#42401=CARTESIAN_POINT('Ctrl Pts',(6.01364372866714,-40.,9.36557780581555));
#42402=CARTESIAN_POINT('Ctrl Pts',(6.06949789365341,-40.,9.33490363661388));
#42403=CARTESIAN_POINT('Ctrl Pts',(6.10987237433491,-40.,9.31273065001283));
#42404=CARTESIAN_POINT('Ctrl Pts',(6.15013052671072,-40.,9.29029793926035));
#42405=CARTESIAN_POINT('Ctrl Pts',(6.19023375294448,-40.,9.26762711136606));
#42406=CARTESIAN_POINT('Ctrl Pts',(6.42530159529298,-40.,9.1347404810909));
#42407=CARTESIAN_POINT('Ctrl Pts',(6.6551974805836,-40.,8.99359845953242));
#42408=CARTESIAN_POINT('Ctrl Pts',(6.87949236004535,-40.,8.84456214268246));
#42409=CARTESIAN_POINT('Ctrl Pts',(7.1090735464645,-40.,8.69201325470042));
#42410=CARTESIAN_POINT('Ctrl Pts',(7.33278726191541,-40.,8.53119349946645));
#42411=CARTESIAN_POINT('Ctrl Pts',(7.55016317409375,-40.,8.36243515486996));
#42412=CARTESIAN_POINT('Ctrl Pts',(7.76753908627209,-40.,8.19367681027347));
#42413=CARTESIAN_POINT('Ctrl Pts',(7.97857784575597,-40.,8.01697958779349));
#42414=CARTESIAN_POINT('Ctrl Pts',(8.18278913651048,-40.,7.83262450231714));
#42415=CARTESIAN_POINT('Ctrl Pts',(8.38288054194601,-40.,7.65198871075115));
#42416=CARTESIAN_POINT('Ctrl Pts',(8.57641773083012,-40.,7.46400053667575));
#42417=CARTESIAN_POINT('Ctrl Pts',(8.76315973735505,-40.,7.26911327773004));
#42418=CARTESIAN_POINT('Ctrl Pts',(8.95087399746834,-40.,7.07321135775353));
#42419=CARTESIAN_POINT('Ctrl Pts',(9.13172256231602,-40.,6.87033788456684));
#42420=CARTESIAN_POINT('Ctrl Pts',(9.30542514585722,-40.,6.66091475526788));
#42421=CARTESIAN_POINT('Ctrl Pts',(9.35096602916371,-40.,6.60600875387947));
#42422=CARTESIAN_POINT('Ctrl Pts',(9.39601551124977,-40.,6.55065236459227));
#42423=CARTESIAN_POINT('Ctrl Pts',(9.44056808201162,-40.,6.49485281517297));
#42424=CARTESIAN_POINT('Ctrl Pts',(9.45871046836229,-40.,6.47213051281313));
#42425=CARTESIAN_POINT('Ctrl Pts',(9.4767704796353,-40.,6.44933463079931));
#42426=CARTESIAN_POINT('Ctrl Pts',(9.49473878095482,-40.,6.42647721576431));
#42427=CARTESIAN_POINT('Ctrl Pts',(9.66342503031444,-40.,6.21189201131205));
#42428=CARTESIAN_POINT('Ctrl Pts',(9.82423055529978,-40.,5.99163828046608));
#42429=CARTESIAN_POINT('Ctrl Pts',(9.97696748002078,-40.,5.76623949569044));
#42430=CARTESIAN_POINT('Ctrl Pts',(10.1322964813989,-40.,5.53701550015035));
#42431=CARTESIAN_POINT('Ctrl Pts',(10.2792811504091,-40.,5.30246996694981));
#42432=CARTESIAN_POINT('Ctrl Pts',(10.417694044428,-40.,5.06310861338164));
#42433=CARTESIAN_POINT('Ctrl Pts',(10.5565955438655,-40.,4.82290230056891));
#42434=CARTESIAN_POINT('Ctrl Pts',(10.6868650567645,-40.,4.5778456180751));
#42435=CARTESIAN_POINT('Ctrl Pts',(10.8082364611378,-40.,4.32841151149382));
#42436=CARTESIAN_POINT('Ctrl Pts',(10.9290278826149,-40.,4.08016934560317));
#42437=CARTESIAN_POINT('Ctrl Pts',(11.0410063972023,-40.,3.82759096037244));
#42438=CARTESIAN_POINT('Ctrl Pts',(11.1438680903661,-40.,3.57111254742491));
#42439=CARTESIAN_POINT('Ctrl Pts',(11.2102577344974,-40.,3.4055746290881));
#42440=CARTESIAN_POINT('Ctrl Pts',(11.2728486827081,-40.,3.2384114695089));
#42441=CARTESIAN_POINT('Ctrl Pts',(11.3315488558307,-40.,3.06973522608137));
#42442=CARTESIAN_POINT('Ctrl Pts',(11.3969138737467,-40.,2.88190740399589));
#42443=CARTESIAN_POINT('Ctrl Pts',(11.4574546537082,-40.,2.69220336876743));
#42444=CARTESIAN_POINT('Ctrl Pts',(11.5131538719282,-40.,2.50080739873));
#42445=CARTESIAN_POINT('Ctrl Pts',(11.5219564527078,-40.,2.47055960457812));
#42446=CARTESIAN_POINT('Ctrl Pts',(11.5306367798565,-40.,2.44027394775998));
#42447=CARTESIAN_POINT('Ctrl Pts',(11.5391927173603,-40.,2.40995901899243));
#42448=CARTESIAN_POINT('Ctrl Pts',(11.6149930718682,-40.,2.14138735791641));
#42449=CARTESIAN_POINT('Ctrl Pts',(11.6810877877354,-40.,1.87033611873909));
#42450=CARTESIAN_POINT('Ctrl Pts',(11.7375427831218,-40.,1.59736118879834));
#42451=CARTESIAN_POINT('Ctrl Pts',(11.7945063358724,-40.,1.3219272486335));
#42452=CARTESIAN_POINT('Ctrl Pts',(11.8416558786766,-40.,1.04453424293325));
#42453=CARTESIAN_POINT('Ctrl Pts',(11.8790117308312,-40.,0.765729000453357));
#42454=CARTESIAN_POINT('Ctrl Pts',(11.9165716379187,-40.,0.485400794856042));
#42455=CARTESIAN_POINT('Ctrl Pts',(11.944230718393,-40.,0.203644274650995));
#42456=CARTESIAN_POINT('Ctrl Pts',(11.9619595695781,-40.,-0.0790002471504572));
#42457=CARTESIAN_POINT('Ctrl Pts',(11.9657577576826,-40.,-0.139553356276698));
#42458=CARTESIAN_POINT('Ctrl Pts',(11.9690999836388,-40.,-0.200147259763613));
#42459=CARTESIAN_POINT('Ctrl Pts',(11.9719856511623,-40.,-0.260776694674977));
#42460=CARTESIAN_POINT('Ctrl Pts',(11.9737712450156,-40.,-0.298292986980646));
#42461=CARTESIAN_POINT('Ctrl Pts',(11.9753819638708,-40.,-0.335822485014977));
#42462=CARTESIAN_POINT('Ctrl Pts',(11.9768172604587,-40.,-0.373350238049461));
#42463=CARTESIAN_POINT('Ctrl Pts',(11.9877545329118,-40.,-0.659319885686147));
#42464=CARTESIAN_POINT('Ctrl Pts',(11.9885197420998,-40.,-0.945390292321779));
#42465=CARTESIAN_POINT('Ctrl Pts',(11.9791433269757,-40.,-1.23099730766991));
#42466=CARTESIAN_POINT('Ctrl Pts',(11.9697517430852,-40.,-1.51706636592596));
#42467=CARTESIAN_POINT('Ctrl Pts',(11.9501858036918,-40.,-1.80267116614139));
#42468=CARTESIAN_POINT('Ctrl Pts',(11.9204255171557,-40.,-2.08725729207421));
#42469=CARTESIAN_POINT('Ctrl Pts',(11.8946825397073,-40.,-2.33342744279288));
#42470=CARTESIAN_POINT('Ctrl Pts',(11.8613109472889,-40.,-2.57883581882763));
#42471=CARTESIAN_POINT('Ctrl Pts',(11.8202663870092,-40.,-2.82312554759088));
#42472=CARTESIAN_POINT('Ctrl Pts',(11.8016841988292,-40.,-2.93372333885434));
#42473=CARTESIAN_POINT('Ctrl Pts',(11.7815289081037,-40.,-3.04409183784577));
#42474=CARTESIAN_POINT('Ctrl Pts',(11.7598151666302,-40.,-3.15420275595777));
#42475=CARTESIAN_POINT('Ctrl Pts',(-3.14788895504392,-20.,11.7604951161383));
#42476=CARTESIAN_POINT('Ctrl Pts',(-3.41583726409301,-20.,11.6689078365353));
#42477=CARTESIAN_POINT('Ctrl Pts',(-3.6800281171579,-20.,11.5679423474188));
#42478=CARTESIAN_POINT('Ctrl Pts',(-3.9400576560663,-20.,11.4579525320777));
#42479=CARTESIAN_POINT('Ctrl Pts',(-4.20217416505819,-20.,11.3470799498977));
#42480=CARTESIAN_POINT('Ctrl Pts',(-4.46006282884733,-20.,11.227037265788));
#42481=CARTESIAN_POINT('Ctrl Pts',(-4.71328870843099,-20.,11.0981380891977));
#42482=CARTESIAN_POINT('Ctrl Pts',(-4.96683786875418,-20.,10.9690743535142));
#42483=CARTESIAN_POINT('Ctrl Pts',(-5.2157128452745,-20.,10.8311311125707));
#42484=CARTESIAN_POINT('Ctrl Pts',(-5.45944793382123,-20.,10.6845799114082));
#42485=CARTESIAN_POINT('Ctrl Pts',(-5.70414316174853,-20.,10.5374514048592));
#42486=CARTESIAN_POINT('Ctrl Pts',(-5.9436584643848,-20.,10.381646622191));
#42487=CARTESIAN_POINT('Ctrl Pts',(-6.17748537864976,-20.,10.2174023572803));
#42488=CARTESIAN_POINT('Ctrl Pts',(-6.35285556434856,-20.,10.0942191585973));
#42489=CARTESIAN_POINT('Ctrl Pts',(-6.52502531464269,-20.,9.96628793637483));
#42490=CARTESIAN_POINT('Ctrl Pts',(-6.69376370895902,-20.,9.83369652465032));
#42491=CARTESIAN_POINT('Ctrl Pts',(-6.82031750469622,-20.,9.73425296585697));
#42492=CARTESIAN_POINT('Ctrl Pts',(-6.94494088192704,-20.,9.63218783302566));
#42493=CARTESIAN_POINT('Ctrl Pts',(-7.06753052957085,-20.,9.52753487822875));
#42494=CARTESIAN_POINT('Ctrl Pts',(-7.10083026081442,-20.,9.49910739405238));
#42495=CARTESIAN_POINT('Ctrl Pts',(-7.13398139806579,-20.,9.4704876398804));
#42496=CARTESIAN_POINT('Ctrl Pts',(-7.16697685341455,-20.,9.44168058852786));
#42497=CARTESIAN_POINT('Ctrl Pts',(-7.1942855680072,-20.,9.4178384097997));
#42498=CARTESIAN_POINT('Ctrl Pts',(-7.22148095877947,-20.,9.39387375783253));
#42499=CARTESIAN_POINT('Ctrl Pts',(-7.24855699713369,-20.,9.36979178770966));
#42500=CARTESIAN_POINT('Ctrl Pts',(-7.45693217509727,-20.,9.18445873623375));
#42501=CARTESIAN_POINT('Ctrl Pts',(-7.65835188614669,-20.,8.99208370432816));
#42502=CARTESIAN_POINT('Ctrl Pts',(-7.85239628226539,-20.,8.79294161273235));
#42503=CARTESIAN_POINT('Ctrl Pts',(-7.93912888539186,-20.,8.70393047743737));
#42504=CARTESIAN_POINT('Ctrl Pts',(-8.02438754698256,-20.,8.61356687371931));
#42505=CARTESIAN_POINT('Ctrl Pts',(-8.10813234606881,-20.,8.52187300942612));
#42506=CARTESIAN_POINT('Ctrl Pts',(-8.29599191369487,-20.,8.31618179172622));
#42507=CARTESIAN_POINT('Ctrl Pts',(-8.47623651864014,-20.,8.10379842051384));
#42508=CARTESIAN_POINT('Ctrl Pts',(-8.64862143631681,-20.,7.8852104092871));
#42509=CARTESIAN_POINT('Ctrl Pts',(-8.82101815484727,-20.,7.66660743430834));
#42510=CARTESIAN_POINT('Ctrl Pts',(-8.9855543755666,-20.,7.44179836760427));
#42511=CARTESIAN_POINT('Ctrl Pts',(-9.14193907461982,-20.,7.21124696766876));
#42512=CARTESIAN_POINT('Ctrl Pts',(-9.2972524856338,-20.,6.9822749227384));
#42513=CARTESIAN_POINT('Ctrl Pts',(-9.44452587993939,-20.,6.74763835305147));
#42514=CARTESIAN_POINT('Ctrl Pts',(-9.58342512212373,-20.,6.50777699481686));
#42515=CARTESIAN_POINT('Ctrl Pts',(-9.65196330375271,-20.,6.38942025594683));
#42516=CARTESIAN_POINT('Ctrl Pts',(-9.71846176210418,-20.,6.26979121078749));
#42517=CARTESIAN_POINT('Ctrl Pts',(-9.78287566835972,-20.,6.14894204251706));
#42518=CARTESIAN_POINT('Ctrl Pts',(-9.81320887096953,-20.,6.09203286685191));
#42519=CARTESIAN_POINT('Ctrl Pts',(-9.84307976388747,-20.,6.03485311689594));
#42520=CARTESIAN_POINT('Ctrl Pts',(-9.87248341770164,-20.,5.97740823116596));
#42521=CARTESIAN_POINT('Ctrl Pts',(-9.88901621100681,-20.,5.94510869355695));
#42522=CARTESIAN_POINT('Ctrl Pts',(-9.90540128490397,-20.,5.9127253338552));
#42523=CARTESIAN_POINT('Ctrl Pts',(-9.92163774063042,-20.,5.88025911881517));
#42524=CARTESIAN_POINT('Ctrl Pts',(-9.93566445788436,-20.,5.85221146935616));
#42525=CARTESIAN_POINT('Ctrl Pts',(-9.94957694946133,-20.,5.82410855096149));
#42526=CARTESIAN_POINT('Ctrl Pts',(-9.96337153280794,-20.,5.79595784393402));
#42527=CARTESIAN_POINT('Ctrl Pts',(-10.0085819469324,-20.,5.70369662149397));
#42528=CARTESIAN_POINT('Ctrl Pts',(-10.0525370764346,-20.,5.6108998857053));
#42529=CARTESIAN_POINT('Ctrl Pts',(-10.0952260546702,-20.,5.51759231250541));
#42530=CARTESIAN_POINT('Ctrl Pts',(-10.2089718864923,-20.,5.2689719901745));
#42531=CARTESIAN_POINT('Ctrl Pts',(-10.3137316499186,-20.,5.01672676215728));
#42532=CARTESIAN_POINT('Ctrl Pts',(-10.4092650117527,-20.,4.76131291979556));
#42533=CARTESIAN_POINT('Ctrl Pts',(-10.5040506852791,-20.,4.50789806438331));
#42534=CARTESIAN_POINT('Ctrl Pts',(-10.5897539783247,-20.,4.25136340977421));
#42535=CARTESIAN_POINT('Ctrl Pts',(-10.6660911528296,-20.,3.99214067649283));
#42536=CARTESIAN_POINT('Ctrl Pts',(-10.7164100464605,-20.,3.82126978393892));
#42537=CARTESIAN_POINT('Ctrl Pts',(-10.76265835388,-20.,3.64923065339804));
#42538=CARTESIAN_POINT('Ctrl Pts',(-10.8047424783443,-20.,3.47614542570932));
#42539=CARTESIAN_POINT('Ctrl Pts',(-10.8705314538897,-20.,3.20556596239269));
#42540=CARTESIAN_POINT('Ctrl Pts',(-10.9261465394823,-20.,2.93242944986049));
#42541=CARTESIAN_POINT('Ctrl Pts',(-10.971539533839,-20.,2.65731524077356));
#42542=CARTESIAN_POINT('Ctrl Pts',(-11.0169325281957,-20.,2.38220103168662));
#42543=CARTESIAN_POINT('Ctrl Pts',(-11.0521033806315,-20.,2.10510839212968));
#42544=CARTESIAN_POINT('Ctrl Pts',(-11.0769480123086,-20.,1.82662914162098));
#42545=CARTESIAN_POINT('Ctrl Pts',(-11.0805510773543,-20.,1.78624299838922));
#42546=CARTESIAN_POINT('Ctrl Pts',(-11.0839368669433,-20.,1.74582772459025));
#42547=CARTESIAN_POINT('Ctrl Pts',(-11.0871049669885,-20.,1.70538516141017));
#42548=CARTESIAN_POINT('Ctrl Pts',(-11.0904162776532,-20.,1.6631144348383));
#42549=CARTESIAN_POINT('Ctrl Pts',(-11.093490147485,-20.,1.62080741465348));
#42550=CARTESIAN_POINT('Ctrl Pts',(-11.0963238911948,-20.,1.57850150671815));
#42551=CARTESIAN_POINT('Ctrl Pts',(-11.1141911417012,-20.,1.31175534601939));
#42552=CARTESIAN_POINT('Ctrl Pts',(-11.1225356031101,-20.,1.04484600136718));
#42553=CARTESIAN_POINT('Ctrl Pts',(-11.1214040387022,-20.,0.778285111147121));
#42554=CARTESIAN_POINT('Ctrl Pts',(-11.1202704089919,-20.,0.511237700808428));
#42555=CARTESIAN_POINT('Ctrl Pts',(-11.1096260686144,-20.,0.244539371965727));
#42556=CARTESIAN_POINT('Ctrl Pts',(-11.0894661186613,-20.,-0.0212930845089499));
#42557=CARTESIAN_POINT('Ctrl Pts',(-11.0694226013899,-20.,-0.285590240256897));
#42558=CARTESIAN_POINT('Ctrl Pts',(-11.0399729544248,-20.,-0.549032107069646));
#42559=CARTESIAN_POINT('Ctrl Pts',(-11.0010625247024,-20.,-0.811099100987041));
#42560=CARTESIAN_POINT('Ctrl Pts',(-10.962784322418,-20.,-1.06890795781023));
#42561=CARTESIAN_POINT('Ctrl Pts',(-10.9153500989546,-20.,-1.32538677921543));
#42562=CARTESIAN_POINT('Ctrl Pts',(-10.8586617972334,-20.,-1.58002123156791));
#42563=CARTESIAN_POINT('Ctrl Pts',(-10.8242835539937,-20.,-1.73444260025203));
#42564=CARTESIAN_POINT('Ctrl Pts',(-10.7865010252999,-20.,-1.88818524302589));
#42565=CARTESIAN_POINT('Ctrl Pts',(-10.7452842897659,-20.,-2.04112961510651));
#42566=CARTESIAN_POINT('Ctrl Pts',(-10.6983394263361,-20.,-2.21532955031828));
#42567=CARTESIAN_POINT('Ctrl Pts',(-10.6469394936606,-20.,-2.38849410088828));
#42568=CARTESIAN_POINT('Ctrl Pts',(-10.5911391151801,-20.,-2.5604596881072));
#42569=CARTESIAN_POINT('Ctrl Pts',(-10.5808112700642,-20.,-2.59228803763508));
#42570=CARTESIAN_POINT('Ctrl Pts',(-10.5703323195386,-20.,-2.6240761705273));
#42571=CARTESIAN_POINT('Ctrl Pts',(-10.5597080024052,-20.,-2.65580723494851));
#42572=CARTESIAN_POINT('Ctrl Pts',(-10.4761217376019,-20.,-2.90544974089913));
#42573=CARTESIAN_POINT('Ctrl Pts',(-10.3834680471006,-20.,-3.1517916819884));
#42574=CARTESIAN_POINT('Ctrl Pts',(-10.2820203829828,-20.,-3.39437485165505));
#42575=CARTESIAN_POINT('Ctrl Pts',(-10.1805768302642,-20.,-3.63694819008265));
#42576=CARTESIAN_POINT('Ctrl Pts',(-10.070339637341,-20.,-3.87576361218799));
#42577=CARTESIAN_POINT('Ctrl Pts',(-9.9515383732788,-20.,-4.1103350805885));
#42578=CARTESIAN_POINT('Ctrl Pts',(-9.8329461967683,-20.,-4.3444937084824));
#42579=CARTESIAN_POINT('Ctrl Pts',(-9.70581969060581,-20.,-4.5744238409605));
#42580=CARTESIAN_POINT('Ctrl Pts',(-9.57034919815825,-20.,-4.79960611605748));
#42581=CARTESIAN_POINT('Ctrl Pts',(-9.54674783670939,-20.,-4.83883686048325));
#42582=CARTESIAN_POINT('Ctrl Pts',(-9.52289211519482,-20.,-4.87792504279439));
#42583=CARTESIAN_POINT('Ctrl Pts',(-9.49878621049929,-20.,-4.9168625054116));
#42584=CARTESIAN_POINT('Ctrl Pts',(-9.47147256286588,-20.,-4.96098132804441));
#42585=CARTESIAN_POINT('Ctrl Pts',(-9.44384413272872,-20.,-5.00489628904724));
#42586=CARTESIAN_POINT('Ctrl Pts',(-9.41590688798062,-20.,-5.04859740776055));
#42587=CARTESIAN_POINT('Ctrl Pts',(-9.27645734814993,-20.,-5.26673276611845));
#42588=CARTESIAN_POINT('Ctrl Pts',(-9.12928197945513,-20.,-5.47959888543939));
#42589=CARTESIAN_POINT('Ctrl Pts',(-8.97460596288743,-20.,-5.68672989182249));
#42590=CARTESIAN_POINT('Ctrl Pts',(-8.82197250195883,-20.,-5.89112565447157));
#42591=CARTESIAN_POINT('Ctrl Pts',(-8.66203475773642,-20.,-6.0899371852121));
#42592=CARTESIAN_POINT('Ctrl Pts',(-8.49497512476503,-20.,-6.28267972759005));
#42593=CARTESIAN_POINT('Ctrl Pts',(-8.37973300463925,-20.,-6.4156385927988));
#42594=CARTESIAN_POINT('Ctrl Pts',(-8.26110115916421,-20.,-6.54570870297757));
#42595=CARTESIAN_POINT('Ctrl Pts',(-8.13913138220323,-20.,-6.6727188759329));
#42596=CARTESIAN_POINT('Ctrl Pts',(-8.07193084909504,-20.,-6.74269646829574));
#42597=CARTESIAN_POINT('Ctrl Pts',(-8.0037169417772,-20.,-6.81174500263592));
#42598=CARTESIAN_POINT('Ctrl Pts',(-7.93451184210526,-20.,-6.87984615149801));
#42599=CARTESIAN_POINT('Origin',(0.,-40.,-2.22044604925031E-15));
#42600=CARTESIAN_POINT('',(9.46171656752341,-40.,16.3881738217667));
#42601=CARTESIAN_POINT('',(-9.46171656752339,-40.,16.3881738217667));
#42602=CARTESIAN_POINT('',(9.46171656752341,-40.,16.3881738217667));
#42603=CARTESIAN_POINT('',(-18.9234331350468,-40.,4.44089209850063E-15));
#42604=CARTESIAN_POINT('',(-9.46171656752339,-40.,16.3881738217667));
#42605=CARTESIAN_POINT('',(-9.4617165675234,-40.,-16.3881738217667));
#42606=CARTESIAN_POINT('',(-18.9234331350468,-40.,4.44089209850063E-15));
#42607=CARTESIAN_POINT('',(9.46171656752339,-40.,-16.3881738217667));
#42608=CARTESIAN_POINT('',(-9.4617165675234,-40.,-16.3881738217667));
#42609=CARTESIAN_POINT('',(18.9234331350468,-40.,-1.22124532708767E-14));
#42610=CARTESIAN_POINT('',(9.46171656752339,-40.,-16.3881738217667));
#42611=CARTESIAN_POINT('',(18.9234331350468,-40.,-1.22124532708767E-14));
#42612=CARTESIAN_POINT('Origin',(18.9234331350468,-20.,-1.22124532708767E-14));
#42613=CARTESIAN_POINT('',(18.9234331350468,-20.,-1.22124532708767E-14));
#42614=CARTESIAN_POINT('',(9.46171656752341,-20.,16.3881738217667));
#42615=CARTESIAN_POINT('',(18.9234331350468,-20.,-1.22124532708767E-14));
#42616=CARTESIAN_POINT('',(9.46171656752341,-20.,16.3881738217667));
#42617=CARTESIAN_POINT('',(18.9234331350468,-20.,-1.22124532708767E-14));
#42618=CARTESIAN_POINT('Origin',(9.46171656752339,-20.,-16.3881738217667));
#42619=CARTESIAN_POINT('',(9.46171656752339,-20.,-16.3881738217667));
#42620=CARTESIAN_POINT('',(9.46171656752339,-20.,-16.3881738217667));
#42621=CARTESIAN_POINT('',(9.46171656752339,-20.,-16.3881738217667));
#42622=CARTESIAN_POINT('Origin',(-9.4617165675234,-20.,-16.3881738217667));
#42623=CARTESIAN_POINT('',(-9.4617165675234,-20.,-16.3881738217667));
#42624=CARTESIAN_POINT('',(-9.4617165675234,-20.,-16.3881738217667));
#42625=CARTESIAN_POINT('',(-9.4617165675234,-20.,-16.3881738217667));
#42626=CARTESIAN_POINT('Origin',(-18.9234331350468,-20.,4.44089209850063E-15));
#42627=CARTESIAN_POINT('',(-18.9234331350468,-20.,4.44089209850063E-15));
#42628=CARTESIAN_POINT('',(-18.9234331350468,-20.,4.44089209850063E-15));
#42629=CARTESIAN_POINT('',(-18.9234331350468,-20.,4.44089209850063E-15));
#42630=CARTESIAN_POINT('Origin',(-9.46171656752339,-20.,16.3881738217667));
#42631=CARTESIAN_POINT('',(-9.46171656752339,-20.,16.3881738217667));
#42632=CARTESIAN_POINT('',(-9.46171656752339,-20.,16.3881738217667));
#42633=CARTESIAN_POINT('',(-9.46171656752339,-20.,16.3881738217667));
#42634=CARTESIAN_POINT('Origin',(9.46171656752341,-20.,16.3881738217667));
#42635=CARTESIAN_POINT('',(9.46171656752341,-20.,16.3881738217667));
#42636=CARTESIAN_POINT('Origin',(0.,-20.,-2.22044604925031E-15));
#42655=UNCERTAINTY_MEASURE_WITH_UNIT(LENGTH_MEASURE(0.01),#42668,
'DISTANCE_ACCURACY_VALUE',
'Maximum model space distance between geometric entities at asserted c
onnectivities');
#42656=UNCERTAINTY_MEASURE_WITH_UNIT(LENGTH_MEASURE(0.01),#42668,
'DISTANCE_ACCURACY_VALUE',
'Maximum model space distance between geometric entities at asserted c
onnectivities');
#42666=(
GEOMETRIC_REPRESENTATION_CONTEXT(3)
GLOBAL_UNCERTAINTY_ASSIGNED_CONTEXT((#42655))
GLOBAL_UNIT_ASSIGNED_CONTEXT((#42668,#42670,#42671))
REPRESENTATION_CONTEXT('','3D')
);
#42667=(
GEOMETRIC_REPRESENTATION_CONTEXT(3)
GLOBAL_UNCERTAINTY_ASSIGNED_CONTEXT((#42656))
GLOBAL_UNIT_ASSIGNED_CONTEXT((#42668,#42670,#42671))
REPRESENTATION_CONTEXT('','3D')
);
#42668=(
LENGTH_UNIT()
NAMED_UNIT(*)
SI_UNIT(.MILLI.,.METRE.)
);
#42670=(
NAMED_UNIT(*)
PLANE_ANGLE_UNIT()
SI_UNIT($,.RADIAN.)
);
#42671=(
NAMED_UNIT(*)
SI_UNIT($,.STERADIAN.)
SOLID_ANGLE_UNIT()
);
#42681=SHAPE_DEFINITION_REPRESENTATION(#42691,#42710);
#42691=PRODUCT_DEFINITION_SHAPE('',$,#42721);
#42710=SHAPE_REPRESENTATION('',(#4430),#42666);
#42711=PRODUCT_DEFINITION_CONTEXT('part definition',#42743,'design');
#42721=PRODUCT_DEFINITION('Adapter_01','Adapter_01',#42731,#42711);
#42731=PRODUCT_DEFINITION_FORMATION('',$,#42754);
#42743=APPLICATION_CONTEXT(
'Core Data for Automotive Mechanical Design Process');
#42744=PRODUCT_CONTEXT('part definition',#42743,'mechanical');
#42754=PRODUCT('Adapter_01','Adapter_01',$,(#42744));
#42756=PRESENTATION_STYLE_ASSIGNMENT((#42758));
#42758=SURFACE_STYLE_USAGE(.BOTH.,#42760);
#42760=SURFACE_SIDE_STYLE('',(#42762));
#42762=SURFACE_STYLE_FILL_AREA(#42764);
#42764=FILL_AREA_STYLE('Opaque(160,160,160)',(#42766));
#42766=FILL_AREA_STYLE_COLOUR('Opaque(160,160,160)',#42768);
#42768=COLOUR_RGB('Opaque(160,160,160)', 0.09019608, 0.27058824, 0.51372549);
ENDSEC;
END-ISO-10303-21;
